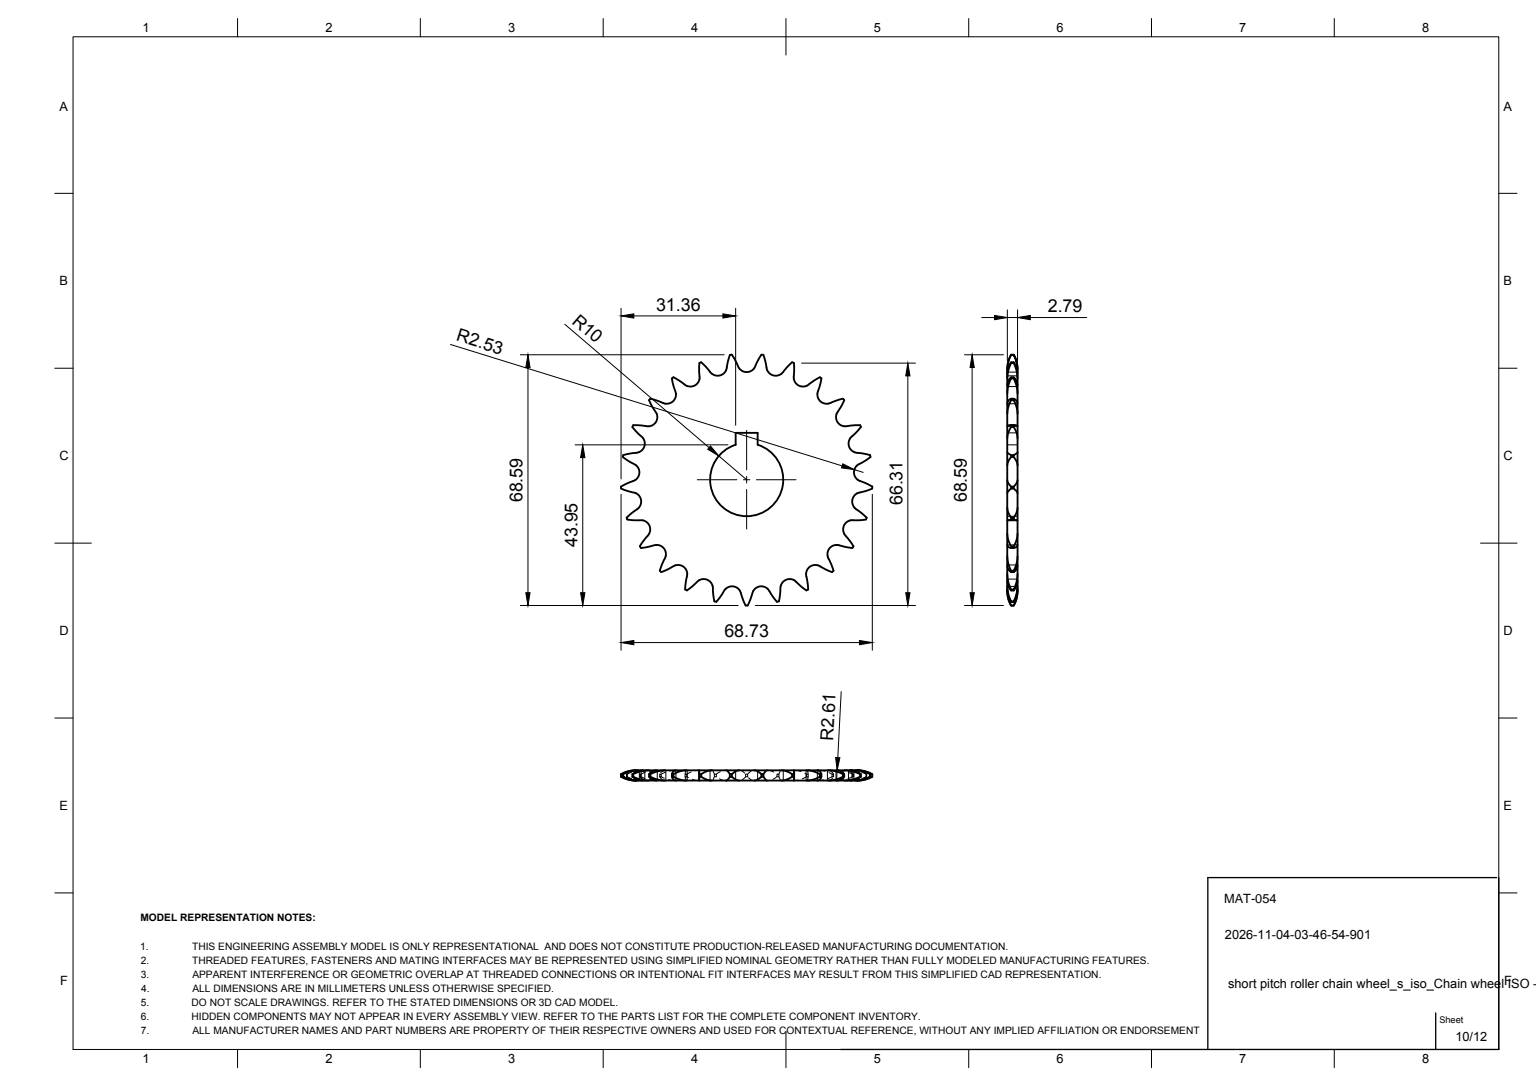
ISO-10303-21;
HEADER;
FILE_DESCRIPTION (('STEP AP214'),
    '1' );
FILE_NAME ('short pitch roller chain wheel_s_iso_Chain wheel ISO - 25Z 05B-1 --25SA20.0S1.step',
    '2026-10-21T17:50:41',
    ( '' ),
    ( '' ),
    'SwSTEP 2.0',
    'SolidWorks 2026',
    '' );
FILE_SCHEMA (( 'AUTOMOTIVE_DESIGN' ));
ENDSEC;

DATA;
#9=CARTESIAN_POINT ( 'NONE',  ( 0.000000000000000000, -17.83604598421681331, 24.70480026434162113 ) ) ;
#11=CARTESIAN_POINT ( 'NONE',  ( 2.789999999999999147, -7.666252171205286459, -29.49034198003814566 ) ) ;
#12=ADVANCED_FACE ( 'NONE', ( #16842 ), #19853, .T. ) ;
#15=ORIENTED_EDGE ( 'NONE', *, *, #1082, .T. ) ;
#18=DIRECTION ( 'NONE',  ( -1.000000000000000000, -0.000000000000000000, -0.000000000000000000 ) ) ;
#20=EDGE_LOOP ( 'NONE', ( #54, #27423, #18321, #7945 ) ) ;
#27=EDGE_LOOP ( 'NONE', ( #3921, #9561, #6087, #4128, #28214, #30495, #16586, #17626 ) ) ;
#41=DIRECTION ( 'NONE',  ( -1.000000000000000000, -0.000000000000000000, -0.000000000000000000 ) ) ;
#48=CARTESIAN_POINT ( 'NONE',  ( 8.000000000000000000, 0.000000000000000000, 0.000000000000000000 ) ) ;
#50=DIRECTION ( 'NONE',  ( -1.000000000000000000, -0.000000000000000000, -0.000000000000000000 ) ) ;
#53=B_SPLINE_CURVE_WITH_KNOTS ( 'NONE', 3,
 ( #11296, #13610, #21443, #2909 ),
 .UNSPECIFIED., .F., .F.,
 ( 4, 4 ),
 ( 1.980634265047841514E-07, 0.0006879337600918932361 ),
 .UNSPECIFIED. ) ;
#54=ORIENTED_EDGE ( 'NONE', *, *, #21337, .T. ) ;
#56=CARTESIAN_POINT ( 'NONE',  ( 2.789999999999999147, -23.41952779159776199, 19.49300927180536291 ) ) ;
#64=AXIS2_PLACEMENT_3D ( 'NONE', #13573, #18917, #21744 ) ;
#71=DIRECTION ( 'NONE',  ( 0.000000000000000000, -6.870191984066554061E-16, -1.000000000000000000 ) ) ;
#72=EDGE_LOOP ( 'NONE', ( #10606, #16036, #12165, #7623, #9118, #25813 ) ) ;
#78=ORIENTED_EDGE ( 'NONE', *, *, #19900, .T. ) ;
#82=ORIENTED_EDGE ( 'NONE', *, *, #22501, .F. ) ;
#89=FACE_OUTER_BOUND ( 'NONE', #8391, .T. ) ;
#102=AXIS2_PLACEMENT_3D ( 'NONE', #15826, #31812, #4404 ) ;
#107=CARTESIAN_POINT ( 'NONE',  ( 0.000000000000000000, -29.91351748324107973, 5.799410679710550021 ) ) ;
#112=ADVANCED_FACE ( 'NONE', ( #7166 ), #34411, .T. ) ;
#113=DIRECTION ( 'NONE',  ( 0.000000000000000000, 1.717547996016640980E-15, -1.000000000000000000 ) ) ;
#115=CARTESIAN_POINT ( 'NONE',  ( 1.749999999999999778, -10.89151784028265624, -32.64600270996228204 ) ) ;
#117=ORIENTED_EDGE ( 'NONE', *, *, #2620, .T. ) ;
#131=CARTESIAN_POINT ( 'NONE',  ( 1.039999999999999591, -18.21166265554809627, 29.20140402659733425 ) ) ;
#147=B_SPLINE_CURVE_WITH_KNOTS ( 'NONE', 3,
 ( #10015, #12703, #20870, #26557, #32247, #23363 ),
 .UNSPECIFIED., .F., .F.,
 ( 4, 2, 4 ),
 ( 2.446897702420577325E-07, 0.001873443032870420388, 0.003746641375970598611 ),
 .UNSPECIFIED. ) ;
#152=B_SPLINE_CURVE_WITH_KNOTS ( 'NONE', 3,
 ( #1584, #18327, #31299, #33977, #2108, #6909 ),
 .UNSPECIFIED., .F., .F.,
 ( 4, 2, 4 ),
 ( 4.404817104455272006E-07, 0.001874269680285309877, 0.003748098878860173927 ),
 .UNSPECIFIED. ) ;
#154=AXIS2_PLACEMENT_3D ( 'NONE', #33975, #1065, #20629 ) ;
#159=ORIENTED_EDGE ( 'NONE', *, *, #4581, .F. ) ;
#163=EDGE_CURVE ( 'NONE', #29138, #16548, #8258, .T. ) ;
#164=DIRECTION ( 'NONE',  ( -1.000000000000000000, -0.000000000000000000, -0.000000000000000000 ) ) ;
#176=DIRECTION ( 'NONE',  ( 0.000000000000000000, 0.000000000000000000, 1.000000000000000000 ) ) ;
#183=CARTESIAN_POINT ( 'NONE',  ( 1.749999999999999778, 32.09669216789253454, -12.41728656686340138 ) ) ;
#184=DIRECTION ( 'NONE',  ( 0.000000000000000000, 0.000000000000000000, 1.000000000000000000 ) ) ;
#188=TOROIDAL_SURFACE ( 'NONE', #34853, 30.47050528711512030, 8.000000000000000000 ) ;
#190=LINE ( 'NONE', #16406, #20541 ) ;
#191=CARTESIAN_POINT ( 'NONE',  ( 2.789999999999999147, -1.291199951812987523, -30.41225463960053332 ) ) ;
#205=TOROIDAL_SURFACE ( 'NONE', #2485, 30.47050528711512030, 8.000000000000000000 ) ;
#206=ORIENTED_EDGE ( 'NONE', *, *, #33017, .T. ) ;
#207=ORIENTED_EDGE ( 'NONE', *, *, #14796, .T. ) ;
#218=CARTESIAN_POINT ( 'NONE',  ( 1.749999999999999778, -33.26546734453825849, 8.820166447041632551 ) ) ;
#220=CARTESIAN_POINT ( 'NONE',  ( 0.5248942730704680981, -11.05013152551600442, -31.49770363594219091 ) ) ;
#227=CARTESIAN_POINT ( 'NONE',  ( -8.297462993384987146E-14, 27.83741677616693266, 12.85620214406761086 ) ) ;
#245=VERTEX_POINT ( 'NONE', #5376 ) ;
#256=VECTOR ( 'NONE', #18006, 1000.000000000000000 ) ;
#258=CARTESIAN_POINT ( 'NONE',  ( 2.789999999999999147, -25.83993731729808729, 18.77381338200959604 ) ) ;
#263=AXIS2_PLACEMENT_3D ( 'NONE', #22124, #50, #11096 ) ;
#267=CARTESIAN_POINT ( 'NONE',  ( 0.000000000000000000, -7.666252171205264254, -29.49034198003815632 ) ) ;
#272=ORIENTED_EDGE ( 'NONE', *, *, #3278, .F. ) ;
#278=ADVANCED_FACE ( 'NONE', ( #16441 ), #5428, .T. ) ;
#289=ORIENTED_EDGE ( 'NONE', *, *, #26141, .T. ) ;
#292=VERTEX_POINT ( 'NONE', #13238 ) ;
#293=ORIENTED_EDGE ( 'NONE', *, *, #23924, .F. ) ;
#294=CARTESIAN_POINT ( 'NONE',  ( -10.00000000000000000, 0.000000000000000000, 0.000000000000000000 ) ) ;
#301=CARTESIAN_POINT ( 'NONE',  ( 2.033589663487044952, 13.95893286369055097, -30.90974742850055179 ) ) ;
#312=CARTESIAN_POINT ( 'NONE',  ( 2.789999999999999147, 7.350529080603967813, -30.20932655202929595 ) ) ;
#320=CARTESIAN_POINT ( 'NONE',  ( 1.749999999999999778, 0.000000000000000000, 0.000000000000000000 ) ) ;
#326=ORIENTED_EDGE ( 'NONE', *, *, #11265, .T. ) ;
#328=CARTESIAN_POINT ( 'NONE',  ( 2.789999999999999147, 0.000000000000000000, 0.000000000000000000 ) ) ;
#343=ORIENTED_EDGE ( 'NONE', *, *, #19695, .F. ) ;
#349=CARTESIAN_POINT ( 'NONE',  ( 0.000000000000000000, -30.41598411195408502, -1.821977758773957179 ) ) ;
#364=VECTOR ( 'NONE', #34672, 1000.000000000000000 ) ;
#391=CARTESIAN_POINT ( 'NONE',  ( 2.261199744108339349, -18.53787122671715082, -27.77096539590149504 ) ) ;
#400=ORIENTED_EDGE ( 'NONE', *, *, #18488, .T. ) ;
#401=DIRECTION ( 'NONE',  ( 0.000000000000000000, -4.122115190439938353E-15, -1.000000000000000000 ) ) ;
#403=DIRECTION ( 'NONE',  ( 0.000000000000000000, 0.000000000000000000, 1.000000000000000000 ) ) ;
#405=CARTESIAN_POINT ( 'NONE',  ( 2.789999999999999147, -2.530647759431309929, -30.33427519320597199 ) ) ;
#408=FACE_OUTER_BOUND ( 'NONE', #18168, .T. ) ;
#416=ORIENTED_EDGE ( 'NONE', *, *, #6218, .F. ) ;
#422=DIRECTION ( 'NONE',  ( -1.000000000000000000, -0.000000000000000000, -0.000000000000000000 ) ) ;
#432=ORIENTED_EDGE ( 'NONE', *, *, #20397, .F. ) ;
#447=CARTESIAN_POINT ( 'NONE',  ( 0.006892415499590480790, 4.187058600949983500, -30.58452291340886831 ) ) ;
#448=CARTESIAN_POINT ( 'NONE',  ( 2.719010669804482916, -30.32061017160040350, -9.230676164042293408 ) ) ;
#453=ORIENTED_EDGE ( 'NONE', *, *, #7812, .T. ) ;
#455=CIRCLE ( 'NONE', #12411, 2.524999999999999467 ) ;
#462=EDGE_LOOP ( 'NONE', ( #2821, #4541, #31445, #15602, #5501, #28046 ) ) ;
#471=CARTESIAN_POINT ( 'NONE',  ( 2.783107615394383672, -17.88431215799149143, 25.16139613958896604 ) ) ;
#483=CARTESIAN_POINT ( 'NONE',  ( 0.7564103440795023614, 14.91861104533797899, -30.45815716957487496 ) ) ;
#485=DIRECTION ( 'NONE',  ( -1.000000000000000000, 0.000000000000000000, -0.000000000000000000 ) ) ;
#487=ORIENTED_EDGE ( 'NONE', *, *, #9637, .F. ) ;
#491=CIRCLE ( 'NONE', #22653, 2.524999999999999467 ) ;
#492=DIRECTION ( 'NONE',  ( -1.000000000000000000, -0.000000000000000000, -0.000000000000000000 ) ) ;
#500=TOROIDAL_SURFACE ( 'NONE', #9599, 30.47050528711512030, 8.000000000000000000 ) ;
#507=CARTESIAN_POINT ( 'NONE',  ( 0.5248942543850775300, -33.37077467988373769, 0.7759739055973007282 ) ) ;
#509=VERTEX_POINT ( 'NONE', #1793 ) ;
#513=CARTESIAN_POINT ( 'NONE',  ( 2.719010673315533477, 14.74869129583236216, -28.05389252521634802 ) ) ;
#517=ORIENTED_EDGE ( 'NONE', *, *, #32290, .F. ) ;
#527=VERTEX_POINT ( 'NONE', #12669 ) ;
#528=LINE ( 'NONE', #11379, #25963 ) ;
#536=DIRECTION ( 'NONE',  ( 1.000000000000000000, -0.000000000000000000, -0.000000000000000000 ) ) ;
#537=ORIENTED_EDGE ( 'NONE', *, *, #19901, .F. ) ;
#543=LINE ( 'NONE', #35085, #19991 ) ;
#550=DIRECTION ( 'NONE',  ( -1.000000000000000000, 0.000000000000000000, 0.000000000000000000 ) ) ;
#559=EDGE_CURVE ( 'NONE', #10218, #5077, #21246, .T. ) ;
#570=CARTESIAN_POINT ( 'NONE',  ( 0.000000000000000000, -20.35927063852824048, 24.61013060777164796 ) ) ;
#583=DIRECTION ( 'NONE',  ( -1.000000000000000000, -0.000000000000000000, -0.000000000000000000 ) ) ;
#589=CARTESIAN_POINT ( 'NONE',  ( 2.789999999999999591, -3.625355760179855835, 30.44651458975030067 ) ) ;
#595=CARTESIAN_POINT ( 'NONE',  ( 0.000000000000000000, -25.77598557799239742, -16.24962337825829195 ) ) ;
#597=ORIENTED_EDGE ( 'NONE', *, *, #21069, .F. ) ;
#602=ADVANCED_FACE ( 'NONE', ( #4451 ), #23172, .T. ) ;
#605=CARTESIAN_POINT ( 'NONE',  ( 2.261199747851626807, 5.497007441955480189, -32.93420861807575051 ) ) ;
#612=CARTESIAN_POINT ( 'NONE',  ( 1.040000000000003810, -2.430610048905784915, -34.32897884578301984 ) ) ;
#615=CARTESIAN_POINT ( 'NONE',  ( 1.040000000000000258, 28.00026196654270905, 20.00929742917132614 ) ) ;
#617=CARTESIAN_POINT ( 'NONE',  ( 0.02407890056655825201, -23.70329957282570632, -20.11932597908854703 ) ) ;
#622=( GEOMETRIC_REPRESENTATION_CONTEXT ( 3 ) GLOBAL_UNCERTAINTY_ASSIGNED_CONTEXT ( ( #6076 ) ) GLOBAL_UNIT_ASSIGNED_CONTEXT ( ( #14562, #33576, #1191 ) ) REPRESENTATION_CONTEXT ( 'NONE', 'WORKASPACE' ) );
#625=DIRECTION ( 'NONE',  ( -1.000000000000000000, -0.000000000000000000, -0.000000000000000000 ) ) ;
#628=CYLINDRICAL_SURFACE ( 'NONE', #33668, 34.41491905851385269 ) ;
#637=DIRECTION ( 'NONE',  ( -1.000000000000000000, -0.000000000000000000, -0.000000000000000000 ) ) ;
#638=CARTESIAN_POINT ( 'NONE',  ( 2.789999999999999147, -21.75986515490462736, -21.28569233123117144 ) ) ;
#642=FACE_OUTER_BOUND ( 'NONE', #3782, .T. ) ;
#644=AXIS2_PLACEMENT_3D ( 'NONE', #32551, #30604, #176 ) ;
#645=CARTESIAN_POINT ( 'NONE',  ( -4.087654984470516816E-16, 27.73515059361837842, -12.87176213890998433 ) ) ;
#655=LINE ( 'NONE', #13651, #10552 ) ;
#671=AXIS2_PLACEMENT_3D ( 'NONE', #19191, #13656, #30199 ) ;
#674=CARTESIAN_POINT ( 'NONE',  ( 1.749999999999999778, 14.89726405156217126, 31.02351007835983054 ) ) ;
#681=EDGE_CURVE ( 'NONE', #1567, #23446, #30476, .T. ) ;
#684=DIRECTION ( 'NONE',  ( -1.000000000000000000, -0.000000000000000000, -0.000000000000000000 ) ) ;
#686=CARTESIAN_POINT ( 'NONE',  ( 0.02407890056655695096, -23.70329957282599764, 20.11932597908820242 ) ) ;
#689=LINE ( 'NONE', #22397, #22097 ) ;
#693=VERTEX_POINT ( 'NONE', #5676 ) ;
#698=CARTESIAN_POINT ( 'NONE',  ( 2.765921099433441999, -23.70329957282570632, -20.11932597908854703 ) ) ;
#701=VERTEX_POINT ( 'NONE', #5505 ) ;
#706=CARTESIAN_POINT ( 'NONE',  ( 0.02407890056655868569, 24.20451283648829133, 19.51346322004938827 ) ) ;
#713=FACE_OUTER_BOUND ( 'NONE', #31703, .T. ) ;
#719=EDGE_CURVE ( 'NONE', #25735, #29292, #10014, .T. ) ;
#723=VECTOR ( 'NONE', #4056, 1000.000000000000000 ) ;
#758=ORIENTED_EDGE ( 'NONE', *, *, #30163, .F. ) ;
#762=EDGE_CURVE ( 'NONE', #30403, #3499, #15137, .T. ) ;
#765=ORIENTED_EDGE ( 'NONE', *, *, #6752, .T. ) ;
#767=AXIS2_PLACEMENT_3D ( 'NONE', #17195, #9516, #17375 ) ;
#784=ORIENTED_EDGE ( 'NONE', *, *, #22789, .T. ) ;
#795=AXIS2_PLACEMENT_3D ( 'NONE', #25885, #23221, #30872 ) ;
#797=VERTEX_POINT ( 'NONE', #7654 ) ;
#798=DIRECTION ( 'NONE',  ( 0.000000000000000000, 0.000000000000000000, 1.000000000000000000 ) ) ;
#812=ORIENTED_EDGE ( 'NONE', *, *, #27179, .F. ) ;
#814=B_SPLINE_CURVE_WITH_KNOTS ( 'NONE', 3,
 ( #14475, #31011, #28163, #940, #14997, #1459 ),
 .UNSPECIFIED., .F., .F.,
 ( 4, 2, 4 ),
 ( 2.343813143889068798E-07, 0.001873432713173589807, 0.003746631045032783325 ),
 .UNSPECIFIED. ) ;
#816=CIRCLE ( 'NONE', #30389, 30.47050528711512030 ) ;
#818=CARTESIAN_POINT ( 'NONE',  ( 0.000000000000000000, 0.000000000000000000, 0.000000000000000000 ) ) ;
#822=CARTESIAN_POINT ( 'NONE',  ( 0.07098932849787087385, 31.23843357299762857, -5.357709411917221054 ) ) ;
#824=ORIENTED_EDGE ( 'NONE', *, *, #23128, .F. ) ;
#830=DIRECTION ( 'NONE',  ( 0.000000000000000000, 0.000000000000000000, 1.000000000000000000 ) ) ;
#831=CARTESIAN_POINT ( 'NONE',  ( 0.000000000000000000, -5.984944020946091570, 31.37417528048439763 ) ) ;
#833=CARTESIAN_POINT ( 'NONE',  ( 1.394999999999999574, 6.714005886385425725, -33.75364837705166110 ) ) ;
#839=AXIS2_PLACEMENT_3D ( 'NONE', #13257, #7899, #20906 ) ;
#840=B_SPLINE_CURVE_WITH_KNOTS ( 'NONE', 3,
 ( #9936, #25292, #8926, #10109, #6597, #26129 ),
 .UNSPECIFIED., .F., .F.,
 ( 4, 2, 4 ),
 ( 4.404817133574835894E-07, 0.001874269703891905288, 0.003748098926070445643 ),
 .UNSPECIFIED. ) ;
#845=AXIS2_PLACEMENT_3D ( 'NONE', #22762, #9054, #27387 ) ;
#850=AXIS2_PLACEMENT_3D ( 'NONE', #14253, #6390, #19596 ) ;
#853=LINE ( 'NONE', #6703, #25713 ) ;
#856=ORIENTED_EDGE ( 'NONE', *, *, #12997, .T. ) ;
#876=ORIENTED_EDGE ( 'NONE', *, *, #5437, .T. ) ;
#886=ORIENTED_EDGE ( 'NONE', *, *, #32162, .T. ) ;
#908=CARTESIAN_POINT ( 'NONE',  ( 8.000000000000000000, 0.000000000000000000, 0.000000000000000000 ) ) ;
#915=DIRECTION ( 'NONE',  ( -1.000000000000000000, -0.000000000000000000, -0.000000000000000000 ) ) ;
#916=VERTEX_POINT ( 'NONE', #17758 ) ;
#919=AXIS2_PLACEMENT_3D ( 'NONE', #30994, #17497, #28147 ) ;
#925=CARTESIAN_POINT ( 'NONE',  ( 0.07094833174329351344, -22.12275578582332258, -22.69570394412150094 ) ) ;
#926=EDGE_CURVE ( 'NONE', #18645, #8559, #4534, .T. ) ;
#930=DIRECTION ( 'NONE',  ( -1.000000000000000000, -0.000000000000000000, 0.000000000000000000 ) ) ;
#933=CARTESIAN_POINT ( 'NONE',  ( 0.000000000000000000, 0.000000000000000000, 0.000000000000000000 ) ) ;
#938=CARTESIAN_POINT ( 'NONE',  ( 0.07098930208213954929, -22.12324074713423983, 22.69596835361121379 ) ) ;
#939=VERTEX_POINT ( 'NONE', #24113 ) ;
#940=CARTESIAN_POINT ( 'NONE',  ( 2.265105836449367249, -9.574141296992072725, -31.97728166840280295 ) ) ;
#947=EDGE_LOOP ( 'NONE', ( #30573, #9309, #21201, #23371 ) ) ;
#949=VERTEX_POINT ( 'NONE', #26096 ) ;
#956=CARTESIAN_POINT ( 'NONE',  ( 1.749999999999999778, 0.000000000000000000, 0.000000000000000000 ) ) ;
#965=DIRECTION ( 'NONE',  ( -1.000000000000000000, -0.000000000000000000, 0.000000000000000000 ) ) ;
#968=EDGE_CURVE ( 'NONE', #34921, #949, #21287, .T. ) ;
#992=ORIENTED_EDGE ( 'NONE', *, *, #23128, .T. ) ;
#1002=ORIENTED_EDGE ( 'NONE', *, *, #10125, .T. ) ;
#1008=CARTESIAN_POINT ( 'NONE',  ( 1.040000000000000924, -18.66807150955393624, -28.91175816027522316 ) ) ;
#1011=EDGE_CURVE ( 'NONE', #29748, #30400, #2067, .T. ) ;
#1013=DIRECTION ( 'NONE',  ( -1.000000000000000000, 0.000000000000000000, 0.000000000000000000 ) ) ;
#1023=ORIENTED_EDGE ( 'NONE', *, *, #17027, .T. ) ;
#1026=CIRCLE ( 'NONE', #29448, 2.525000000000000799 ) ;
#1033=CYLINDRICAL_SURFACE ( 'NONE', #4520, 16.19999999999999929 ) ;
#1048=B_SPLINE_CURVE_WITH_KNOTS ( 'NONE', 3,
 ( #12793, #34310, #605, #32333, #16164, #22322 ),
 .UNSPECIFIED., .F., .F.,
 ( 4, 2, 4 ),
 ( 4.404817060652725496E-07, 0.001874269649560036423, 0.003748098817414007630 ),
 .UNSPECIFIED. ) ;
#1049=CARTESIAN_POINT ( 'NONE',  ( 1.040000000000001146, 21.72796464722008025, 26.68861566460903134 ) ) ;
#1051=ORIENTED_EDGE ( 'NONE', *, *, #3243, .F. ) ;
#1052=CARTESIAN_POINT ( 'NONE',  ( 2.606461907020827251, -31.53621309121735194, 6.848028948309839770 ) ) ;
#1057=ADVANCED_FACE ( 'NONE', ( #28943 ), #34459, .F. ) ;
#1060=ORIENTED_EDGE ( 'NONE', *, *, #27470, .F. ) ;
#1065=DIRECTION ( 'NONE',  ( -1.000000000000000000, -0.000000000000000000, -0.000000000000000000 ) ) ;
#1078=EDGE_LOOP ( 'NONE', ( #8545, #2209, #34917, #26406 ) ) ;
#1080=EDGE_CURVE ( 'NONE', #5077, #15056, #15786, .T. ) ;
#1082=EDGE_CURVE ( 'NONE', #13600, #23413, #21990, .T. ) ;
#1088=CARTESIAN_POINT ( 'NONE',  ( 2.719010679974587230, -18.14847849655048506, 25.98417794693611782 ) ) ;
#1093=CARTESIAN_POINT ( 'NONE',  ( 1.749999999999999778, 34.10861917999622506, -4.581348211831717698 ) ) ;
#1099=EDGE_CURVE ( 'NONE', #12821, #24367, #15334, .T. ) ;
#1100=EDGE_CURVE ( 'NONE', #17221, #31475, #28500, .T. ) ;
#1106=CARTESIAN_POINT ( 'NONE',  ( 2.265105730852140287, 33.01038087096667084, 4.952322205615443451 ) ) ;
#1112=FACE_OUTER_BOUND ( 'NONE', #12815, .T. ) ;
#1122=ORIENTED_EDGE ( 'NONE', *, *, #12067, .F. ) ;
#1127=EDGE_CURVE ( 'NONE', #13812, #701, #14617, .T. ) ;
#1135=DIRECTION ( 'NONE',  ( -1.000000000000000000, -0.000000000000000000, -0.000000000000000000 ) ) ;
#1139=FACE_OUTER_BOUND ( 'NONE', #18911, .T. ) ;
#1150=AXIS2_PLACEMENT_3D ( 'NONE', #6582, #33640, #25277 ) ;
#1159=CARTESIAN_POINT ( 'NONE',  ( 2.765921099433444219, 31.00221527374952046, 2.344426712874309260 ) ) ;
#1166=ORIENTED_EDGE ( 'NONE', *, *, #4549, .T. ) ;
#1173=ORIENTED_EDGE ( 'NONE', *, *, #31545, .T. ) ;
#1176=DIRECTION ( 'NONE',  ( 1.000000000000000000, -0.000000000000000000, -0.000000000000000000 ) ) ;
#1183=AXIS2_PLACEMENT_3D ( 'NONE', #16487, #14473, #30162 ) ;
#1185=CARTESIAN_POINT ( 'NONE',  ( 1.040000000000000036, 31.89769921723006263, -12.91988538846923973 ) ) ;
#1187=ORIENTED_EDGE ( 'NONE', *, *, #14083, .F. ) ;
#1191=( NAMED_UNIT ( * ) SI_UNIT ( $, .STERADIAN. ) SOLID_ANGLE_UNIT ( ) );
#1195=SHAPE_REPRESENTATION ( 'short pitch roller chain wheel_s_iso_Chain wheel ISO - 25Z 05B-1 --25SA20.0S1', ( #28566 ), #10954 ) ;
#1205=AXIS2_PLACEMENT_3D ( 'NONE', #9898, #1882, #15429 ) ;
#1206=CARTESIAN_POINT ( 'NONE',  ( 2.789999999999999147, -29.91351748324099091, -5.799410679710938155 ) ) ;
#1207=ADVANCED_FACE ( 'NONE', ( #28028 ), #11195, .T. ) ;
#1215=ORIENTED_EDGE ( 'NONE', *, *, #12710, .T. ) ;
#1219=AXIS2_PLACEMENT_3D ( 'NONE', #14763, #14936, #23289 ) ;
#1222=CARTESIAN_POINT ( 'NONE',  ( 2.789999999999999147, 11.49079834592189897, 28.42701364291173149 ) ) ;
#1224=CARTESIAN_POINT ( 'NONE',  ( 0.000000000000000000, 1.224646799147353256E-15, -10.00000000000000000 ) ) ;
#1226=VERTEX_POINT ( 'NONE', #12375 ) ;
#1231=CARTESIAN_POINT ( 'NONE',  ( 1.749999999999999778, -18.21166265554766994, -29.20140402659760070 ) ) ;
#1236=AXIS2_PLACEMENT_3D ( 'NONE', #2308, #29726, #32744 ) ;
#1250=EDGE_CURVE ( 'NONE', #2295, #22708, #31023, .T. ) ;
#1251=CARTESIAN_POINT ( 'NONE',  ( 2.033800793502754445, 13.95859842408627038, 30.90949138205576219 ) ) ;
#1253=EDGE_CURVE ( 'NONE', #22184, #6749, #4918, .T. ) ;
#1254=DIRECTION ( 'NONE',  ( -1.000000000000000000, -0.000000000000000000, -0.000000000000000000 ) ) ;
#1277=CARTESIAN_POINT ( 'NONE',  ( 0.5248942285756895698, 33.20489141755878393, 3.412611943275336124 ) ) ;
#1281=AXIS2_PLACEMENT_3D ( 'NONE', #20582, #12757, #15597 ) ;
#1284=CYLINDRICAL_SURFACE ( 'NONE', #1183, 2.524999999999999467 ) ;
#1286=B_SPLINE_CURVE_WITH_KNOTS ( 'NONE', 3,
 ( #7807, #32013, #34519, #18000 ),
 .UNSPECIFIED., .F., .F.,
 ( 4, 4 ),
 ( 0.005298345749243330016, 0.005985214453301815341 ),
 .UNSPECIFIED. ) ;
#1293=FACE_OUTER_BOUND ( 'NONE', #25940, .T. ) ;
#1294=EDGE_CURVE ( 'NONE', #23520, #30318, #7681, .T. ) ;
#1297=ORIENTED_EDGE ( 'NONE', *, *, #33193, .F. ) ;
#1302=CARTESIAN_POINT ( 'NONE',  ( 2.789999999999999147, -23.41952779159776199, 19.49300927180536291 ) ) ;
#1305=VERTEX_POINT ( 'NONE', #14347 ) ;
#1307=EDGE_LOOP ( 'NONE', ( #15407, #21157, #27983, #5723, #28927, #18871 ) ) ;
#1313=EDGE_CURVE ( 'NONE', #292, #9463, #11107, .T. ) ;
#1333=CARTESIAN_POINT ( 'NONE',  ( 0.000000000000000000, -20.35927063852789232, -24.61013060777193218 ) ) ;
#1336=AXIS2_PLACEMENT_3D ( 'NONE', #1879, #2063, #34282 ) ;
#1341=B_SPLINE_CURVE_WITH_KNOTS ( 'NONE', 3,
 ( #18800, #8455, #21987, #19157 ),
 .UNSPECIFIED., .F., .F.,
 ( 4, 4 ),
 ( 0.005298347253562356134, 0.005985215922708608631 ),
 .UNSPECIFIED. ) ;
#1348=CARTESIAN_POINT ( 'NONE',  ( 0.02407890056655738464, -11.07880054387241664, 29.04985141099759360 ) ) ;
#1351=CARTESIAN_POINT ( 'NONE',  ( 0.000000000000000000, 0.000000000000000000, 0.000000000000000000 ) ) ;
#1352=ORIENTED_EDGE ( 'NONE', *, *, #31784, .F. ) ;
#1362=VECTOR ( 'NONE', #25435, 1000.000000000000000 ) ;
#1364=VERTEX_POINT ( 'NONE', #34776 ) ;
#1366=CARTESIAN_POINT ( 'NONE',  ( 2.783107601403548959, -11.06505884892056102, 28.81855237217592958 ) ) ;
#1371=CARTESIAN_POINT ( 'NONE',  ( 2.789999999999999147, 0.000000000000000000, 0.000000000000000000 ) ) ;
#1380=ORIENTED_EDGE ( 'NONE', *, *, #5701, .T. ) ;
#1384=ORIENTED_EDGE ( 'NONE', *, *, #16115, .T. ) ;
#1389=CARTESIAN_POINT ( 'NONE',  ( 2.789999999999999147, 30.11551674275779433, 4.430359003076457469 ) ) ;
#1391=ORIENTED_EDGE ( 'NONE', *, *, #25706, .F. ) ;
#1395=CARTESIAN_POINT ( 'NONE',  ( 2.783128933731652488, 23.98851302352063897, -19.42881381898143545 ) ) ;
#1401=ORIENTED_EDGE ( 'NONE', *, *, #25136, .T. ) ;
#1404=CARTESIAN_POINT ( 'NONE',  ( 0.5288002438369178160, 20.68324032934645018, 26.21226347405753998 ) ) ;
#1408=EDGE_CURVE ( 'NONE', #14065, #34278, #9467, .T. ) ;
#1409=AXIS2_PLACEMENT_3D ( 'NONE', #21590, #27624, #30295 ) ;
#1412=ORIENTED_EDGE ( 'NONE', *, *, #19543, .F. ) ;
#1459=CARTESIAN_POINT ( 'NONE',  ( 1.749999999999999778, -10.37741591188871482, -32.81304455236878681 ) ) ;
#1466=CIRCLE ( 'NONE', #5996, 34.41491905851385269 ) ;
#1467=CARTESIAN_POINT ( 'NONE',  ( 0.006871098824289784829, 18.40312061469623472, 24.78412275958840283 ) ) ;
#1468=ORIENTED_EDGE ( 'NONE', *, *, #27241, .T. ) ;
#1476=DIRECTION ( 'NONE',  ( -1.000000000000000000, -0.000000000000000000, -0.000000000000000000 ) ) ;
#1477=ORIENTED_EDGE ( 'NONE', *, *, #32189, .F. ) ;
#1481=LINE ( 'NONE', #23362, #3323 ) ;
#1490=CARTESIAN_POINT ( 'NONE',  ( 1.749999999999999778, 14.89726405156260469, -31.02351007835961383 ) ) ;
#1502=ORIENTED_EDGE ( 'NONE', *, *, #9274, .F. ) ;
#1510=EDGE_CURVE ( 'NONE', #24976, #16592, #18747, .T. ) ;
#1511=B_SPLINE_CURVE_WITH_KNOTS ( 'NONE', 3,
 ( #13514, #35058, #32364, #29704 ),
 .UNSPECIFIED., .F., .F.,
 ( 4, 4 ),
 ( 0.0006242955995025980349, 0.0006879396046782833979 ),
 .UNSPECIFIED. ) ;
#1515=ORIENTED_EDGE ( 'NONE', *, *, #30287, .F. ) ;
#1519=CARTESIAN_POINT ( 'NONE',  ( 0.5288002590931849545, -11.04911166161968161, 31.50867056184614867 ) ) ;
#1522=B_SPLINE_CURVE_WITH_KNOTS ( 'NONE', 3,
 ( #218, #30393, #18920, #10736, #5365, #5537 ),
 .UNSPECIFIED., .F., .F.,
 ( 4, 2, 4 ),
 ( 4.404817001457452636E-07, 0.001874269605587669443, 0.003748098729475193413 ),
 .UNSPECIFIED. ) ;
#1537=CARTESIAN_POINT ( 'NONE',  ( 8.768203845046324740E-16, -14.96303950468941402, 26.76267923429985629 ) ) ;
#1540=ORIENTED_EDGE ( 'NONE', *, *, #30668, .F. ) ;
#1544=ORIENTED_EDGE ( 'NONE', *, *, #30501, .F. ) ;
#1548=AXIS2_PLACEMENT_3D ( 'NONE', #5309, #19047, #32723 ) ;
#1564=DIRECTION ( 'NONE',  ( 0.000000000000000000, 0.000000000000000000, 1.000000000000000000 ) ) ;
#1567=VERTEX_POINT ( 'NONE', #17212 ) ;
#1573=TOROIDAL_SURFACE ( 'NONE', #14654, 30.47050528711512030, 8.000000000000000000 ) ;
#1581=EDGE_LOOP ( 'NONE', ( #13449, #1380, #34172, #23284 ) ) ;
#1582=CARTESIAN_POINT ( 'NONE',  ( 1.394999999999999574, -18.66807150955433769, 28.91175816027496381 ) ) ;
#1584=CARTESIAN_POINT ( 'NONE',  ( 1.749999999999999778, -25.27164158951550732, -23.36088151536945645 ) ) ;
#1603=ORIENTED_EDGE ( 'NONE', *, *, #13178, .F. ) ;
#1604=DIRECTION ( 'NONE',  ( -1.000000000000000000, -0.000000000000000000, -0.000000000000000000 ) ) ;
#1613=VERTEX_POINT ( 'NONE', #10394 ) ;
#1617=VERTEX_POINT ( 'NONE', #31408 ) ;
#1624=CARTESIAN_POINT ( 'NONE',  ( 0.000000000000000000, 0.000000000000000000, -3.000000000000000000 ) ) ;
#1626=CARTESIAN_POINT ( 'NONE',  ( 0.01642902444827818234, 28.19451832957808435, -12.86842533592864868 ) ) ;
#1628=AXIS2_PLACEMENT_3D ( 'NONE', #14190, #24007, #830 ) ;
#1629=ORIENTED_EDGE ( 'NONE', *, *, #19026, .F. ) ;
#1630=( NAMED_UNIT ( * ) SI_UNIT ( $, .STERADIAN. ) SOLID_ANGLE_UNIT ( ) );
#1633=ADVANCED_FACE ( 'NONE', ( #34077 ), #26587, .T. ) ;
#1636=DIRECTION ( 'NONE',  ( 0.000000000000000000, 0.000000000000000000, 1.000000000000000000 ) ) ;
#1637=ORIENTED_EDGE ( 'NONE', *, *, #15211, .T. ) ;
#1638=ORIENTED_EDGE ( 'NONE', *, *, #5076, .T. ) ;
#1640=EDGE_CURVE ( 'NONE', #21299, #6869, #11120, .T. ) ;
#1641=CYLINDRICAL_SURFACE ( 'NONE', #33225, 34.41491905851385269 ) ;
#1651=EDGE_CURVE ( 'NONE', #12523, #25735, #8256, .T. ) ;
#1656=DIRECTION ( 'NONE',  ( 0.000000000000000000, 0.000000000000000000, 1.000000000000000000 ) ) ;
#1659=CARTESIAN_POINT ( 'NONE',  ( 2.789999999999999147, -29.32277567846606203, 8.169899392882690847 ) ) ;
#1667=VECTOR ( 'NONE', #14363, 1000.000000000000000 ) ;
#1669=ORIENTED_EDGE ( 'NONE', *, *, #20197, .F. ) ;
#1671=CARTESIAN_POINT ( 'NONE',  ( 2.765921099433441999, 26.03801215795542134, -16.98986790278583570 ) ) ;
#1676=EDGE_LOOP ( 'NONE', ( #26031, #3781, #26289, #18122 ) ) ;
#1681=CARTESIAN_POINT ( 'NONE',  ( 2.789999999999999147, -20.35927063852789232, -24.61013060777193218 ) ) ;
#1686=EDGE_CURVE ( 'NONE', #14706, #14486, #11041, .T. ) ;
#1696=EDGE_CURVE ( 'NONE', #23220, #32336, #12547, .T. ) ;
#1700=VECTOR ( 'NONE', #12167, 1000.000000000000000 ) ;
#1702=CARTESIAN_POINT ( 'NONE',  ( 1.749999999999999778, -18.66807150955392913, -28.91175816027522671 ) ) ;
#1705=CARTESIAN_POINT ( 'NONE',  ( 0.7564103443181301456, 33.57753319639230227, 4.776354065835291429 ) ) ;
#1706=DIRECTION ( 'NONE',  ( -1.000000000000000000, -0.000000000000000000, -0.000000000000000000 ) ) ;
#1708=FACE_OUTER_BOUND ( 'NONE', #15646, .T. ) ;
#1710=B_SPLINE_CURVE_WITH_KNOTS ( 'NONE', 3,
 ( #22334, #12024, #8988, #8621, #30342, #32997 ),
 .UNSPECIFIED., .F., .F.,
 ( 4, 2, 4 ),
 ( 2.555309558411697678E-07, 0.001873453885876980246, 0.003746652240798119347 ),
 .UNSPECIFIED. ) ;
#1712=VERTEX_POINT ( 'NONE', #7183 ) ;
#1727=DIRECTION ( 'NONE',  ( 0.000000000000000000, 0.000000000000000000, 1.000000000000000000 ) ) ;
#1732=ORIENTED_EDGE ( 'NONE', *, *, #9450, .T. ) ;
#1744=CYLINDRICAL_SURFACE ( 'NONE', #33902, 16.19999999999999574 ) ;
#1749=EDGE_LOOP ( 'NONE', ( #32130, #272, #159, #32027 ) ) ;
#1766=AXIS2_PLACEMENT_3D ( 'NONE', #4866, #15764, #4174 ) ;
#1771=VERTEX_POINT ( 'NONE', #21603 ) ;
#1773=CARTESIAN_POINT ( 'NONE',  ( 2.765921099433442887, 24.20451283648829133, 19.51346322004938827 ) ) ;
#1782=FACE_OUTER_BOUND ( 'NONE', #3943, .T. ) ;
#1785=CARTESIAN_POINT ( 'NONE',  ( 2.789999999999999147, -20.92506858792740587, -22.14933852381698642 ) ) ;
#1790=DIRECTION ( 'NONE',  ( -1.000000000000000000, 0.000000000000000000, 0.000000000000000000 ) ) ;
#1792=CARTESIAN_POINT ( 'NONE',  ( 2.789999999999999147, -7.666252171205286459, -29.49034198003814566 ) ) ;
#1793=CARTESIAN_POINT ( 'NONE',  ( 2.765921099433441555, -0.3931553186911057041, -31.08824725498900676 ) ) ;
#1797=DIRECTION ( 'NONE',  ( -1.000000000000000000, -0.000000000000000000, -0.000000000000000000 ) ) ;
#1805=TOROIDAL_SURFACE ( 'NONE', #33644, 30.47050528711511674, 8.000000000000000000 ) ;
#1821=CARTESIAN_POINT ( 'NONE',  ( 2.789999999999999147, 20.99477179376825120, 22.93149026599753526 ) ) ;
#1822=CARTESIAN_POINT ( 'NONE',  ( 2.789999999999999147, -29.32277567846594835, -8.169899392883101186 ) ) ;
#1832=CARTESIAN_POINT ( 'NONE',  ( 0.000000000000000000, 12.80000000000000071, -3.000000000000000000 ) ) ;
#1833=EDGE_CURVE ( 'NONE', #1364, #11691, #30931, .T. ) ;
#1839=DIRECTION ( 'NONE',  ( 0.000000000000000000, 0.000000000000000000, 1.000000000000000000 ) ) ;
#1840=ORIENTED_EDGE ( 'NONE', *, *, #24407, .T. ) ;
#1845=ORIENTED_EDGE ( 'NONE', *, *, #34788, .F. ) ;
#1846=DIRECTION ( 'NONE',  ( 0.000000000000000000, 0.9048270524660234626, -0.4257792915650642773 ) ) ;
#1851=AXIS2_PLACEMENT_3D ( 'NONE', #14872, #12538, #26057 ) ;
#1852=ORIENTED_EDGE ( 'NONE', *, *, #29644, .T. ) ;
#1854=ORIENTED_EDGE ( 'NONE', *, *, #33044, .F. ) ;
#1869=DIRECTION ( 'NONE',  ( -1.000000000000000000, -0.000000000000000000, -0.000000000000000000 ) ) ;
#1871=CARTESIAN_POINT ( 'NONE',  ( 2.033589655505266158, -10.98355401466430337, -32.08778326630013567 ) ) ;
#1877=AXIS2_PLACEMENT_3D ( 'NONE', #3498, #19362, #16524 ) ;
#1879=CARTESIAN_POINT ( 'NONE',  ( 2.789999999999999147, 31.93991905851385837, 0.000000000000000000 ) ) ;
#1882=DIRECTION ( 'NONE',  ( -1.000000000000000000, -0.000000000000000000, -0.000000000000000000 ) ) ;
#1903=ORIENTED_EDGE ( 'NONE', *, *, #33134, .F. ) ;
#1909=CARTESIAN_POINT ( 'NONE',  ( 2.604019713817498527, 32.15598440394879987, 2.846506069495843061 ) ) ;
#1922=EDGE_CURVE ( 'NONE', #3499, #33582, #12992, .T. ) ;
#1929=DIRECTION ( 'NONE',  ( -1.000000000000000000, 0.000000000000000000, -0.000000000000000000 ) ) ;
#1939=CARTESIAN_POINT ( 'NONE',  ( 0.02407890056655564992, -30.46391896562403190, -6.211548095912885259 ) ) ;
#1956=CARTESIAN_POINT ( 'NONE',  ( 2.265105787010242011, 21.86923048072728548, -25.21799932878511896 ) ) ;
#1957=ORIENTED_EDGE ( 'NONE', *, *, #8248, .F. ) ;
#1959=EDGE_CURVE ( 'NONE', #15766, #27456, #3071, .T. ) ;
#1962=ORIENTED_EDGE ( 'NONE', *, *, #24634, .F. ) ;
#1965=DIRECTION ( 'NONE',  ( -1.000000000000000000, -0.000000000000000000, -0.000000000000000000 ) ) ;
#1982=EDGE_LOOP ( 'NONE', ( #31595, #16984, #9012, #11873, #16346, #19167 ) ) ;
#1997=ORIENTED_EDGE ( 'NONE', *, *, #1696, .T. ) ;
#2001=CARTESIAN_POINT ( 'NONE',  ( 2.790000000000080860, 27.73561032191001274, -12.87169219037303236 ) ) ;
#2003=CARTESIAN_POINT ( 'NONE',  ( 1.040000000000000924, 14.89726405156217126, 31.02351007835982344 ) ) ;
#2013=CARTESIAN_POINT ( 'NONE',  ( 0.07098929342602722237, -24.04031276246357152, -20.65449384219786211 ) ) ;
#2025=ORIENTED_EDGE ( 'NONE', *, *, #17902, .T. ) ;
#2026=CARTESIAN_POINT ( 'NONE',  ( 2.789999999999999147, -13.59935610937951900, -28.90010281771846223 ) ) ;
#2028=TOROIDAL_SURFACE ( 'NONE', #3167, 30.47050528711511674, 8.000000000000000000 ) ;
#2036=EDGE_CURVE ( 'NONE', #5629, #3012, #1511, .T. ) ;
#2041=CARTESIAN_POINT ( 'NONE',  ( 0.02407890056655825201, -23.70329957282570632, -20.11932597908854703 ) ) ;
#2047=DIRECTION ( 'NONE',  ( -1.000000000000000000, 0.000000000000000000, 0.000000000000000000 ) ) ;
#2058=DIRECTION ( 'NONE',  ( 0.000000000000000000, 0.000000000000000000, 1.000000000000000000 ) ) ;
#2061=DIRECTION ( 'NONE',  ( 0.000000000000000000, 0.000000000000000000, 1.000000000000000000 ) ) ;
#2063=DIRECTION ( 'NONE',  ( 1.000000000000000000, 0.000000000000000000, -0.000000000000000000 ) ) ;
#2067=CIRCLE ( 'NONE', #16283, 2.525000000000003020 ) ;
#2082=B_SPLINE_CURVE_WITH_KNOTS ( 'NONE', 3,
 ( #2722, #26446, #34958, #8239 ),
 .UNSPECIFIED., .F., .F.,
 ( 4, 4 ),
 ( 1.979774382698240400E-07, 0.0006879336733830264785 ),
 .UNSPECIFIED. ) ;
#2085=DIRECTION ( 'NONE',  ( 0.000000000000000000, 0.000000000000000000, 1.000000000000000000 ) ) ;
#2101=EDGE_CURVE ( 'NONE', #14860, #30400, #4774, .T. ) ;
#2108=CARTESIAN_POINT ( 'NONE',  ( 2.719051671025304984, -24.04001846604966630, -20.65402650742342061 ) ) ;
#2110=ORIENTED_EDGE ( 'NONE', *, *, #1080, .T. ) ;
#2117=EDGE_LOOP ( 'NONE', ( #2255, #11135, #14646, #758, #24030, #12999 ) ) ;
#2122=DIRECTION ( 'NONE',  ( -1.000000000000000000, -0.000000000000000000, -0.000000000000000000 ) ) ;
#2127=EDGE_CURVE ( 'NONE', #26408, #23670, #4212, .T. ) ;
#2135=DIRECTION ( 'NONE',  ( -1.000000000000000000, -0.000000000000000000, -0.000000000000000000 ) ) ;
#2136=EDGE_LOOP ( 'NONE', ( #15980, #30214, #23106, #20246 ) ) ;
#2141=AXIS2_PLACEMENT_3D ( 'NONE', #28233, #6846, #28049 ) ;
#2142=ORIENTED_EDGE ( 'NONE', *, *, #10636, .F. ) ;
#2146=CARTESIAN_POINT ( 'NONE',  ( 0.006892420738473521713, 30.38148214875513631, -5.469007969453248741 ) ) ;
#2154=CARTESIAN_POINT ( 'NONE',  ( 2.765921099433443331, 18.59128259035506758, -24.91982945642901726 ) ) ;
#2155=VECTOR ( 'NONE', #1176, 1000.000000000000000 ) ;
#2163=DIRECTION ( 'NONE',  ( -1.000000000000000000, -0.000000000000000000, -0.000000000000000000 ) ) ;
#2168=CARTESIAN_POINT ( 'NONE',  ( 2.604019716835467513, 21.49213631816418513, 24.08729967255630910 ) ) ;
#2174=EDGE_CURVE ( 'NONE', #18033, #11540, #23587, .T. ) ;
#2187=DIRECTION ( 'NONE',  ( -1.000000000000000000, -0.000000000000000000, -0.000000000000000000 ) ) ;
#2191=CARTESIAN_POINT ( 'NONE',  ( 1.749999999999999778, 27.68252950111368094, -20.44661865013457458 ) ) ;
#2192=ORIENTED_EDGE ( 'NONE', *, *, #4524, .T. ) ;
#2196=EDGE_CURVE ( 'NONE', #2517, #13256, #7869, .T. ) ;
#2199=ORIENTED_EDGE ( 'NONE', *, *, #6355, .F. ) ;
#2200=DIRECTION ( 'NONE',  ( 0.000000000000000000, 0.000000000000000000, 1.000000000000000000 ) ) ;
#2209=ORIENTED_EDGE ( 'NONE', *, *, #4188, .T. ) ;
#2217=CARTESIAN_POINT ( 'NONE',  ( 0.02407890056655564992, -30.46391896562403190, -6.211548095912885259 ) ) ;
#2221=ORIENTED_EDGE ( 'NONE', *, *, #29603, .F. ) ;
#2228=CARTESIAN_POINT ( 'NONE',  ( 2.033589660436532220, -9.974843919189428476, 32.41553303492214866 ) ) ;
#2229=ORIENTED_EDGE ( 'NONE', *, *, #4752, .T. ) ;
#2231=DIRECTION ( 'NONE',  ( -1.000000000000000000, 0.000000000000000000, 0.000000000000000000 ) ) ;
#2232=ORIENTED_EDGE ( 'NONE', *, *, #32979, .F. ) ;
#2234=VERTEX_POINT ( 'NONE', #24516 ) ;
#2241=ORIENTED_EDGE ( 'NONE', *, *, #34180, .T. ) ;
#2255=ORIENTED_EDGE ( 'NONE', *, *, #8623, .F. ) ;
#2258=CARTESIAN_POINT ( 'NONE',  ( 2.789999999999999147, 2.005524111408653720, -31.87689292423236154 ) ) ;
#2266=CARTESIAN_POINT ( 'NONE',  ( 0.7564103367120450505, 27.74660763222631132, -19.50359089280043534 ) ) ;
#2267=CARTESIAN_POINT ( 'NONE',  ( 2.719051659750488792, 28.92406410882585277, -12.95800229409215909 ) ) ;
#2274=TOROIDAL_SURFACE ( 'NONE', #27278, 30.47050528711511674, 8.000000000000000000 ) ;
#2282=ORIENTED_EDGE ( 'NONE', *, *, #5572, .F. ) ;
#2285=DIRECTION ( 'NONE',  ( -0.000000000000000000, 1.000000000000000000, 0.000000000000000000 ) ) ;
#2295=VERTEX_POINT ( 'NONE', #11547 ) ;
#2299=CYLINDRICAL_SURFACE ( 'NONE', #33443, 2.524999999999999467 ) ;
#2308=CARTESIAN_POINT ( 'NONE',  ( 2.789999999999999147, 23.28319895603578971, 21.86437915510226659 ) ) ;
#2311=CARTESIAN_POINT ( 'NONE',  ( 0.5288002570077341424, -33.38088972941606869, -0.7716149733917129216 ) ) ;
#2316=CARTESIAN_POINT ( 'NONE',  ( 2.265105789152631388, 5.490830290249586909, 32.92508943594316406 ) ) ;
#2325=ORIENTED_EDGE ( 'NONE', *, *, #5872, .T. ) ;
#2330=AXIS2_PLACEMENT_3D ( 'NONE', #23825, #21512, #16361 ) ;
#2331=ORIENTED_EDGE ( 'NONE', *, *, #3397, .F. ) ;
#2332=VECTOR ( 'NONE', #17025, 1000.000000000000000 ) ;
#2336=B_SPLINE_CURVE_WITH_KNOTS ( 'NONE', 3,
 ( #9511, #12012, #8979, #28197 ),
 .UNSPECIFIED., .F., .F.,
 ( 4, 4 ),
 ( 2.038594426256260137E-07, 0.0006242955995025980349 ),
 .UNSPECIFIED. ) ;
#2340=CARTESIAN_POINT ( 'NONE',  ( 1.040000000000001146, 6.183021911002323456, -33.85493898757056286 ) ) ;
#2341=CIRCLE ( 'NONE', #6887, 2.524999999999999467 ) ;
#2346=ORIENTED_EDGE ( 'NONE', *, *, #11507, .F. ) ;
#2350=CARTESIAN_POINT ( 'NONE',  ( 2.789999999999999147, 28.95078156989571383, -9.502838467757751317 ) ) ;
#2351=APPLICATION_CONTEXT ( 'automotive_design' ) ;
#2359=CARTESIAN_POINT ( 'NONE',  ( 2.789999999999999147, -29.00730259674844902, 9.328884633908842261 ) ) ;
#2368=ADVANCED_FACE ( 'NONE', ( #4032 ), #26990, .T. ) ;
#2369=CARTESIAN_POINT ( 'NONE',  ( 2.789999999999998703, -23.48484457444959972, 19.71282888652477538 ) ) ;
#2376=DIRECTION ( 'NONE',  ( 0.000000000000000000, 0.000000000000000000, 1.000000000000000000 ) ) ;
#2379=CARTESIAN_POINT ( 'NONE',  ( 1.749999999999999778, 0.000000000000000000, 0.000000000000000000 ) ) ;
#2381=ORIENTED_EDGE ( 'NONE', *, *, #9348, .F. ) ;
#2390=EDGE_CURVE ( 'NONE', #22410, #13078, #29117, .T. ) ;
#2397=CARTESIAN_POINT ( 'NONE',  ( 2.789999999999999147, -20.35927063852824048, 24.61013060777164796 ) ) ;
#2408=CYLINDRICAL_SURFACE ( 'NONE', #28466, 16.19999999999999574 ) ;
#2421=DIRECTION ( 'NONE',  ( -1.000000000000000000, -0.000000000000000000, 0.000000000000000000 ) ) ;
#2427=FACE_OUTER_BOUND ( 'NONE', #2848, .T. ) ;
#2428=DIRECTION ( 'NONE',  ( -1.000000000000000000, -0.000000000000000000, 0.000000000000000000 ) ) ;
#2454=VERTEX_POINT ( 'NONE', #28266 ) ;
#2456=VERTEX_POINT ( 'NONE', #26285 ) ;
#2460=DIRECTION ( 'NONE',  ( 0.000000000000000000, 0.000000000000000000, 1.000000000000000000 ) ) ;
#2464=CARTESIAN_POINT ( 'NONE',  ( 1.394999999999999574, -18.66807150955393624, -28.91175816027523027 ) ) ;
#2485=AXIS2_PLACEMENT_3D ( 'NONE', #24632, #16659, #21985 ) ;
#2490=DIRECTION ( 'NONE',  ( 1.000000000000000000, 0.000000000000000000, 0.000000000000000000 ) ) ;
#2492=CARTESIAN_POINT ( 'NONE',  ( 0.07094833732824711026, -0.5905164915254609292, -31.68852467239035420 ) ) ;
#2515=CARTESIAN_POINT ( 'NONE',  ( 2.604019710756261929, -18.30372525367464220, -26.59104308589841992 ) ) ;
#2517=VERTEX_POINT ( 'NONE', #25009 ) ;
#2518=CARTESIAN_POINT ( 'NONE',  ( -8.205391194442450056E-14, 7.412271713511258575, -29.75335163721776865 ) ) ;
#2522=CARTESIAN_POINT ( 'NONE',  ( 0.02407890056655825201, 14.63235270440936731, 27.43224275967444470 ) ) ;
#2527=TOROIDAL_SURFACE ( 'NONE', #11642, 30.47050528711512030, 8.000000000000000000 ) ;
#2531=CARTESIAN_POINT ( 'NONE',  ( 0.5248942728107164335, 7.015288891536787474, 32.63428354963185285 ) ) ;
#2540=CARTESIAN_POINT ( 'NONE',  ( 2.765921099433441999, 26.03801215795542134, -16.98986790278583570 ) ) ;
#2549=ORIENTED_EDGE ( 'NONE', *, *, #24788, .T. ) ;
#2551=ORIENTED_EDGE ( 'NONE', *, *, #10036, .F. ) ;
#2555=FACE_OUTER_BOUND ( 'NONE', #28740, .T. ) ;
#2557=ORIENTED_EDGE ( 'NONE', *, *, #25305, .F. ) ;
#2560=CARTESIAN_POINT ( 'NONE',  ( 2.789999999999999147, -26.45933846664182099, -16.32596387352474565 ) ) ;
#2567=EDGE_CURVE ( 'NONE', #8018, #25712, #5266, .T. ) ;
#2572=CARTESIAN_POINT ( 'NONE',  ( 2.790000000000000036, -30.07665394020993688, 5.960573492977232490 ) ) ;
#2577=AXIS2_PLACEMENT_3D ( 'NONE', #7021, #31756, #14894 ) ;
#2590=ORIENTED_EDGE ( 'NONE', *, *, #24493, .T. ) ;
#2592=EDGE_CURVE ( 'NONE', #18981, #33679, #10388, .T. ) ;
#2604=VERTEX_POINT ( 'NONE', #8645 ) ;
#2606=DIRECTION ( 'NONE',  ( 0.000000000000000000, 0.000000000000000000, 1.000000000000000000 ) ) ;
#2608=CARTESIAN_POINT ( 'NONE',  ( 2.604019705252365480, 7.229557500018881200, 31.46177729073544072 ) ) ;
#2610=CARTESIAN_POINT ( 'NONE',  ( 2.789999999999999147, -20.35927063852789232, -24.61013060777193218 ) ) ;
#2611=EDGE_CURVE ( 'NONE', #14020, #18600, #14001, .T. ) ;
#2620=EDGE_CURVE ( 'NONE', #32635, #26400, #25402, .T. ) ;
#2631=CARTESIAN_POINT ( 'NONE',  ( 1.395000000000002238, -33.26546734453825849, 8.820166447041648539 ) ) ;
#2632=DIRECTION ( 'NONE',  ( 1.000000000000000000, -0.000000000000000000, -0.000000000000000000 ) ) ;
#2635=VERTEX_POINT ( 'NONE', #115 ) ;
#2640=CARTESIAN_POINT ( 'NONE',  ( 0.7561992242453015045, -33.91102616014372728, 0.5305038583916231731 ) ) ;
#2642=AXIS2_PLACEMENT_3D ( 'NONE', #4328, #34068, #26576 ) ;
#2649=ORIENTED_EDGE ( 'NONE', *, *, #29824, .T. ) ;
#2652=DIRECTION ( 'NONE',  ( 0.000000000000000000, 0.000000000000000000, 1.000000000000000000 ) ) ;
#2662=CARTESIAN_POINT ( 'NONE',  ( 0.006871079570366611135, -21.36428053051087161, -22.28216981039808786 ) ) ;
#2667=VERTEX_POINT ( 'NONE', #25368 ) ;
#2669=CARTESIAN_POINT ( 'NONE',  ( 2.789999999999999147, 28.52477022197300727, 10.62590764890735606 ) ) ;
#2673=CARTESIAN_POINT ( 'NONE',  ( -10.00000000000000000, 0.000000000000000000, 0.000000000000000000 ) ) ;
#2674=DIRECTION ( 'NONE',  ( -1.000000000000000000, -0.000000000000000000, -0.000000000000000000 ) ) ;
#2679=CIRCLE ( 'NONE', #12381, 2.524999999999999467 ) ;
#2680=AXIS2_PLACEMENT_3D ( 'NONE', #26348, #23504, #18018 ) ;
#2683=CARTESIAN_POINT ( 'NONE',  ( 0.5594631266314759044, 30.83012635351326480, 13.00174666746673324 ) ) ;
#2695=ORIENTED_EDGE ( 'NONE', *, *, #4672, .T. ) ;
#2697=CARTESIAN_POINT ( 'NONE',  ( 0.02407890056655564992, -0.3931553186911057041, -31.08824725498900676 ) ) ;
#2698=DIRECTION ( 'NONE',  ( -1.000000000000000000, -0.000000000000000000, -0.000000000000000000 ) ) ;
#2711=CARTESIAN_POINT ( 'NONE',  ( 2.765921099433441555, 18.59128259035472297, 24.91982945642928016 ) ) ;
#2722=CARTESIAN_POINT ( 'NONE',  ( 0.02407890056655738464, -11.07880054387241664, 29.04985141099759360 ) ) ;
#2732=CIRCLE ( 'NONE', #5014, 34.41491905851385269 ) ;
#2737=CARTESIAN_POINT ( 'NONE',  ( 0.5248940516409021928, -29.61686074518734202, -15.39650178189456398 ) ) ;
#2739=CARTESIAN_POINT ( 'NONE',  ( 1.040000000000000480, -10.89151784028265979, -32.64600270996228204 ) ) ;
#2744=AXIS2_PLACEMENT_3D ( 'NONE', #9095, #27781, #6227 ) ;
#2753=CARTESIAN_POINT ( 'NONE',  ( 2.789999999999999147, -13.59935610937992401, 28.90010281771827039 ) ) ;
#2759=VERTEX_POINT ( 'NONE', #3650 ) ;
#2761=CARTESIAN_POINT ( 'NONE',  ( 1.394999999999999574, -10.89151784028311809, 32.64600270996213283 ) ) ;
#2772=ORIENTED_EDGE ( 'NONE', *, *, #18265, .F. ) ;
#2783=CYLINDRICAL_SURFACE ( 'NONE', #14085, 16.19999999999999574 ) ;
#2786=DIRECTION ( 'NONE',  ( 0.000000000000000000, 0.000000000000000000, 1.000000000000000000 ) ) ;
#2792=CARTESIAN_POINT ( 'NONE',  ( 2.765921099433443775, -31.05158812718220673, -1.559667679918931738 ) ) ;
#2796=EDGE_LOOP ( 'NONE', ( #16490, #1957, #8917, #16128, #9760, #32886 ) ) ;
#2800=ORIENTED_EDGE ( 'NONE', *, *, #6915, .F. ) ;
#2804=ORIENTED_EDGE ( 'NONE', *, *, #33019, .T. ) ;
#2807=ADVANCED_FACE ( 'NONE', ( #17219 ), #9362, .T. ) ;
#2820=ORIENTED_EDGE ( 'NONE', *, *, #25287, .T. ) ;
#2821=ORIENTED_EDGE ( 'NONE', *, *, #5114, .F. ) ;
#2824=CARTESIAN_POINT ( 'NONE',  ( 0.006871057928818130774, -30.82708482934414462, -1.618146408792933810 ) ) ;
#2825=CYLINDRICAL_SURFACE ( 'NONE', #28658, 2.525000000000001243 ) ;
#2829=ORIENTED_EDGE ( 'NONE', *, *, #1250, .T. ) ;
#2843=CARTESIAN_POINT ( 'NONE',  ( 1.749999999999999778, -30.02688531850407472, 16.81585001935568613 ) ) ;
#2844=DIRECTION ( 'NONE',  ( 1.000000000000000000, 0.000000000000000000, 0.000000000000000000 ) ) ;
#2848=EDGE_LOOP ( 'NONE', ( #8992, #33439, #11552, #27371 ) ) ;
#2849=EDGE_CURVE ( 'NONE', #9840, #13159, #18778, .T. ) ;
#2861=TOROIDAL_SURFACE ( 'NONE', #6348, 30.47050528711512030, 8.000000000000000000 ) ;
#2862=ORIENTED_EDGE ( 'NONE', *, *, #25345, .F. ) ;
#2874=LINE ( 'NONE', #13406, #7241 ) ;
#2879=CARTESIAN_POINT ( 'NONE',  ( 2.789999999999999147, 23.53611639059738536, -19.35207786518964213 ) ) ;
#2885=LINE ( 'NONE', #29957, #32538 ) ;
#2886=CARTESIAN_POINT ( 'NONE',  ( 2.033800775754698975, -33.91102616014372018, -0.5305038583921004580 ) ) ;
#2893=EDGE_LOOP ( 'NONE', ( #13763, #14228, #35021, #11969, #19644, #12214 ) ) ;
#2909=CARTESIAN_POINT ( 'NONE',  ( 2.789999999999999147, 7.489092610871091793, 29.53582882395389930 ) ) ;
#2913=ADVANCED_FACE ( 'NONE', ( #15941 ), #8952, .T. ) ;
#2915=CARTESIAN_POINT ( 'NONE',  ( 1.039999999999999369, -1.891117961020236216, 34.36292081097831641 ) ) ;
#2921=CARTESIAN_POINT ( 'NONE',  ( 1.256659300721212479E-17, 4.060282914029830437, -30.39157201494045779 ) ) ;
#2928=CARTESIAN_POINT ( 'NONE',  ( 2.606461819198067520, -27.67670874042536511, -16.59602520068896325 ) ) ;
#2929=CARTESIAN_POINT ( 'NONE',  ( 0.000000000000000000, 0.000000000000000000, 0.000000000000000000 ) ) ;
#2930=AXIS2_PLACEMENT_3D ( 'NONE', #4126, #18048, #4472 ) ;
#2936=CIRCLE ( 'NONE', #21693, 2.525000000000003020 ) ;
#2947=CARTESIAN_POINT ( 'NONE',  ( 0.006892384605615998854, -17.88431215799113971, -25.16139613958922894 ) ) ;
#2950=VERTEX_POINT ( 'NONE', #12734 ) ;
#2963=CARTESIAN_POINT ( 'NONE',  ( 0.7561992021476438008, -17.72251720152558008, 28.91628452940440752 ) ) ;
#2966=ORIENTED_EDGE ( 'NONE', *, *, #32440, .F. ) ;
#2967=AXIS2_PLACEMENT_3D ( 'NONE', #13018, #15203, #23850 ) ;
#2968=EDGE_CURVE ( 'NONE', #8710, #18246, #11277, .T. ) ;
#2973=CARTESIAN_POINT ( 'NONE',  ( 2.765921099433442443, 30.61125888652961891, 5.439165181699118889 ) ) ;
#2985=CARTESIAN_POINT ( 'NONE',  ( 0.07094832897469352528, -24.04001846604995762, 20.65402650742307955 ) ) ;
#2996=DIRECTION ( 'NONE',  ( -1.000000000000000000, -0.000000000000000000, -0.000000000000000000 ) ) ;
#2997=DIRECTION ( 'NONE',  ( 0.000000000000000000, -0.8443279255020161855, 0.5358267949789948803 ) ) ;
#3010=EDGE_CURVE ( 'NONE', #5255, #939, #27647, .T. ) ;
#3012=VERTEX_POINT ( 'NONE', #595 ) ;
#3015=CARTESIAN_POINT ( 'NONE',  ( 0.02407890056655651728, 7.350529080603541487, 30.20932655202940254 ) ) ;
#3025=CYLINDRICAL_SURFACE ( 'NONE', #26247, 16.19999999999999574 ) ;
#3031=CIRCLE ( 'NONE', #17300, 2.524999999999999467 ) ;
#3033=DIRECTION ( 'NONE',  ( -1.000000000000000000, 0.000000000000000000, -0.000000000000000000 ) ) ;
#3040=CARTESIAN_POINT ( 'NONE',  ( 2.789999999999999147, -30.41598411195409923, 1.821977758773558165 ) ) ;
#3057=FACE_OUTER_BOUND ( 'NONE', #15149, .T. ) ;
#3067=CARTESIAN_POINT ( 'NONE',  ( 2.789999999999999147, 27.98916443103621177, -15.38717335695007904 ) ) ;
#3071=CIRCLE ( 'NONE', #3660, 10.00000000000000000 ) ;
#3074=ADVANCED_FACE ( 'NONE', ( #5920 ), #7827, .T. ) ;
#3079=ORIENTED_EDGE ( 'NONE', *, *, #16775, .T. ) ;
#3080=CARTESIAN_POINT ( 'NONE',  ( 2.789999999999999147, 30.61125888652969707, -5.439165181698684570 ) ) ;
#3083=CARTESIAN_POINT ( 'NONE',  ( 8.000000000000000000, 0.000000000000000000, 0.000000000000000000 ) ) ;
#3090=VECTOR ( 'NONE', #31667, 1000.000000000000000 ) ;
#3094=EDGE_CURVE ( 'NONE', #22708, #14860, #23994, .T. ) ;
#3099=ORIENTED_EDGE ( 'NONE', *, *, #33722, .T. ) ;
#3101=CARTESIAN_POINT ( 'NONE',  ( 2.789999999999999147, -21.56796757982795043, -22.39322359481629476 ) ) ;
#3103=CARTESIAN_POINT ( 'NONE',  ( 0.07094834073506586791, -30.32005755872678776, -9.230678093032972598 ) ) ;
#3106=VERTEX_POINT ( 'NONE', #1302 ) ;
#3109=CARTESIAN_POINT ( 'NONE',  ( 1.749999999999999778, 31.89769921722987434, 12.91988538846969803 ) ) ;
#3111=VERTEX_POINT ( 'NONE', #3952 ) ;
#3121=ORIENTED_EDGE ( 'NONE', *, *, #25985, .F. ) ;
#3124=ORIENTED_EDGE ( 'NONE', *, *, #4524, .F. ) ;
#3133=CARTESIAN_POINT ( 'NONE',  ( 0.000000000000000000, 30.40449935640661039, 2.004522720844265304 ) ) ;
#3136=DIRECTION ( 'NONE',  ( 0.000000000000000000, 0.000000000000000000, 1.000000000000000000 ) ) ;
#3138=CARTESIAN_POINT ( 'NONE',  ( 1.039999999999999813, 14.89726405156260114, -31.02351007835961383 ) ) ;
#3141=ORIENTED_EDGE ( 'NONE', *, *, #25780, .T. ) ;
#3142=TOROIDAL_SURFACE ( 'NONE', #7680, 30.47050528711511674, 8.000000000000000000 ) ;
#3151=DIRECTION ( 'NONE',  ( 0.000000000000000000, 0.000000000000000000, 1.000000000000000000 ) ) ;
#3154=ORIENTED_EDGE ( 'NONE', *, *, #12208, .F. ) ;
#3160=ORIENTED_EDGE ( 'NONE', *, *, #8197, .F. ) ;
#3166=ORIENTED_EDGE ( 'NONE', *, *, #32162, .F. ) ;
#3167=AXIS2_PLACEMENT_3D ( 'NONE', #28712, #31212, #3796 ) ;
#3178=ADVANCED_FACE ( 'NONE', ( #30503 ), #6098, .F. ) ;
#3181=ORIENTED_EDGE ( 'NONE', *, *, #13503, .T. ) ;
#3189=ORIENTED_EDGE ( 'NONE', *, *, #11960, .T. ) ;
#3192=EDGE_LOOP ( 'NONE', ( #16759, #10547, #21688, #33457, #35003, #10147 ) ) ;
#3196=CARTESIAN_POINT ( 'NONE',  ( 2.789999999999999147, -0.3931553186915530129, 31.08824725498900321 ) ) ;
#3199=DIRECTION ( 'NONE',  ( 1.000000000000000000, 0.000000000000000000, 0.000000000000000000 ) ) ;
#3213=EDGE_CURVE ( 'NONE', #5389, #22114, #19236, .T. ) ;
#3215=ORIENTED_EDGE ( 'NONE', *, *, #32034, .F. ) ;
#3220=VERTEX_POINT ( 'NONE', #28360 ) ;
#3222=CARTESIAN_POINT ( 'NONE',  ( 2.789999999999999147, 24.98605633783575897, -17.38589710834512658 ) ) ;
#3231=B_SPLINE_CURVE_WITH_KNOTS ( 'NONE', 3,
 ( #20756, #7206, #12930, #4528 ),
 .UNSPECIFIED., .F., .F.,
 ( 4, 4 ),
 ( 3.668583969174124871E-07, 0.0006881039678812997601 ),
 .UNSPECIFIED. ) ;
#3242=VECTOR ( 'NONE', #18530, 1000.000000000000000 ) ;
#3243=EDGE_CURVE ( 'NONE', #29665, #2517, #28645, .T. ) ;
#3245=VERTEX_POINT ( 'NONE', #15362 ) ;
#3265=ORIENTED_EDGE ( 'NONE', *, *, #21739, .F. ) ;
#3269=DIRECTION ( 'NONE',  ( -1.000000000000000000, 0.000000000000000000, 0.000000000000000000 ) ) ;
#3278=EDGE_CURVE ( 'NONE', #10268, #4330, #12402, .T. ) ;
#3281=CARTESIAN_POINT ( 'NONE',  ( 1.040000000000001590, -33.26546734453813059, -8.820166447042128155 ) ) ;
#3300=DIRECTION ( 'NONE',  ( -1.000000000000000000, -0.000000000000000000, 0.000000000000000000 ) ) ;
#3301=ORIENTED_EDGE ( 'NONE', *, *, #13740, .F. ) ;
#3302=ORIENTED_EDGE ( 'NONE', *, *, #15393, .F. ) ;
#3308=ORIENTED_EDGE ( 'NONE', *, *, #19543, .T. ) ;
#3312=CARTESIAN_POINT ( 'NONE',  ( 0.000000000000000000, -27.53147453683416757, -13.05640081644872197 ) ) ;
#3321=CARTESIAN_POINT ( 'NONE',  ( 1.749999999999999778, -33.26546734453825849, 8.820166447041632551 ) ) ;
#3322=DIRECTION ( 'NONE',  ( -1.000000000000000000, -0.000000000000000000, -0.000000000000000000 ) ) ;
#3323=VECTOR ( 'NONE', #28186, 1000.000000000000000 ) ;
#3325=DIRECTION ( 'NONE',  ( -1.000000000000000000, -0.000000000000000000, -0.000000000000000000 ) ) ;
#3334=CARTESIAN_POINT ( 'NONE',  ( 0.000000000000000000, -7.666252171205713672, 29.49034198003804974 ) ) ;
#3340=FACE_OUTER_BOUND ( 'NONE', #18173, .T. ) ;
#3342=CARTESIAN_POINT ( 'NONE',  ( 0.5288002468691824776, -9.581412748858038952, -31.98555481955064295 ) ) ;
#3344=DIRECTION ( 'NONE',  ( 0.000000000000000000, 0.000000000000000000, 1.000000000000000000 ) ) ;
#3346=CARTESIAN_POINT ( 'NONE',  ( 2.789999999999999147, 27.60935207499552035, 12.89090262359662731 ) ) ;
#3366=EDGE_CURVE ( 'NONE', #25284, #27727, #29228, .T. ) ;
#3380=ORIENTED_EDGE ( 'NONE', *, *, #16494, .T. ) ;
#3384=CARTESIAN_POINT ( 'NONE',  ( 2.606462031291651993, 12.63602821951805133, 29.69442701139049134 ) ) ;
#3392=DIRECTION ( 'NONE',  ( -1.000000000000000000, -0.000000000000000000, -0.000000000000000000 ) ) ;
#3393=FACE_OUTER_BOUND ( 'NONE', #18212, .T. ) ;
#3397=EDGE_CURVE ( 'NONE', #7267, #34651, #12693, .T. ) ;
#3399=CARTESIAN_POINT ( 'NONE',  ( 2.783107613148426029, -27.79373726981387449, 13.43326644626213806 ) ) ;
#3416=DIRECTION ( 'NONE',  ( 0.000000000000000000, 0.000000000000000000, -1.000000000000000000 ) ) ;
#3422=CARTESIAN_POINT ( 'NONE',  ( 2.790000000000000924, 0.000000000000000000, 0.000000000000000000 ) ) ;
#3441=CARTESIAN_POINT ( 'NONE',  ( 0.5248942630475922355, -2.869810969760784314, -33.25620129461683661 ) ) ;
#3451=EDGE_CURVE ( 'NONE', #6854, #18398, #14229, .T. ) ;
#3469=FACE_OUTER_BOUND ( 'NONE', #30331, .T. ) ;
#3474=DIRECTION ( 'NONE',  ( -1.000000000000000000, 0.000000000000000000, -0.000000000000000000 ) ) ;
#3491=LINE ( 'NONE', #28061, #32689 ) ;
#3493=CIRCLE ( 'NONE', #12033, 30.47050528711512030 ) ;
#3495=ORIENTED_EDGE ( 'NONE', *, *, #18707, .F. ) ;
#3496=ADVANCED_FACE ( 'NONE', ( #26899 ), #11071, .T. ) ;
#3498=CARTESIAN_POINT ( 'NONE',  ( 0.000000000000000000, 0.000000000000000000, 0.000000000000000000 ) ) ;
#3499=VERTEX_POINT ( 'NONE', #29933 ) ;
#3502=AXIS2_PLACEMENT_3D ( 'NONE', #10283, #12969, #7958 ) ;
#3505=CARTESIAN_POINT ( 'NONE',  ( 1.749999999999999778, 31.89769921722987434, 12.91988538846969803 ) ) ;
#3509=ORIENTED_EDGE ( 'NONE', *, *, #12209, .T. ) ;
#3513=CARTESIAN_POINT ( 'NONE',  ( 2.789999999999999591, 0.000000000000000000, -3.000000000000000000 ) ) ;
#3516=EDGE_CURVE ( 'NONE', #949, #4047, #24333, .T. ) ;
#3522=ORIENTED_EDGE ( 'NONE', *, *, #30033, .F. ) ;
#3526=CARTESIAN_POINT ( 'NONE',  ( 2.789999999999999147, 17.11426446101199161, 26.96776559937732642 ) ) ;
#3532=AXIS2_PLACEMENT_3D ( 'NONE', #27531, #3325, #27349 ) ;
#3541=ORIENTED_EDGE ( 'NONE', *, *, #32779, .T. ) ;
#3548=EDGE_CURVE ( 'NONE', #18398, #25712, #33233, .T. ) ;
#3553=VECTOR ( 'NONE', #4364, 1000.000000000000000 ) ;
#3559=ADVANCED_FACE ( 'NONE', ( #11414 ), #500, .T. ) ;
#3567=ORIENTED_EDGE ( 'NONE', *, *, #33673, .F. ) ;
#3574=CARTESIAN_POINT ( 'NONE',  ( 2.789999999999999147, -23.70329957282599764, 20.11932597908820242 ) ) ;
#3582=CYLINDRICAL_SURFACE ( 'NONE', #21847, 2.524999999999999467 ) ;
#3585=CARTESIAN_POINT ( 'NONE',  ( 0.02407890056655738464, -11.07880054387200985, -29.04985141099774637 ) ) ;
#3591=EDGE_CURVE ( 'NONE', #25806, #32541, #4082, .T. ) ;
#3595=B_SPLINE_CURVE_WITH_KNOTS ( 'NONE', 3,
 ( #30959, #6564, #34142, #28808, #17980, #15299 ),
 .UNSPECIFIED., .F., .F.,
 ( 4, 2, 4 ),
 ( 2.333473478908865889E-07, 0.001873431678079538970, 0.003746630008811186949 ),
 .UNSPECIFIED. ) ;
#3596=ADVANCED_FACE ( 'NONE', ( #3393 ), #31164, .T. ) ;
#3611=CARTESIAN_POINT ( 'NONE',  ( 2.033800777031441243, -1.599833918847377801, -33.87742110695038633 ) ) ;
#3620=ORIENTED_EDGE ( 'NONE', *, *, #30632, .T. ) ;
#3633=CARTESIAN_POINT ( 'NONE',  ( 0.02407890056655695096, 30.61125888652961891, 5.439165181699118889 ) ) ;
#3638=VECTOR ( 'NONE', #28264, 1000.000000000000000 ) ;
#3642=ORIENTED_EDGE ( 'NONE', *, *, #32787, .T. ) ;
#3648=LINE ( 'NONE', #11158, #1667 ) ;
#3649=AXIS2_PLACEMENT_3D ( 'NONE', #10378, #4660, #26919 ) ;
#3650=CARTESIAN_POINT ( 'NONE',  ( 2.789999999999999147, -25.77598557799260703, 16.24962337825793313 ) ) ;
#3651=CARTESIAN_POINT ( 'NONE',  ( 0.1835381989597825725, 31.84255742294098113, -5.242117949250411080 ) ) ;
#3652=EDGE_CURVE ( 'NONE', #18208, #7089, #8442, .T. ) ;
#3657=CARTESIAN_POINT ( 'NONE',  ( 0.7564103407256241862, -32.97789401874111093, 7.919772684712727440 ) ) ;
#3660=AXIS2_PLACEMENT_3D ( 'NONE', #3422, #6260, #19651 ) ;
#3664=DIRECTION ( 'NONE',  ( 0.000000000000000000, 0.000000000000000000, 1.000000000000000000 ) ) ;
#3668=ADVANCED_FACE ( 'NONE', ( #30810 ), #25458, .T. ) ;
#3677=ORIENTED_EDGE ( 'NONE', *, *, #21645, .F. ) ;
#3689=CARTESIAN_POINT ( 'NONE',  ( 2.783128731155445124, -30.26101440722778335, -6.099076262612814325 ) ) ;
#3695=DIRECTION ( 'NONE',  ( -1.000000000000000000, -0.000000000000000000, -0.000000000000000000 ) ) ;
#3709=VECTOR ( 'NONE', #2632, 1000.000000000000000 ) ;
#3710=CARTESIAN_POINT ( 'NONE',  ( 0.02407890056655781832, 18.59128259035472297, 24.91982945642928016 ) ) ;
#3725=ADVANCED_FACE ( 'NONE', ( #16956 ), #33999, .F. ) ;
#3728=B_SPLINE_CURVE_WITH_KNOTS ( 'NONE', 3,
 ( #25457, #1088, #8556, #11956, #19436, #30274 ),
 .UNSPECIFIED., .F., .F.,
 ( 4, 2, 4 ),
 ( 2.073839991540172406E-07, 0.001873405686414694694, 0.003746603988830235401 ),
 .UNSPECIFIED. ) ;
#3730=FACE_OUTER_BOUND ( 'NONE', #9143, .T. ) ;
#3744=ORIENTED_EDGE ( 'NONE', *, *, #17853, .T. ) ;
#3746=VECTOR ( 'NONE', #18434, 1000.000000000000000 ) ;
#3748=CARTESIAN_POINT ( 'NONE',  ( 2.789999999999999147, 0.000000000000000000, 0.000000000000000000 ) ) ;
#3753=CARTESIAN_POINT ( 'NONE',  ( 2.789999999999999147, 24.25608676733002156, -18.39061402768334119 ) ) ;
#3754=CARTESIAN_POINT ( 'NONE',  ( 0.000000000000000000, 27.98916443103621177, -15.38717335695007904 ) ) ;
#3764=CARTESIAN_POINT ( 'NONE',  ( 0.07098931461607634053, 31.58942871418359744, 2.579295332369118565 ) ) ;
#3766=CARTESIAN_POINT ( 'NONE',  ( 2.765921099433440666, -8.112136323388726922, -30.01377904834218668 ) ) ;
#3778=ORIENTED_EDGE ( 'NONE', *, *, #3839, .T. ) ;
#3781=ORIENTED_EDGE ( 'NONE', *, *, #28415, .F. ) ;
#3782=EDGE_LOOP ( 'NONE', ( #23329, #34940, #22038, #30078 ) ) ;
#3783=FACE_OUTER_BOUND ( 'NONE', #33989, .T. ) ;
#3790=FACE_OUTER_BOUND ( 'NONE', #5666, .T. ) ;
#3791=CARTESIAN_POINT ( 'NONE',  ( 0.006871051096725699914, -29.45617853245860118, -9.233693611950151592 ) ) ;
#3796=DIRECTION ( 'NONE',  ( 0.000000000000000000, 0.000000000000000000, 1.000000000000000000 ) ) ;
#3806=DIRECTION ( 'NONE',  ( 0.000000000000000000, 0.000000000000000000, 1.000000000000000000 ) ) ;
#3807=ORIENTED_EDGE ( 'NONE', *, *, #30479, .F. ) ;
#3808=ADVANCED_FACE ( 'NONE', ( #12478 ), #23489, .T. ) ;
#3830=DIRECTION ( 'NONE',  ( -1.000000000000000000, 0.000000000000000000, -0.000000000000000000 ) ) ;
#3839=EDGE_CURVE ( 'NONE', #33582, #693, #18890, .T. ) ;
#3844=DIRECTION ( 'NONE',  ( -1.000000000000000000, -0.000000000000000000, -0.000000000000000000 ) ) ;
#3847=DIRECTION ( 'NONE',  ( 0.000000000000000000, 0.000000000000000000, 1.000000000000000000 ) ) ;
#3856=CARTESIAN_POINT ( 'NONE',  ( 2.789999999999999147, -25.77598557799260703, 16.24962337825793313 ) ) ;
#3862=ORIENTED_EDGE ( 'NONE', *, *, #13178, .T. ) ;
#3865=CARTESIAN_POINT ( 'NONE',  ( 8.000000000000000000, 0.000000000000000000, 0.000000000000000000 ) ) ;
#3872=CARTESIAN_POINT ( 'NONE',  ( 2.789999999999999147, -5.984944020945660803, -28.84917528048448787 ) ) ;
#3876=ORIENTED_EDGE ( 'NONE', *, *, #6661, .T. ) ;
#3877=CARTESIAN_POINT ( 'NONE',  ( 2.719010698802078796, -31.01706505092339228, 6.518161977769513449 ) ) ;
#3888=CARTESIAN_POINT ( 'NONE',  ( 0.000000000000000000, -0.09145294252657359957, -30.47036804522409525 ) ) ;
#3892=ADVANCED_FACE ( 'NONE', ( #18700 ), #34052, .T. ) ;
#3895=UNCERTAINTY_MEASURE_WITH_UNIT (LENGTH_MEASURE( 1.000000000000000082E-05 ), #25844, 'distance_accuracy_value', 'NONE');
#3898=ORIENTED_EDGE ( 'NONE', *, *, #28327, .F. ) ;
#3902=ORIENTED_EDGE ( 'NONE', *, *, #4188, .F. ) ;
#3905=FACE_OUTER_BOUND ( 'NONE', #14944, .T. ) ;
#3914=DIRECTION ( 'NONE',  ( -1.000000000000000000, 0.000000000000000000, 0.000000000000000000 ) ) ;
#3917=CARTESIAN_POINT ( 'NONE',  ( 2.789999999999999147, 23.28319895603611300, -21.86437915510192909 ) ) ;
#3921=ORIENTED_EDGE ( 'NONE', *, *, #18983, .F. ) ;
#3939=ORIENTED_EDGE ( 'NONE', *, *, #9917, .T. ) ;
#3940=ORIENTED_EDGE ( 'NONE', *, *, #28690, .F. ) ;
#3943=EDGE_LOOP ( 'NONE', ( #16572, #34885, #28217, #16509, #8418, #26069 ) ) ;
#3950=EDGE_CURVE ( 'NONE', #25284, #21475, #26063, .T. ) ;
#3952=CARTESIAN_POINT ( 'NONE',  ( 0.000000000000000000, -11.13185981125856294, -28.36429779836965182 ) ) ;
#3967=B_SPLINE_CURVE_WITH_KNOTS ( 'NONE', 3,
 ( #15599, #31136, #26609, #5061, #26435, #1231 ),
 .UNSPECIFIED., .F., .F.,
 ( 4, 2, 4 ),
 ( 2.699892340800535851E-07, 0.001873468359918846558, 0.003746666730603612824 ),
 .UNSPECIFIED. ) ;
#3975=CARTESIAN_POINT ( 'NONE',  ( 2.719051662671754244, -0.5905164915259186742, 31.68852467239034709 ) ) ;
#3977=CARTESIAN_POINT ( 'NONE',  ( 2.789999999999999147, 29.44518845714779332, -9.980709654879110104 ) ) ;
#3978=CYLINDRICAL_SURFACE ( 'NONE', #16082, 2.524999999999999467 ) ;
#3981=DIRECTION ( 'NONE',  ( -1.000000000000000000, -0.000000000000000000, -0.000000000000000000 ) ) ;
#3994=DIRECTION ( 'NONE',  ( -1.000000000000000000, 0.000000000000000000, 0.000000000000000000 ) ) ;
#3995=CARTESIAN_POINT ( 'NONE',  ( 0.5248942691478599709, 33.01038087096675611, -4.952322205614974493 ) ) ;
#4005=AXIS2_PLACEMENT_3D ( 'NONE', #8397, #16430, #22457 ) ;
#4007=ORIENTED_EDGE ( 'NONE', *, *, #15393, .T. ) ;
#4010=CARTESIAN_POINT ( 'NONE',  ( 2.789999999999999147, -11.13185981125896795, 28.36429779836946352 ) ) ;
#4015=CIRCLE ( 'NONE', #22786, 2.525000000000000799 ) ;
#4019=ORIENTED_EDGE ( 'NONE', *, *, #10405, .F. ) ;
#4027=CARTESIAN_POINT ( 'NONE',  ( 2.789999999999999147, -25.83993731729781729, -16.24881338200996694 ) ) ;
#4032=FACE_OUTER_BOUND ( 'NONE', #7499, .T. ) ;
#4037=VECTOR ( 'NONE', #15730, 1000.000000000000000 ) ;
#4044=EDGE_CURVE ( 'NONE', #31622, #9953, #27215, .T. ) ;
#4047=VERTEX_POINT ( 'NONE', #1008 ) ;
#4051=EDGE_CURVE ( 'NONE', #527, #5845, #21767, .T. ) ;
#4056=DIRECTION ( 'NONE',  ( -1.000000000000000000, 0.000000000000000000, 0.000000000000000000 ) ) ;
#4072=CARTESIAN_POINT ( 'NONE',  ( 2.789999999999999147, -29.00730259674831757, -9.328884633909261481 ) ) ;
#4074=DIRECTION ( 'NONE',  ( 0.000000000000000000, 0.000000000000000000, 1.000000000000000000 ) ) ;
#4082=LINE ( 'NONE', #22800, #25487 ) ;
#4083=ORIENTED_EDGE ( 'NONE', *, *, #5194, .T. ) ;
#4087=LINE ( 'NONE', #31506, #28226 ) ;
#4097=CARTESIAN_POINT ( 'NONE',  ( 0.02407890056655651728, 18.59128259035506758, -24.91982945642901726 ) ) ;
#4116=ORIENTED_EDGE ( 'NONE', *, *, #926, .T. ) ;
#4121=DIRECTION ( 'NONE',  ( -1.000000000000000000, -0.000000000000000000, -0.000000000000000000 ) ) ;
#4123=ORIENTED_EDGE ( 'NONE', *, *, #8999, .F. ) ;
#4126=CARTESIAN_POINT ( 'NONE',  ( 0.000000000000000000, 0.000000000000000000, 0.000000000000000000 ) ) ;
#4128=ORIENTED_EDGE ( 'NONE', *, *, #32403, .T. ) ;
#4129=EDGE_CURVE ( 'NONE', #13694, #12785, #17746, .T. ) ;
#4142=EDGE_LOOP ( 'NONE', ( #16622, #6608, #22354, #24302 ) ) ;
#4147=CARTESIAN_POINT ( 'NONE',  ( 0.000000000000000000, 14.59907093257217170, 26.74544485249471393 ) ) ;
#4154=DIRECTION ( 'NONE',  ( -1.000000000000000000, -0.000000000000000000, -0.000000000000000000 ) ) ;
#4159=EDGE_LOOP ( 'NONE', ( #13622, #22176, #15776, #27684 ) ) ;
#4174=DIRECTION ( 'NONE',  ( 0.000000000000000000, 0.000000000000000000, 1.000000000000000000 ) ) ;
#4175=ORIENTED_EDGE ( 'NONE', *, *, #27568, .F. ) ;
#4187=ORIENTED_EDGE ( 'NONE', *, *, #11783, .T. ) ;
#4188=EDGE_CURVE ( 'NONE', #16780, #1364, #23588, .T. ) ;
#4199=EDGE_CURVE ( 'NONE', #23325, #5785, #6757, .T. ) ;
#4200=EDGE_CURVE ( 'NONE', #14739, #28456, #6512, .T. ) ;
#4212=CIRCLE ( 'NONE', #27523, 30.47050528711511674 ) ;
#4242=CARTESIAN_POINT ( 'NONE',  ( 0.02407890056655695096, -26.45933846664205902, 16.32596387352436551 ) ) ;
#4244=CARTESIAN_POINT ( 'NONE',  ( 0.000000000000000000, -13.59935610937951900, -28.90010281771846223 ) ) ;
#4247=AXIS2_PLACEMENT_3D ( 'NONE', #25281, #25807, #6584 ) ;
#4251=TOROIDAL_SURFACE ( 'NONE', #11678, 30.47050528711512030, 8.000000000000000000 ) ;
#4255=AXIS2_PLACEMENT_3D ( 'NONE', #24678, #22031, #3151 ) ;
#4256=FACE_OUTER_BOUND ( 'NONE', #1982, .T. ) ;
#4268=CARTESIAN_POINT ( 'NONE',  ( 0.000000000000000000, 30.40449935640661039, 2.004522720844265304 ) ) ;
#4291=ORIENTED_EDGE ( 'NONE', *, *, #18038, .F. ) ;
#4293=DIRECTION ( 'NONE',  ( -1.000000000000000000, 0.000000000000000000, 0.000000000000000000 ) ) ;
#4297=DIRECTION ( 'NONE',  ( -1.000000000000000000, -0.000000000000000000, -0.000000000000000000 ) ) ;
#4302=CARTESIAN_POINT ( 'NONE',  ( 0.7564103425703777583, 27.12319051591914487, 20.36165095825682414 ) ) ;
#4303=ORIENTED_EDGE ( 'NONE', *, *, #29931, .F. ) ;
#4328=CARTESIAN_POINT ( 'NONE',  ( 0.000000000000000000, -31.68806325674604452, -4.003133335385915537 ) ) ;
#4329=AXIS2_PLACEMENT_3D ( 'NONE', #5622, #19357, #14199 ) ;
#4330=VERTEX_POINT ( 'NONE', #2739 ) ;
#4335=ORIENTED_EDGE ( 'NONE', *, *, #25985, .T. ) ;
#4339=ORIENTED_EDGE ( 'NONE', *, *, #18971, .F. ) ;
#4351=CARTESIAN_POINT ( 'NONE',  ( 50.00050000000000239, 9.539392014169456147, 3.000000000000000000 ) ) ;
#4353=CARTESIAN_POINT ( 'NONE',  ( 2.765921099433441999, -31.05158812718222450, 1.559667679918499417 ) ) ;
#4361=CARTESIAN_POINT ( 'NONE',  ( 0.000000000000000000, -14.75935258146432005, 26.65732927035515232 ) ) ;
#4363=FACE_OUTER_BOUND ( 'NONE', #4142, .T. ) ;
#4364=DIRECTION ( 'NONE',  ( -1.000000000000000000, 0.000000000000000000, 0.000000000000000000 ) ) ;
#4367=EDGE_LOOP ( 'NONE', ( #33169, #27149, #32648, #21965, #16147, #24832, #24199 ) ) ;
#4373=CIRCLE ( 'NONE', #23725, 34.41491905851385269 ) ;
#4374=EDGE_LOOP ( 'NONE', ( #22803, #11011, #12293, #32546, #30410, #4291 ) ) ;
#4376=CARTESIAN_POINT ( 'NONE',  ( 2.789999999999999147, -14.75935258146429341, 26.65732927035513811 ) ) ;
#4399=CARTESIAN_POINT ( 'NONE',  ( 2.261199745872888744, 33.21438043751174973, 3.418204286533153446 ) ) ;
#4404=DIRECTION ( 'NONE',  ( 0.000000000000000000, 0.000000000000000000, 1.000000000000000000 ) ) ;
#4415=VERTEX_POINT ( 'NONE', #23203 ) ;
#4423=CARTESIAN_POINT ( 'NONE',  ( 0.7561992169675183506, -32.97757984916171381, -7.919492155588399918 ) ) ;
#4446=CARTESIAN_POINT ( 'NONE',  ( 0.02407890056655564992, 31.00221527374952046, 2.344426712874309260 ) ) ;
#4450=CARTESIAN_POINT ( 'NONE',  ( 1.040000000000001812, -34.41385771548413430, -0.2702793785573777696 ) ) ;
#4451=FACE_OUTER_BOUND ( 'NONE', #6884, .T. ) ;
#4454=CARTESIAN_POINT ( 'NONE',  ( 2.789999999999999147, 28.06759692514783922, -11.78059558880183921 ) ) ;
#4462=CARTESIAN_POINT ( 'NONE',  ( 1.749999999999999778, 0.000000000000000000, 0.000000000000000000 ) ) ;
#4472=DIRECTION ( 'NONE',  ( 0.000000000000000000, 0.000000000000000000, 1.000000000000000000 ) ) ;
#4486=CYLINDRICAL_SURFACE ( 'NONE', #7347, 16.19999999999999218 ) ;
#4487=ORIENTED_EDGE ( 'NONE', *, *, #6509, .T. ) ;
#4490=EDGE_CURVE ( 'NONE', #23180, #25989, #15874, .T. ) ;
#4497=CARTESIAN_POINT ( 'NONE',  ( 2.765921099433441555, 18.59128259035472297, 24.91982945642928016 ) ) ;
#4503=AXIS2_PLACEMENT_3D ( 'NONE', #3753, #12314, #22456 ) ;
#4504=ORIENTED_EDGE ( 'NONE', *, *, #19900, .F. ) ;
#4509=CARTESIAN_POINT ( 'NONE',  ( 8.000000000000000000, 0.000000000000000000, 0.000000000000000000 ) ) ;
#4510=DIRECTION ( 'NONE',  ( 0.000000000000000000, 0.000000000000000000, 1.000000000000000000 ) ) ;
#4517=CARTESIAN_POINT ( 'NONE',  ( 0.000000000000000000, 11.30192140231274500, -28.29696565125059493 ) ) ;
#4518=CARTESIAN_POINT ( 'NONE',  ( 1.394999999999999574, 22.14447232807506438, 26.34405054495565679 ) ) ;
#4520=AXIS2_PLACEMENT_3D ( 'NONE', #11723, #6536, #20085 ) ;
#4524=EDGE_CURVE ( 'NONE', #34913, #18033, #33683, .T. ) ;
#4528=CARTESIAN_POINT ( 'NONE',  ( 2.789999999999999147, -7.666252171205694133, 29.49034198003803198 ) ) ;
#4529=DIRECTION ( 'NONE',  ( 0.000000000000000000, 0.000000000000000000, 1.000000000000000000 ) ) ;
#4534=LINE ( 'NONE', #21106, #9445 ) ;
#4541=ORIENTED_EDGE ( 'NONE', *, *, #8957, .F. ) ;
#4542=CIRCLE ( 'NONE', #28433, 30.47050528711511674 ) ;
#4545=ORIENTED_EDGE ( 'NONE', *, *, #10903, .T. ) ;
#4549=EDGE_CURVE ( 'NONE', #7253, #9347, #147, .T. ) ;
#4557=CARTESIAN_POINT ( 'NONE',  ( 1.040000000000000258, 28.00026196654270905, 20.00929742917132614 ) ) ;
#4562=EDGE_CURVE ( 'NONE', #2950, #2759, #23291, .T. ) ;
#4566=VECTOR ( 'NONE', #10233, 1000.000000000000000 ) ;
#4567=FACE_OUTER_BOUND ( 'NONE', #29904, .T. ) ;
#4569=VECTOR ( 'NONE', #28439, 1000.000000000000000 ) ;
#4577=TOROIDAL_SURFACE ( 'NONE', #1205, 30.47050528711512030, 8.000000000000000000 ) ;
#4581=EDGE_CURVE ( 'NONE', #31215, #10268, #15728, .T. ) ;
#4589=CARTESIAN_POINT ( 'NONE',  ( 0.000000000000000000, 0.000000000000000000, 0.000000000000000000 ) ) ;
#4601=VERTEX_POINT ( 'NONE', #34752 ) ;
#4602=CIRCLE ( 'NONE', #30781, 34.41491905851385269 ) ;
#4605=CARTESIAN_POINT ( 'NONE',  ( 2.789999999999999147, -11.13185981125896795, 28.36429779836946352 ) ) ;
#4614=FACE_OUTER_BOUND ( 'NONE', #21775, .T. ) ;
#4615=DIRECTION ( 'NONE',  ( 1.000000000000000000, 0.000000000000000000, -0.000000000000000000 ) ) ;
#4632=ORIENTED_EDGE ( 'NONE', *, *, #9637, .T. ) ;
#4633=FACE_OUTER_BOUND ( 'NONE', #20108, .T. ) ;
#4644=ORIENTED_EDGE ( 'NONE', *, *, #21449, .F. ) ;
#4645=CARTESIAN_POINT ( 'NONE',  ( 0.02407890056655781832, 4.286445725888479608, -30.79383171238939809 ) ) ;
#4655=ORIENTED_EDGE ( 'NONE', *, *, #31078, .F. ) ;
#4660=DIRECTION ( 'NONE',  ( -1.000000000000000000, 0.000000000000000000, 0.000000000000000000 ) ) ;
#4668=EDGE_CURVE ( 'NONE', #9316, #28134, #26201, .T. ) ;
#4669=EDGE_CURVE ( 'NONE', #16394, #14153, #12022, .T. ) ;
#4672=EDGE_CURVE ( 'NONE', #16780, #8132, #23267, .T. ) ;
#4680=ORIENTED_EDGE ( 'NONE', *, *, #12361, .F. ) ;
#4682=CARTESIAN_POINT ( 'NONE',  ( 2.765921099433442443, 28.29688452313417812, -12.88099432405573630 ) ) ;
#4685=DIRECTION ( 'NONE',  ( 0.000000000000000000, -1.000000000000000000, 0.000000000000000000 ) ) ;
#4686=ORIENTED_EDGE ( 'NONE', *, *, #27186, .F. ) ;
#4694=ORIENTED_EDGE ( 'NONE', *, *, #1294, .F. ) ;
#4695=CARTESIAN_POINT ( 'NONE',  ( 2.789999999999999147, 30.40449935640660684, 2.004522720844263084 ) ) ;
#4697=CARTESIAN_POINT ( 'NONE',  ( 0.02407890056655868569, -17.95514392185398833, -25.38201125280375692 ) ) ;
#4700=CYLINDRICAL_SURFACE ( 'NONE', #7480, 16.19999999999999574 ) ;
#4708=CIRCLE ( 'NONE', #24603, 30.47050528711512030 ) ;
#4710=ORIENTED_EDGE ( 'NONE', *, *, #14205, .F. ) ;
#4712=CARTESIAN_POINT ( 'NONE',  ( 0.006871066268349140978, 23.98851302352036186, 19.42881381898178716 ) ) ;
#4713=B_SPLINE_CURVE_WITH_KNOTS ( 'NONE', 3,
 ( #19285, #21592, #24590, #2540 ),
 .UNSPECIFIED., .F., .F.,
 ( 4, 4 ),
 ( 0.005298347253562320572, 0.005985215922708605162 ),
 .UNSPECIFIED. ) ;
#4716=DIRECTION ( 'NONE',  ( -1.000000000000000000, -0.000000000000000000, -0.000000000000000000 ) ) ;
#4735=ORIENTED_EDGE ( 'NONE', *, *, #30501, .T. ) ;
#4741=CARTESIAN_POINT ( 'NONE',  ( 0.000000000000000000, -3.728217946243090886, 30.24156218513556738 ) ) ;
#4752=EDGE_CURVE ( 'NONE', #22681, #8703, #30675, .T. ) ;
#4761=CYLINDRICAL_SURFACE ( 'NONE', #10882, 2.525000000000001243 ) ;
#4768=ADVANCED_FACE ( 'NONE', ( #30108 ), #31728, .T. ) ;
#4774=LINE ( 'NONE', #5127, #7617 ) ;
#4786=CARTESIAN_POINT ( 'NONE',  ( 1.749999999999999778, -30.28730148581149706, -16.34215476954067015 ) ) ;
#4790=DIRECTION ( 'NONE',  ( -1.000000000000000000, 0.000000000000000000, -0.000000000000000000 ) ) ;
#4791=ORIENTED_EDGE ( 'NONE', *, *, #19067, .T. ) ;
#4795=ORIENTED_EDGE ( 'NONE', *, *, #2849, .F. ) ;
#4799=CARTESIAN_POINT ( 'NONE',  ( 5.127716880498843092E-16, 30.15879770317936348, -5.529954278609071849 ) ) ;
#4800=CARTESIAN_POINT ( 'NONE',  ( 0.1859802911799672831, -32.25918669212988021, -1.206152977788097713 ) ) ;
#4805=ADVANCED_FACE ( 'NONE', ( #19796 ), #30815, .T. ) ;
#4808=DIRECTION ( 'NONE',  ( -1.000000000000000000, -0.000000000000000000, -0.000000000000000000 ) ) ;
#4818=CARTESIAN_POINT ( 'NONE',  ( 0.000000000000000000, 25.67797970382157402, -16.40405592474731833 ) ) ;
#4821=CARTESIAN_POINT ( 'NONE',  ( 0.000000000000000000, 20.79173593595263370, 22.27454621808773538 ) ) ;
#4822=CARTESIAN_POINT ( 'NONE',  ( 0.02407890056655911937, -15.32140196853734970, -27.05343472113007763 ) ) ;
#4824=CARTESIAN_POINT ( 'NONE',  ( 2.789999999999999147, -11.07880054387241664, 29.04985141099759360 ) ) ;
#4825=CARTESIAN_POINT ( 'NONE',  ( -10.00000000000000000, 0.000000000000000000, 0.000000000000000000 ) ) ;
#4830=CARTESIAN_POINT ( 'NONE',  ( 0.02407890056655695096, 26.03801215795542134, -16.98986790278583570 ) ) ;
#4836=EDGE_CURVE ( 'NONE', #23446, #5845, #28346, .T. ) ;
#4842=AXIS2_PLACEMENT_3D ( 'NONE', #1681, #17911, #12549 ) ;
#4845=DIRECTION ( 'NONE',  ( -1.000000000000000000, -0.000000000000000000, 0.000000000000000000 ) ) ;
#4857=AXIS2_PLACEMENT_3D ( 'NONE', #30327, #19488, #16298 ) ;
#4858=EDGE_LOOP ( 'NONE', ( #34273, #30610, #6487, #7399, #16364, #19702 ) ) ;
#4859=ORIENTED_EDGE ( 'NONE', *, *, #31267, .F. ) ;
#4862=ORIENTED_EDGE ( 'NONE', *, *, #14813, .T. ) ;
#4866=CARTESIAN_POINT ( 'NONE',  ( 0.000000000000000000, 0.000000000000000000, 0.000000000000000000 ) ) ;
#4871=DIRECTION ( 'NONE',  ( -1.000000000000000000, -0.000000000000000000, -0.000000000000000000 ) ) ;
#4883=B_SPLINE_CURVE_WITH_KNOTS ( 'NONE', 3,
 ( #30092, #29920, #2683, #27065 ),
 .UNSPECIFIED., .F., .F.,
 ( 4, 4 ),
 ( 4.404817005620765685E-07, 0.001749480761540356689 ),
 .UNSPECIFIED. ) ;
#4897=AXIS2_PLACEMENT_3D ( 'NONE', #13196, #32039, #19070 ) ;
#4898=ORIENTED_EDGE ( 'NONE', *, *, #26687, .T. ) ;
#4901=ORIENTED_EDGE ( 'NONE', *, *, #15315, .T. ) ;
#4904=ORIENTED_EDGE ( 'NONE', *, *, #31270, .F. ) ;
#4909=CARTESIAN_POINT ( 'NONE',  ( 2.783107618804362193, 30.78707849925352136, -2.258378142202823735 ) ) ;
#4911=CARTESIAN_POINT ( 'NONE',  ( 2.790000000000000924, 12.80000000000000071, -3.000000000000000000 ) ) ;
#4918=CIRCLE ( 'NONE', #12320, 2.524999999999999467 ) ;
#4921=FACE_OUTER_BOUND ( 'NONE', #13858, .T. ) ;
#4924=CARTESIAN_POINT ( 'NONE',  ( 2.789999999999999147, 25.67797970382158113, -16.40405592474728635 ) ) ;
#4926=ADVANCED_FACE ( 'NONE', ( #33479 ), #11609, .T. ) ;
#4932=ORIENTED_EDGE ( 'NONE', *, *, #16204, .T. ) ;
#4938=VERTEX_POINT ( 'NONE', #20317 ) ;
#4942=EDGE_LOOP ( 'NONE', ( #21439, #33003, #28983, #33705 ) ) ;
#4945=DIRECTION ( 'NONE',  ( -1.000000000000000000, 0.000000000000000000, 0.000000000000000000 ) ) ;
#4958=DIRECTION ( 'NONE',  ( 0.000000000000000000, 0.000000000000000000, 1.000000000000000000 ) ) ;
#4966=CARTESIAN_POINT ( 'NONE',  ( 2.765921099433443775, -26.45933846664182099, -16.32596387352474565 ) ) ;
#4970=CARTESIAN_POINT ( 'NONE',  ( 0.000000000000000000, -25.83993731729808729, 18.77381338200959604 ) ) ;
#4976=FACE_OUTER_BOUND ( 'NONE', #12978, .T. ) ;
#4980=DIRECTION ( 'NONE',  ( 1.000000000000000000, 0.000000000000000000, 0.000000000000000000 ) ) ;
#4982=AXIS2_PLACEMENT_3D ( 'NONE', #29015, #1965, #34362 ) ;
#4989=DIRECTION ( 'NONE',  ( 0.000000000000000000, 0.000000000000000000, 1.000000000000000000 ) ) ;
#5005=DIRECTION ( 'NONE',  ( -1.000000000000000000, -0.000000000000000000, 0.000000000000000000 ) ) ;
#5014=AXIS2_PLACEMENT_3D ( 'NONE', #20278, #28450, #25774 ) ;
#5018=ADVANCED_FACE ( 'NONE', ( #1782 ), #2299, .F. ) ;
#5023=CARTESIAN_POINT ( 'NONE',  ( 0.000000000000000000, 9.869977788040968036, 30.37666815053940539 ) ) ;
#5032=ORIENTED_EDGE ( 'NONE', *, *, #9390, .F. ) ;
#5039=ORIENTED_EDGE ( 'NONE', *, *, #31322, .T. ) ;
#5047=ORIENTED_EDGE ( 'NONE', *, *, #8835, .F. ) ;
#5049=CARTESIAN_POINT ( 'NONE',  ( 1.040000000000001368, -30.28730148581149706, -16.34215476954066304 ) ) ;
#5051=CARTESIAN_POINT ( 'NONE',  ( 0.006915246992955798207, 27.98916443103565399, -12.86217335695007868 ) ) ;
#5061=CARTESIAN_POINT ( 'NONE',  ( 2.265105943055672810, -17.22577838686547835, -28.59166429730548487 ) ) ;
#5068=ADVANCED_FACE ( 'NONE', ( #26516 ), #15500, .T. ) ;
#5072=AXIS2_PLACEMENT_3D ( 'NONE', #18220, #18395, #18749 ) ;
#5076=EDGE_CURVE ( 'NONE', #18937, #9222, #19645, .T. ) ;
#5077=VERTEX_POINT ( 'NONE', #4966 ) ;
#5085=B_SPLINE_CURVE_WITH_KNOTS ( 'NONE', 3,
 ( #27057, #24020, #24728, #29912, #2492, #7651 ),
 .UNSPECIFIED., .F., .F.,
 ( 4, 2, 4 ),
 ( 4.404817030685402330E-07, 0.001874269627226453306, 0.003748098772749838131 ),
 .UNSPECIFIED. ) ;
#5091=ORIENTED_EDGE ( 'NONE', *, *, #30449, .F. ) ;
#5109=B_SPLINE_CURVE_WITH_KNOTS ( 'NONE', 3,
 ( #4697, #34626, #6853, #34095, #31426, #15592 ),
 .UNSPECIFIED., .F., .F.,
 ( 4, 2, 4 ),
 ( 2.073839991539819829E-07, 0.001873405686414693827, 0.003746603988830233666 ),
 .UNSPECIFIED. ) ;
#5113=ORIENTED_EDGE ( 'NONE', *, *, #3278, .T. ) ;
#5114=EDGE_CURVE ( 'NONE', #7721, #26602, #28390, .T. ) ;
#5127=CARTESIAN_POINT ( 'NONE',  ( 2.789999999999999147, 9.869977788041397915, -27.85166815053926115 ) ) ;
#5130=VERTEX_POINT ( 'NONE', #27396 ) ;
#5137=CARTESIAN_POINT ( 'NONE',  ( 2.033800773663356765, -10.98362253094254726, 32.08736770015211448 ) ) ;
#5140=CARTESIAN_POINT ( 'NONE',  ( 0.7564103416931459156, 5.833445725192799358, 33.41010632092324073 ) ) ;
#5158=VECTOR ( 'NONE', #4685, 1000.000000000000000 ) ;
#5164=ADVANCED_FACE ( 'NONE', ( #16561 ), #32733, .F. ) ;
#5191=DIRECTION ( 'NONE',  ( 0.000000000000000000, 0.000000000000000000, -1.000000000000000000 ) ) ;
#5194=EDGE_CURVE ( 'NONE', #7946, #17530, #13952, .T. ) ;
#5216=AXIS2_PLACEMENT_3D ( 'NONE', #16305, #5229, #32819 ) ;
#5219=ORIENTED_EDGE ( 'NONE', *, *, #28327, .T. ) ;
#5221=CARTESIAN_POINT ( 'NONE',  ( 0.02407890056655608360, -27.96208973699893008, -13.59246946040217630 ) ) ;
#5229=DIRECTION ( 'NONE',  ( -1.000000000000000000, 0.000000000000000000, -0.000000000000000000 ) ) ;
#5239=CARTESIAN_POINT ( 'NONE',  ( 1.040000000000000258, 22.14447232807544452, -26.34405054495532639 ) ) ;
#5245=EDGE_LOOP ( 'NONE', ( #11945, #24399, #34992, #4898, #1637, #15865, #30497, #24758 ) ) ;
#5253=CARTESIAN_POINT ( 'NONE',  ( -5.210000000000000853, 0.000000000000000000, 0.000000000000000000 ) ) ;
#5255=VERTEX_POINT ( 'NONE', #33440 ) ;
#5266=B_SPLINE_CURVE_WITH_KNOTS ( 'NONE', 3,
 ( #33014, #18996, #2947, #11505 ),
 .UNSPECIFIED., .F., .F.,
 ( 4, 4 ),
 ( 0.005298373595863164684, 0.005985241895929849926 ),
 .UNSPECIFIED. ) ;
#5270=CARTESIAN_POINT ( 'NONE',  ( 1.394999999999999574, 6.183021911001842064, 33.85493898757065523 ) ) ;
#5278=CARTESIAN_POINT ( 'NONE',  ( 2.765921099433443331, -3.506335382740311868, -30.89238256715869468 ) ) ;
#5281=CARTESIAN_POINT ( 'NONE',  ( 2.789999999999999147, -0.09145294252698496495, 30.47036804522407749 ) ) ;
#5282=VERTEX_POINT ( 'NONE', #30773 ) ;
#5286=CARTESIAN_POINT ( 'NONE',  ( 2.789999999999999147, 29.94779062842786743, 5.619744560739183825 ) ) ;
#5287=CARTESIAN_POINT ( 'NONE',  ( 2.789999999999999147, -29.68817180695669578, -9.232883799364548949 ) ) ;
#5291=DIRECTION ( 'NONE',  ( -1.000000000000000000, -0.000000000000000000, -0.000000000000000000 ) ) ;
#5309=CARTESIAN_POINT ( 'NONE',  ( 2.789999999999999147, 2.005524111408653720, -31.87689292423236154 ) ) ;
#5322=VERTEX_POINT ( 'NONE', #11923 ) ;
#5333=CARTESIAN_POINT ( 'NONE',  ( 2.789999999999999147, -23.70329957282570632, -20.11932597908854703 ) ) ;
#5334=DIRECTION ( 'NONE',  ( 0.000000000000000000, 0.6845471059286788451, 0.7289686274214207673 ) ) ;
#5337=CARTESIAN_POINT ( 'NONE',  ( 2.790000000000000924, 0.000000000000000000, 0.000000000000000000 ) ) ;
#5352=CARTESIAN_POINT ( 'NONE',  ( 2.789999999999999147, 20.79173593595296055, -22.27454621808740853 ) ) ;
#5354=DIRECTION ( 'NONE',  ( -1.000000000000000000, -0.000000000000000000, -0.000000000000000000 ) ) ;
#5361=CARTESIAN_POINT ( 'NONE',  ( 2.789999999999999147, 23.28319895603611300, -19.33937915510192695 ) ) ;
#5363=ORIENTED_EDGE ( 'NONE', *, *, #25345, .T. ) ;
#5365=CARTESIAN_POINT ( 'NONE',  ( 2.719051659264935417, -30.32005755872691921, 9.230678093032533837 ) ) ;
#5367=CARTESIAN_POINT ( 'NONE',  ( 2.719051683032043254, -15.78353653323396166, 27.48438217453478671 ) ) ;
#5371=CARTESIAN_POINT ( 'NONE',  ( 0.07098932975109609189, 7.308614668456146823, 30.84037831947998143 ) ) ;
#5374=DIRECTION ( 'NONE',  ( 0.000000000000000000, 0.9048270524660234626, -0.4257792915650642773 ) ) ;
#5376=CARTESIAN_POINT ( 'NONE',  ( 1.040000000000000924, 14.89726405156217126, 31.02351007835982344 ) ) ;
#5378=ADVANCED_FACE ( 'NONE', ( #13463 ), #10664, .T. ) ;
#5381=FACE_OUTER_BOUND ( 'NONE', #16709, .T. ) ;
#5383=CYLINDRICAL_SURFACE ( 'NONE', #18473, 34.41491905851385269 ) ;
#5387=ORIENTED_EDGE ( 'NONE', *, *, #10036, .T. ) ;
#5389=VERTEX_POINT ( 'NONE', #5776 ) ;
#5404=CARTESIAN_POINT ( 'NONE',  ( 2.789999999999999147, 23.53611639059710114, 19.35207786518998319 ) ) ;
#5420=FACE_OUTER_BOUND ( 'NONE', #14418, .T. ) ;
#5428=TOROIDAL_SURFACE ( 'NONE', #35006, 30.47050528711512030, 8.000000000000000000 ) ;
#5435=ORIENTED_EDGE ( 'NONE', *, *, #1313, .T. ) ;
#5437=EDGE_CURVE ( 'NONE', #28097, #33936, #14665, .T. ) ;
#5453=CARTESIAN_POINT ( 'NONE',  ( 1.395000000000002238, -30.02688531850407827, 16.81585001935568968 ) ) ;
#5461=VERTEX_POINT ( 'NONE', #16740 ) ;
#5464=DIRECTION ( 'NONE',  ( 0.000000000000000000, 0.000000000000000000, -1.000000000000000000 ) ) ;
#5471=LINE ( 'NONE', #27021, #3709 ) ;
#5472=FACE_OUTER_BOUND ( 'NONE', #11128, .T. ) ;
#5478=CYLINDRICAL_SURFACE ( 'NONE', #17525, 16.19999999999999574 ) ;
#5481=CARTESIAN_POINT ( 'NONE',  ( 2.765921099433443331, 14.63235270440974922, -27.43224275967423509 ) ) ;
#5484=EDGE_LOOP ( 'NONE', ( #9410, #876, #3181, #34065, #28483, #23898 ) ) ;
#5487=AXIS2_PLACEMENT_3D ( 'NONE', #27970, #19804, #14107 ) ;
#5490=CARTESIAN_POINT ( 'NONE',  ( 1.749999999999999778, -10.37741591188916424, 32.81304455236865181 ) ) ;
#5501=ORIENTED_EDGE ( 'NONE', *, *, #11064, .T. ) ;
#5503=CARTESIAN_POINT ( 'NONE',  ( 8.000000000000000000, 0.000000000000000000, 0.000000000000000000 ) ) ;
#5505=CARTESIAN_POINT ( 'NONE',  ( 2.789999999999999147, 27.60935207499552035, 12.89090262359662731 ) ) ;
#5506=CARTESIAN_POINT ( 'NONE',  ( 0.02407890056655825201, -17.95514392185434360, 25.38201125280350468 ) ) ;
#5512=VERTEX_POINT ( 'NONE', #22000 ) ;
#5522=CARTESIAN_POINT ( 'NONE',  ( 2.765921099433441110, -17.95514392185398833, -25.38201125280375692 ) ) ;
#5537=CARTESIAN_POINT ( 'NONE',  ( 2.765921099433443331, -29.68817180695682723, 9.232883799364120847 ) ) ;
#5538=DIRECTION ( 'NONE',  ( 0.000000000000000000, 0.000000000000000000, -1.000000000000000000 ) ) ;
#5539=CARTESIAN_POINT ( 'NONE',  ( 1.040000000000000480, -10.89151784028265979, -32.64600270996228204 ) ) ;
#5548=DIRECTION ( 'NONE',  ( -1.000000000000000000, 0.000000000000000000, -0.000000000000000000 ) ) ;
#5552=ADVANCED_FACE ( 'NONE', ( #23077 ), #22725, .T. ) ;
#5560=ORIENTED_EDGE ( 'NONE', *, *, #30163, .T. ) ;
#5561=EDGE_LOOP ( 'NONE', ( #16389, #21797, #33200, #25822, #29105, #1669 ) ) ;
#5564=CIRCLE ( 'NONE', #30034, 30.47050528711511674 ) ;
#5566=DIRECTION ( 'NONE',  ( 0.000000000000000000, 0.000000000000000000, 1.000000000000000000 ) ) ;
#5572=EDGE_CURVE ( 'NONE', #16565, #31475, #28582, .T. ) ;
#5579=CARTESIAN_POINT ( 'NONE',  ( 1.039999999999999813, -30.02688531850407117, 16.81585001935569323 ) ) ;
#5588=ORIENTED_EDGE ( 'NONE', *, *, #32376, .T. ) ;
#5590=CARTESIAN_POINT ( 'NONE',  ( 0.5288002523874972827, 21.87231946537524152, -25.22857168675658812 ) ) ;
#5592=CIRCLE ( 'NONE', #15308, 30.47050528711511674 ) ;
#5612=ORIENTED_EDGE ( 'NONE', *, *, #19594, .T. ) ;
#5622=CARTESIAN_POINT ( 'NONE',  ( 2.789999999999999147, -8.813854705727257155, -29.13568936554952060 ) ) ;
#5629=VERTEX_POINT ( 'NONE', #20404 ) ;
#5638=DIRECTION ( 'NONE',  ( 0.000000000000000000, 0.000000000000000000, 1.000000000000000000 ) ) ;
#5640=ORIENTED_EDGE ( 'NONE', *, *, #13661, .T. ) ;
#5642=ORIENTED_EDGE ( 'NONE', *, *, #23617, .T. ) ;
#5646=CARTESIAN_POINT ( 'NONE',  ( 0.7561992215529863559, 27.12277411069277377, -20.36158770325022260 ) ) ;
#5660=ORIENTED_EDGE ( 'NONE', *, *, #4044, .F. ) ;
#5666=EDGE_LOOP ( 'NONE', ( #10450, #18151, #22236, #1603 ) ) ;
#5676=CARTESIAN_POINT ( 'NONE',  ( 1.749999999999999778, -2.430610048906265419, 34.32897884578299852 ) ) ;
#5692=CARTESIAN_POINT ( 'NONE',  ( 0.000000000000000000, 0.000000000000000000, 0.000000000000000000 ) ) ;
#5695=DIRECTION ( 'NONE',  ( -1.000000000000000000, 0.000000000000000000, 0.000000000000000000 ) ) ;
#5701=EDGE_CURVE ( 'NONE', #15650, #26161, #31757, .T. ) ;
#5702=CARTESIAN_POINT ( 'NONE',  ( 0.7564103365129547507, 13.95893286369010688, 30.90974742850075074 ) ) ;
#5705=ORIENTED_EDGE ( 'NONE', *, *, #16115, .F. ) ;
#5712=CARTESIAN_POINT ( 'NONE',  ( 1.040000000000002034, 6.714005886384948774, 33.75364837705175347 ) ) ;
#5714=DIRECTION ( 'NONE',  ( 0.000000000000000000, 0.000000000000000000, 1.000000000000000000 ) ) ;
#5715=EDGE_CURVE ( 'NONE', #34278, #5461, #21192, .T. ) ;
#5719=CARTESIAN_POINT ( 'NONE',  ( 0.02407890056655521624, 28.29688452313399338, 12.88099432405614309 ) ) ;
#5723=ORIENTED_EDGE ( 'NONE', *, *, #23863, .F. ) ;
#5731=EDGE_LOOP ( 'NONE', ( #22281, #16856, #9079, #7898, #23020, #2800 ) ) ;
#5743=LINE ( 'NONE', #8261, #17111 ) ;
#5769=DIRECTION ( 'NONE',  ( 0.000000000000000000, 0.000000000000000000, 1.000000000000000000 ) ) ;
#5774=CIRCLE ( 'NONE', #17209, 34.41491905851385269 ) ;
#5776=CARTESIAN_POINT ( 'NONE',  ( 1.749999999999999778, -18.66807150955433769, 28.91175816027496381 ) ) ;
#5783=CARTESIAN_POINT ( 'NONE',  ( 2.033800782743256708, -24.35691930005240735, -23.60041548268739220 ) ) ;
#5785=VERTEX_POINT ( 'NONE', #29094 ) ;
#5801=B_SPLINE_CURVE_WITH_KNOTS ( 'NONE', 3,
 ( #23975, #34859, #10467, #21323 ),
 .UNSPECIFIED., .F., .F.,
 ( 4, 4 ),
 ( 4.077050493238099252E-07, 0.0006881451559005025012 ),
 .UNSPECIFIED. ) ;
#5807=EDGE_CURVE ( 'NONE', #701, #30793, #816, .T. ) ;
#5814=LINE ( 'NONE', #2631, #20020 ) ;
#5815=DIRECTION ( 'NONE',  ( -1.000000000000000000, 0.000000000000000000, 0.000000000000000000 ) ) ;
#5819=DIRECTION ( 'NONE',  ( 0.000000000000000000, 0.9510565162951500895, 0.3090169943749579984 ) ) ;
#5829=EDGE_LOOP ( 'NONE', ( #13908, #12301, #9272, #28673 ) ) ;
#5830=VERTEX_POINT ( 'NONE', #25099 ) ;
#5831=AXIS2_PLACEMENT_3D ( 'NONE', #17235, #17754, #15078 ) ;
#5833=CARTESIAN_POINT ( 'NONE',  ( 0.000000000000000000, -29.00730259674847034, 9.328884633908835156 ) ) ;
#5840=CYLINDRICAL_SURFACE ( 'NONE', #19166, 34.41491905851385269 ) ;
#5845=VERTEX_POINT ( 'NONE', #3040 ) ;
#5847=AXIS2_PLACEMENT_3D ( 'NONE', #34236, #4845, #34761 ) ;
#5851=CARTESIAN_POINT ( 'NONE',  ( 1.749999999999999778, 0.000000000000000000, 0.000000000000000000 ) ) ;
#5855=CIRCLE ( 'NONE', #17811, 2.524999999999999467 ) ;
#5859=DIRECTION ( 'NONE',  ( 0.000000000000000000, 0.000000000000000000, 1.000000000000000000 ) ) ;
#5862=EDGE_LOOP ( 'NONE', ( #22382, #29696, #13327, #14311 ) ) ;
#5866=CARTESIAN_POINT ( 'NONE',  ( 1.040000000000000702, -10.89151784028311809, 32.64600270996213283 ) ) ;
#5872=EDGE_CURVE ( 'NONE', #11863, #13812, #32632, .T. ) ;
#5877=CARTESIAN_POINT ( 'NONE',  ( 2.033589656796778833, -18.61839266759088929, -28.34818773854082963 ) ) ;
#5878=CIRCLE ( 'NONE', #26900, 2.525000000000000799 ) ;
#5884=DIRECTION ( 'NONE',  ( -1.000000000000000000, -0.000000000000000000, -0.000000000000000000 ) ) ;
#5889=DIRECTION ( 'NONE',  ( -1.000000000000000000, -0.000000000000000000, -0.000000000000000000 ) ) ;
#5895=DIRECTION ( 'NONE',  ( 0.000000000000000000, 0.000000000000000000, 1.000000000000000000 ) ) ;
#5899=EDGE_CURVE ( 'NONE', #33010, #5389, #3728, .T. ) ;
#5907=AXIS2_PLACEMENT_3D ( 'NONE', #27188, #23822, #29870 ) ;
#5909=ORIENTED_EDGE ( 'NONE', *, *, #25026, .T. ) ;
#5916=EDGE_CURVE ( 'NONE', #19893, #22114, #19617, .T. ) ;
#5919=B_SPLINE_CURVE_WITH_KNOTS ( 'NONE', 3,
 ( #30819, #29151, #14463, #33657, #925, #20795 ),
 .UNSPECIFIED., .F., .F.,
 ( 4, 2, 4 ),
 ( 4.404817078296468374E-07, 0.001874269662699937699, 0.003748098843692045969 ),
 .UNSPECIFIED. ) ;
#5920=FACE_OUTER_BOUND ( 'NONE', #13160, .T. ) ;
#5921=DIRECTION ( 'NONE',  ( -1.000000000000000000, -0.000000000000000000, -0.000000000000000000 ) ) ;
#5948=CARTESIAN_POINT ( 'NONE',  ( 2.783107553646922305, -30.82736387488650820, -1.618073722873514697 ) ) ;
#5951=EDGE_LOOP ( 'NONE', ( #30208, #21601, #14843, #18773, #29079, #1297 ) ) ;
#5954=ORIENTED_EDGE ( 'NONE', *, *, #29830, .T. ) ;
#5970=CARTESIAN_POINT ( 'NONE',  ( 0.000000000000000000, 0.000000000000000000, 0.000000000000000000 ) ) ;
#5980=FACE_OUTER_BOUND ( 'NONE', #13419, .T. ) ;
#5984=B_SPLINE_CURVE_WITH_KNOTS ( 'NONE', 3,
 ( #1792, #6949, #17843, #3766 ),
 .UNSPECIFIED., .F., .F.,
 ( 4, 4 ),
 ( 0.005298349496164106269, 0.005985218188604198714 ),
 .UNSPECIFIED. ) ;
#5992=CARTESIAN_POINT ( 'NONE',  ( 1.395000000000002238, -1.891117961020238436, 34.36292081097831641 ) ) ;
#5996=AXIS2_PLACEMENT_3D ( 'NONE', #14680, #1135, #12000 ) ;
#6001=CARTESIAN_POINT ( 'NONE',  ( 0.1859802741905670354, -24.34160354263086035, 21.20368514569409513 ) ) ;
#6003=DIRECTION ( 'NONE',  ( 0.000000000000000000, 0.000000000000000000, -1.000000000000000000 ) ) ;
#6006=ORIENTED_EDGE ( 'NONE', *, *, #16687, .T. ) ;
#6008=VERTEX_POINT ( 'NONE', #33830 ) ;
#6020=ORIENTED_EDGE ( 'NONE', *, *, #9348, .T. ) ;
#6024=ORIENTED_EDGE ( 'NONE', *, *, #30619, .T. ) ;
#6033=DIRECTION ( 'NONE',  ( 0.000000000000000000, 0.000000000000000000, 1.000000000000000000 ) ) ;
#6036=CARTESIAN_POINT ( 'NONE',  ( 2.765921099433442443, 29.44518845714779332, -9.980709654879110104 ) ) ;
#6076=UNCERTAINTY_MEASURE_WITH_UNIT (LENGTH_MEASURE( 1.000000000000000082E-05 ), #14562, 'distance_accuracy_value', 'NONE');
#6078=ORIENTED_EDGE ( 'NONE', *, *, #15449, .T. ) ;
#6083=EDGE_CURVE ( 'NONE', #34030, #8526, #17824, .T. ) ;
#6086=EDGE_CURVE ( 'NONE', #4938, #1226, #6225, .T. ) ;
#6087=ORIENTED_EDGE ( 'NONE', *, *, #6218, .T. ) ;
#6098=CYLINDRICAL_SURFACE ( 'NONE', #18648, 2.524999999999999467 ) ;
#6109=AXIS2_PLACEMENT_3D ( 'NONE', #26033, #10013, #23026 ) ;
#6119=DIRECTION ( 'NONE',  ( 0.000000000000000000, 0.000000000000000000, 1.000000000000000000 ) ) ;
#6121=LINE ( 'NONE', #5287, #19000 ) ;
#6122=DIRECTION ( 'NONE',  ( -1.000000000000000000, -0.000000000000000000, -0.000000000000000000 ) ) ;
#6130=EDGE_LOOP ( 'NONE', ( #487, #2381, #33524, #1051, #34952, #25371 ) ) ;
#6132=ADVANCED_FACE ( 'NONE', ( #15680 ), #2825, .F. ) ;
#6139=AXIS2_PLACEMENT_3D ( 'NONE', #28319, #3914, #11602 ) ;
#6140=DIRECTION ( 'NONE',  ( 0.000000000000000000, 0.000000000000000000, 1.000000000000000000 ) ) ;
#6141=CARTESIAN_POINT ( 'NONE',  ( 0.002098586324980263994, 27.86175707474580321, -12.86217335695010533 ) ) ;
#6143=ORIENTED_EDGE ( 'NONE', *, *, #30049, .F. ) ;
#6158=CARTESIAN_POINT ( 'NONE',  ( 2.789999999999999147, -11.07880054387200985, -29.04985141099774637 ) ) ;
#6179=B_SPLINE_CURVE_WITH_KNOTS ( 'NONE', 3,
 ( #18835, #32866, #27530, #24853 ),
 .UNSPECIFIED., .F., .F.,
 ( 4, 4 ),
 ( 4.608367445541797598E-07, 0.0006881987313283725351 ),
 .UNSPECIFIED. ) ;
#6189=CARTESIAN_POINT ( 'NONE',  ( -5.210000000000000853, 0.000000000000000000, 0.000000000000000000 ) ) ;
#6190=ORIENTED_EDGE ( 'NONE', *, *, #7737, .T. ) ;
#6192=DIRECTION ( 'NONE',  ( -1.000000000000000000, -0.000000000000000000, -0.000000000000000000 ) ) ;
#6206=AXIS2_PLACEMENT_3D ( 'NONE', #23593, #26430, #12569 ) ;
#6217=ORIENTED_EDGE ( 'NONE', *, *, #22597, .T. ) ;
#6218=EDGE_CURVE ( 'NONE', #11399, #12523, #32102, .T. ) ;
#6225=B_SPLINE_CURVE_WITH_KNOTS ( 'NONE', 3,
 ( #1773, #18177, #20479, #29003, #15494, #34526 ),
 .UNSPECIFIED., .F., .F.,
 ( 4, 2, 4 ),
 ( 2.120780580243931197E-07, 0.001873410385593401008, 0.003746608693128777694 ),
 .UNSPECIFIED. ) ;
#6227=DIRECTION ( 'NONE',  ( 0.000000000000000000, 0.000000000000000000, 1.000000000000000000 ) ) ;
#6228=ORIENTED_EDGE ( 'NONE', *, *, #11773, .T. ) ;
#6234=ORIENTED_EDGE ( 'NONE', *, *, #12997, .F. ) ;
#6239=VERTEX_POINT ( 'NONE', #5490 ) ;
#6240=CARTESIAN_POINT ( 'NONE',  ( 1.040000000000000924, 0.000000000000000000, 0.000000000000000000 ) ) ;
#6247=ORIENTED_EDGE ( 'NONE', *, *, #14778, .F. ) ;
#6252=TOROIDAL_SURFACE ( 'NONE', #33532, 30.47050528711511674, 8.000000000000000000 ) ;
#6257=VERTEX_POINT ( 'NONE', #30597 ) ;
#6260=DIRECTION ( 'NONE',  ( 1.000000000000000000, 0.000000000000000000, 0.000000000000000000 ) ) ;
#6271=CARTESIAN_POINT ( 'NONE',  ( 2.765921099433442887, -26.45933846664205902, 16.32596387352436551 ) ) ;
#6281=ADVANCED_FACE ( 'NONE', ( #17083 ), #27916, .T. ) ;
#6294=CYLINDRICAL_SURFACE ( 'NONE', #28637, 16.19999999999999574 ) ;
#6299=EDGE_CURVE ( 'NONE', #21605, #12335, #31338, .T. ) ;
#6306=VERTEX_POINT ( 'NONE', #11207 ) ;
#6308=ORIENTED_EDGE ( 'NONE', *, *, #23622, .F. ) ;
#6315=CARTESIAN_POINT ( 'NONE',  ( 1.040000000000002034, 28.00026196654299326, -20.00929742917092824 ) ) ;
#6327=EDGE_CURVE ( 'NONE', #11423, #31622, #9388, .T. ) ;
#6328=CARTESIAN_POINT ( 'NONE',  ( -10.00000000000000000, 0.000000000000000000, 0.000000000000000000 ) ) ;
#6343=VECTOR ( 'NONE', #10831, 1000.000000000000000 ) ;
#6345=VERTEX_POINT ( 'NONE', #1049 ) ;
#6347=CARTESIAN_POINT ( 'NONE',  ( 0.02407890056655695096, -8.112136323389137260, 30.01377904834206589 ) ) ;
#6348=AXIS2_PLACEMENT_3D ( 'NONE', #6189, #17450, #12274 ) ;
#6355=EDGE_CURVE ( 'NONE', #21781, #13694, #16482, .T. ) ;
#6359=DIRECTION ( 'NONE',  ( -1.000000000000000000, -0.000000000000000000, -0.000000000000000000 ) ) ;
#6363=ORIENTED_EDGE ( 'NONE', *, *, #18028, .F. ) ;
#6367=LINE ( 'NONE', #3872, #10304 ) ;
#6373=VERTEX_POINT ( 'NONE', #26122 ) ;
#6390=DIRECTION ( 'NONE',  ( -1.000000000000000000, -0.000000000000000000, -0.000000000000000000 ) ) ;
#6391=CARTESIAN_POINT ( 'NONE',  ( 1.040000000000001590, -33.26546734453813059, -8.820166447042128155 ) ) ;
#6394=ORIENTED_EDGE ( 'NONE', *, *, #2611, .T. ) ;
#6398=VERTEX_POINT ( 'NONE', #28623 ) ;
#6400=CARTESIAN_POINT ( 'NONE',  ( 2.719010730813550047, 12.21472555652470326, 29.24628546289466868 ) ) ;
#6408=EDGE_LOOP ( 'NONE', ( #2110, #32877, #26075, #21112 ) ) ;
#6421=AXIS2_PLACEMENT_3D ( 'NONE', #22118, #29595, #21936 ) ;
#6430=FACE_OUTER_BOUND ( 'NONE', #21986, .T. ) ;
#6431=ORIENTED_EDGE ( 'NONE', *, *, #30379, .F. ) ;
#6432=DIRECTION ( 'NONE',  ( 0.000000000000000000, 0.000000000000000000, 1.000000000000000000 ) ) ;
#6434=VECTOR ( 'NONE', #29766, 1000.000000000000000 ) ;
#6443=ORIENTED_EDGE ( 'NONE', *, *, #24356, .F. ) ;
#6466=ORIENTED_EDGE ( 'NONE', *, *, #8929, .T. ) ;
#6474=CIRCLE ( 'NONE', #34328, 2.525000000000000355 ) ;
#6478=DIRECTION ( 'NONE',  ( -1.000000000000000000, 0.000000000000000000, -0.000000000000000000 ) ) ;
#6487=ORIENTED_EDGE ( 'NONE', *, *, #23617, .F. ) ;
#6496=CARTESIAN_POINT ( 'NONE',  ( 2.789999999999999147, 13.51972826729810961, 27.27250221666296071 ) ) ;
#6500=AXIS2_PLACEMENT_3D ( 'NONE', #18556, #1797, #31690 ) ;
#6506=CARTESIAN_POINT ( 'NONE',  ( 2.789999999999999147, -30.43331811787860275, -0.6209492052235439097 ) ) ;
#6509=EDGE_CURVE ( 'NONE', #34482, #30531, #17306, .T. ) ;
#6510=CARTESIAN_POINT ( 'NONE',  ( 2.789999999999999147, 28.29688452313417812, -12.88099432405573630 ) ) ;
#6512=B_SPLINE_CURVE_WITH_KNOTS ( 'NONE', 3,
 ( #4517, #26952, #21442, #34443 ),
 .UNSPECIFIED., .F., .F.,
 ( 4, 4 ),
 ( 0.005298346188946806770, 0.005985214897255182465 ),
 .UNSPECIFIED. ) ;
#6513=CARTESIAN_POINT ( 'NONE',  ( 0.02407890056655695096, 30.61125888652961891, 5.439165181699118889 ) ) ;
#6536=DIRECTION ( 'NONE',  ( -1.000000000000000000, 0.000000000000000000, 0.000000000000000000 ) ) ;
#6538=LINE ( 'NONE', #17437, #3638 ) ;
#6539=EDGE_CURVE ( 'NONE', #10340, #7014, #34372, .T. ) ;
#6546=ORIENTED_EDGE ( 'NONE', *, *, #15233, .F. ) ;
#6562=CARTESIAN_POINT ( 'NONE',  ( 8.000000000000000000, 0.000000000000000000, 0.000000000000000000 ) ) ;
#6564=CARTESIAN_POINT ( 'NONE',  ( 2.719010706573971703, -24.04031276246385929, 20.65449384219750684 ) ) ;
#6581=LINE ( 'NONE', #33463, #15254 ) ;
#6582=CARTESIAN_POINT ( 'NONE',  ( 1.749999999999999778, 0.000000000000000000, 0.000000000000000000 ) ) ;
#6583=ORIENTED_EDGE ( 'NONE', *, *, #14966, .F. ) ;
#6584=DIRECTION ( 'NONE',  ( 0.000000000000000000, 0.000000000000000000, 1.000000000000000000 ) ) ;
#6593=CIRCLE ( 'NONE', #919, 2.524999999999999911 ) ;
#6597=CARTESIAN_POINT ( 'NONE',  ( 2.719051674741964852, 29.95509811880031492, 10.35390711157494081 ) ) ;
#6603=CARTESIAN_POINT ( 'NONE',  ( 0.1835381450695051930, 32.14582644238494424, 2.841494734165256109 ) ) ;
#6606=CARTESIAN_POINT ( 'NONE',  ( 0.7561992064972459238, 13.95859842408671447, -30.90949138205555968 ) ) ;
#6607=CARTESIAN_POINT ( 'NONE',  ( 2.715598927533382057, 28.97026656347592777, 12.96367524219944833 ) ) ;
#6608=ORIENTED_EDGE ( 'NONE', *, *, #3397, .T. ) ;
#6613=ADVANCED_FACE ( 'NONE', ( #4921 ), #15986, .T. ) ;
#6616=ORIENTED_EDGE ( 'NONE', *, *, #23864, .F. ) ;
#6627=ORIENTED_EDGE ( 'NONE', *, *, #14795, .T. ) ;
#6652=DIRECTION ( 'NONE',  ( -1.000000000000000000, -0.000000000000000000, 0.000000000000000000 ) ) ;
#6655=FACE_OUTER_BOUND ( 'NONE', #20955, .T. ) ;
#6656=DIRECTION ( 'NONE',  ( -1.000000000000000000, -0.000000000000000000, -0.000000000000000000 ) ) ;
#6661=EDGE_CURVE ( 'NONE', #9347, #14830, #29142, .T. ) ;
#6673=ADVANCED_FACE ( 'NONE', ( #12964 ), #4251, .T. ) ;
#6675=CARTESIAN_POINT ( 'NONE',  ( 2.261199747612499422, 21.87231946537488270, 25.22857168675692563 ) ) ;
#6677=CARTESIAN_POINT ( 'NONE',  ( 0.02407890056655695096, 30.61125888652969707, -5.439165181698684570 ) ) ;
#6688=ORIENTED_EDGE ( 'NONE', *, *, #23302, .T. ) ;
#6701=CARTESIAN_POINT ( 'NONE',  ( 0.02407890056655695096, -21.56796757982795043, -22.39322359481629476 ) ) ;
#6703=CARTESIAN_POINT ( 'NONE',  ( 2.789999999999999147, 29.44518845714764765, 9.980709654879525772 ) ) ;
#6707=ADVANCED_FACE ( 'NONE', ( #17229 ), #32685, .T. ) ;
#6709=DIRECTION ( 'NONE',  ( 0.000000000000000000, 0.000000000000000000, 1.000000000000000000 ) ) ;
#6710=ORIENTED_EDGE ( 'NONE', *, *, #19615, .T. ) ;
#6722=ADVANCED_FACE ( 'NONE', ( #27873 ), #17050, .T. ) ;
#6739=EDGE_LOOP ( 'NONE', ( #1477, #6443, #9689, #18085 ) ) ;
#6744=VECTOR ( 'NONE', #24515, 1000.000000000000000 ) ;
#6749=VERTEX_POINT ( 'NONE', #9019 ) ;
#6752=EDGE_CURVE ( 'NONE', #27456, #32641, #655, .T. ) ;
#6757=CIRCLE ( 'NONE', #15887, 30.47050528711511674 ) ;
#6758=DIRECTION ( 'NONE',  ( -1.000000000000000000, 0.000000000000000000, 0.000000000000000000 ) ) ;
#6770=ORIENTED_EDGE ( 'NONE', *, *, #25841, .T. ) ;
#6775=ORIENTED_EDGE ( 'NONE', *, *, #22145, .T. ) ;
#6793=CARTESIAN_POINT ( 'NONE',  ( 0.000000000000000000, 17.98401995359632011, 24.59729088254965035 ) ) ;
#6800=EDGE_LOOP ( 'NONE', ( #824, #27580, #34472, #3677, #29955, #10962 ) ) ;
#6807=ADVANCED_FACE ( 'NONE', ( #27341 ), #14528, .T. ) ;
#6815=EDGE_CURVE ( 'NONE', #13866, #2454, #31276, .T. ) ;
#6816=B_SPLINE_CURVE_WITH_KNOTS ( 'NONE', 3,
 ( #30477, #27449, #8572, #220, #32780, #5539 ),
 .UNSPECIFIED., .F., .F.,
 ( 4, 2, 4 ),
 ( 1.978042196653065176E-07, 0.001873396096185922770, 0.003746594388152190303 ),
 .UNSPECIFIED. ) ;
#6818=ORIENTED_EDGE ( 'NONE', *, *, #24185, .T. ) ;
#6822=CARTESIAN_POINT ( 'NONE',  ( 0.02407890056655695096, 20.99477179376825120, 22.93149026599753526 ) ) ;
#6825=CARTESIAN_POINT ( 'NONE',  ( 1.394999999999999574, -24.90160365674885057, 23.75493189058332533 ) ) ;
#6846=DIRECTION ( 'NONE',  ( -1.000000000000000000, -0.000000000000000000, -0.000000000000000000 ) ) ;
#6847=CARTESIAN_POINT ( 'NONE',  ( 8.000000000000000000, 0.000000000000000000, 0.000000000000000000 ) ) ;
#6853=CARTESIAN_POINT ( 'NONE',  ( 0.1835381660689911765, -18.30111164264862111, -26.58002197185247439 ) ) ;
#6854=VERTEX_POINT ( 'NONE', #1702 ) ;
#6857=CARTESIAN_POINT ( 'NONE',  ( 2.719051659378652896, -11.11627562454391338, -29.68062877649334652 ) ) ;
#6858=CARTESIAN_POINT ( 'NONE',  ( 0.7561992259563318219, 31.33438324387140383, -12.97673134914391824 ) ) ;
#6862=ORIENTED_EDGE ( 'NONE', *, *, #16343, .T. ) ;
#6869=VERTEX_POINT ( 'NONE', #11881 ) ;
#6871=CARTESIAN_POINT ( 'NONE',  ( 2.790000000000080416, -14.96425809615007907, 26.76330950827329147 ) ) ;
#6878=VERTEX_POINT ( 'NONE', #28238 ) ;
#6883=DIRECTION ( 'NONE',  ( -1.000000000000000000, -0.000000000000000000, -0.000000000000000000 ) ) ;
#6884=EDGE_LOOP ( 'NONE', ( #7265, #19306, #12856, #30916 ) ) ;
#6886=VERTEX_POINT ( 'NONE', #14552 ) ;
#6887=AXIS2_PLACEMENT_3D ( 'NONE', #26909, #8039, #30110 ) ;
#6896=ORIENTED_EDGE ( 'NONE', *, *, #1922, .F. ) ;
#6900=CARTESIAN_POINT ( 'NONE',  ( 1.040000000000002034, 32.09669216789253454, -12.41728656686340315 ) ) ;
#6909=CARTESIAN_POINT ( 'NONE',  ( 2.765921099433441999, -23.70329957282570632, -20.11932597908854703 ) ) ;
#6914=ORIENTED_EDGE ( 'NONE', *, *, #27258, .T. ) ;
#6915=EDGE_CURVE ( 'NONE', #5282, #23190, #11753, .T. ) ;
#6932=B_SPLINE_CURVE_WITH_KNOTS ( 'NONE', 3,
 ( #2191, #26572, #7169, #31564, #13241, #12535 ),
 .UNSPECIFIED., .F., .F.,
 ( 4, 2, 4 ),
 ( 4.404817046727483726E-07, 0.001874269636018133147, 0.003748098790331593627 ),
 .UNSPECIFIED. ) ;
#6934=DIRECTION ( 'NONE',  ( 0.000000000000000000, 0.000000000000000000, 1.000000000000000000 ) ) ;
#6946=CARTESIAN_POINT ( 'NONE',  ( 1.394999999999999574, 34.17636915695680244, 4.045051921974837761 ) ) ;
#6949=CARTESIAN_POINT ( 'NONE',  ( 2.789999999999999147, -7.837340408379732892, -29.64303704467405964 ) ) ;
#6951=VECTOR ( 'NONE', #536, 1000.000000000000000 ) ;
#6966=CYLINDRICAL_SURFACE ( 'NONE', #28413, 16.19999999999999574 ) ;
#6975=DIRECTION ( 'NONE',  ( -1.000000000000000000, 0.000000000000000000, 0.000000000000000000 ) ) ;
#6976=AXIS2_PLACEMENT_3D ( 'NONE', #24494, #10991, #30037 ) ;
#6987=ORIENTED_EDGE ( 'NONE', *, *, #2036, .T. ) ;
#6989=FACE_OUTER_BOUND ( 'NONE', #8560, .T. ) ;
#6994=FACE_OUTER_BOUND ( 'NONE', #13567, .T. ) ;
#6998=AXIS2_PLACEMENT_3D ( 'NONE', #21794, #16656, #26964 ) ;
#7002=DIRECTION ( 'NONE',  ( 0.000000000000000000, 0.000000000000000000, 1.000000000000000000 ) ) ;
#7006=AXIS2_PLACEMENT_3D ( 'NONE', #13194, #32559, #184 ) ;
#7008=ORIENTED_EDGE ( 'NONE', *, *, #13779, .T. ) ;
#7010=ADVANCED_FACE ( 'NONE', ( #20919 ), #7374, .F. ) ;
#7014=VERTEX_POINT ( 'NONE', #4695 ) ;
#7021=CARTESIAN_POINT ( 'NONE',  ( 0.000000000000000000, 0.000000000000000000, 0.000000000000000000 ) ) ;
#7032=ORIENTED_EDGE ( 'NONE', *, *, #15211, .F. ) ;
#7034=CARTESIAN_POINT ( 'NONE',  ( 0.02407890056655868569, -8.112136323388726922, -30.01377904834218668 ) ) ;
#7049=AXIS2_PLACEMENT_3D ( 'NONE', #17930, #1869, #15418 ) ;
#7074=AXIS2_PLACEMENT_3D ( 'NONE', #3067, #27214, #19050 ) ;
#7077=ORIENTED_EDGE ( 'NONE', *, *, #23302, .F. ) ;
#7078=CIRCLE ( 'NONE', #1409, 2.524999999999999467 ) ;
#7079=AXIS2_PLACEMENT_3D ( 'NONE', #10524, #2674, #11228 ) ;
#7089=VERTEX_POINT ( 'NONE', #10409 ) ;
#7104=DIRECTION ( 'NONE',  ( 0.000000000000000000, 0.9822872507286906085, -0.1873813145857145812 ) ) ;
#7105=AXIS2_PLACEMENT_3D ( 'NONE', #25164, #8801, #27665 ) ;
#7113=CARTESIAN_POINT ( 'NONE',  ( 2.261199756163084551, 20.68324032934681966, -26.21226347405724155 ) ) ;
#7114=CARTESIAN_POINT ( 'NONE',  ( 2.789999999999999147, 23.28319895603611300, -21.86437915510192909 ) ) ;
#7115=VERTEX_POINT ( 'NONE', #12749 ) ;
#7118=ORIENTED_EDGE ( 'NONE', *, *, #24948, .F. ) ;
#7121=DIRECTION ( 'NONE',  ( 1.000000000000000000, -0.000000000000000000, -0.000000000000000000 ) ) ;
#7123=CARTESIAN_POINT ( 'NONE',  ( 2.606461801040218074, 31.84255742294090652, 5.242117949250861386 ) ) ;
#7166=FACE_OUTER_BOUND ( 'NONE', #18705, .T. ) ;
#7169=CARTESIAN_POINT ( 'NONE',  ( 2.261199745677082262, 26.55216317045652730, -20.24504431679611116 ) ) ;
#7175=ADVANCED_FACE ( 'NONE', ( #11656 ), #22507, .F. ) ;
#7179=VERTEX_POINT ( 'NONE', #24806 ) ;
#7183=CARTESIAN_POINT ( 'NONE',  ( 0.02407890056655825201, -17.95514392185434360, 25.38201125280350468 ) ) ;
#7184=ORIENTED_EDGE ( 'NONE', *, *, #24341, .T. ) ;
#7193=VERTEX_POINT ( 'NONE', #14330 ) ;
#7198=CARTESIAN_POINT ( 'NONE',  ( 0.02407890056655738464, -27.96208973699912548, 13.59246946040177129 ) ) ;
#7206=CARTESIAN_POINT ( 'NONE',  ( 2.783128773493238395, -7.987145637396467990, 29.81833655972095087 ) ) ;
#7214=CARTESIAN_POINT ( 'NONE',  ( 1.394999999999999574, -18.21166265554768415, -29.20140402659759715 ) ) ;
#7234=ORIENTED_EDGE ( 'NONE', *, *, #15256, .F. ) ;
#7235=ORIENTED_EDGE ( 'NONE', *, *, #21337, .F. ) ;
#7239=DIRECTION ( 'NONE',  ( -1.000000000000000000, -0.000000000000000000, -0.000000000000000000 ) ) ;
#7241=VECTOR ( 'NONE', #13229, 1000.000000000000000 ) ;
#7244=CARTESIAN_POINT ( 'NONE',  ( 0.006871144406695839368, -27.79352918700758934, 13.43306967213398906 ) ) ;
#7253=VERTEX_POINT ( 'NONE', #24977 ) ;
#7258=CARTESIAN_POINT ( 'NONE',  ( 0.1859802529459479992, -16.26694784591012777, -27.88362116434760551 ) ) ;
#7260=CARTESIAN_POINT ( 'NONE',  ( 50.00050000000000239, 0.000000000000000000, 3.000000000000000000 ) ) ;
#7261=CARTESIAN_POINT ( 'NONE',  ( 2.765921099433441110, 14.63235270440936731, 27.43224275967444470 ) ) ;
#7262=DIRECTION ( 'NONE',  ( -1.000000000000000000, 0.000000000000000000, 0.000000000000000000 ) ) ;
#7265=ORIENTED_EDGE ( 'NONE', *, *, #17058, .T. ) ;
#7267=VERTEX_POINT ( 'NONE', #30516 ) ;
#7280=CARTESIAN_POINT ( 'NONE',  ( 0.02407890056655608360, 4.286445725888036407, 30.79383171238946204 ) ) ;
#7286=EDGE_LOOP ( 'NONE', ( #35031, #34623, #13433, #34456 ) ) ;
#7291=ORIENTED_EDGE ( 'NONE', *, *, #7902, .F. ) ;
#7299=DIRECTION ( 'NONE',  ( 0.000000000000000000, -1.000000000000000000, 0.000000000000000000 ) ) ;
#7308=ORIENTED_EDGE ( 'NONE', *, *, #25454, .T. ) ;
#7309=AXIS2_PLACEMENT_3D ( 'NONE', #18480, #34656, #113 ) ;
#7315=B_SPLINE_CURVE_WITH_KNOTS ( 'NONE', 3,
 ( #29229, #16385, #13870, #24710 ),
 .UNSPECIFIED., .F., .F.,
 ( 4, 4 ),
 ( 0.005298349227682424070, 0.005985217865144619280 ),
 .UNSPECIFIED. ) ;
#7319=CARTESIAN_POINT ( 'NONE',  ( 2.765921099433443331, 14.63235270440974922, -27.43224275967423509 ) ) ;
#7321=ORIENTED_EDGE ( 'NONE', *, *, #15287, .T. ) ;
#7324=DIRECTION ( 'NONE',  ( 0.000000000000000000, 0.000000000000000000, 1.000000000000000000 ) ) ;
#7334=DIRECTION ( 'NONE',  ( 0.000000000000000000, 0.000000000000000000, 1.000000000000000000 ) ) ;
#7339=DIRECTION ( 'NONE',  ( 0.000000000000000000, 0.000000000000000000, 1.000000000000000000 ) ) ;
#7347=AXIS2_PLACEMENT_3D ( 'NONE', #1659, #18062, #20532 ) ;
#7350=ORIENTED_EDGE ( 'NONE', *, *, #26356, .T. ) ;
#7360=ADVANCED_FACE ( 'NONE', ( #6989 ), #2028, .T. ) ;
#7361=CARTESIAN_POINT ( 'NONE',  ( 2.783107584500409626, 4.187058600949539411, 30.58452291340892160 ) ) ;
#7364=LINE ( 'NONE', #15067, #28731 ) ;
#7366=B_SPLINE_CURVE_WITH_KNOTS ( 'NONE', 3,
 ( #1785, #14985, #23499, #25821 ),
 .UNSPECIFIED., .F., .F.,
 ( 4, 4 ),
 ( 0.005298355823470651295, 0.005985224365431043858 ),
 .UNSPECIFIED. ) ;
#7374=CYLINDRICAL_SURFACE ( 'NONE', #20762, 2.524999999999999467 ) ;
#7390=CARTESIAN_POINT ( 'NONE',  ( -5.210000000000000853, 0.000000000000000000, 0.000000000000000000 ) ) ;
#7392=EDGE_LOOP ( 'NONE', ( #25845, #13798, #23914, #3380 ) ) ;
#7395=VERTEX_POINT ( 'NONE', #12525 ) ;
#7399=ORIENTED_EDGE ( 'NONE', *, *, #15315, .F. ) ;
#7405=CIRCLE ( 'NONE', #21064, 34.41491905851385269 ) ;
#7419=ORIENTED_EDGE ( 'NONE', *, *, #5701, .F. ) ;
#7423=CARTESIAN_POINT ( 'NONE',  ( 1.040000000000002034, 28.00026196654299326, -20.00929742917092824 ) ) ;
#7429=CARTESIAN_POINT ( 'NONE',  ( 0.000000000000000000, -17.83604598421681331, 24.70480026434162113 ) ) ;
#7432=CIRCLE ( 'NONE', #22299, 30.47050528711511674 ) ;
#7437=EDGE_LOOP ( 'NONE', ( #14980, #5588, #13560, #14411 ) ) ;
#7440=VECTOR ( 'NONE', #9138, 1000.000000000000000 ) ;
#7441=VERTEX_POINT ( 'NONE', #18754 ) ;
#7452=CARTESIAN_POINT ( 'NONE',  ( 2.033800774785157195, -2.658747979797710936, 33.81079988514328249 ) ) ;
#7453=CIRCLE ( 'NONE', #19405, 30.47050528711511674 ) ;
#7464=LINE ( 'NONE', #21009, #33348 ) ;
#7466=B_SPLINE_CURVE_WITH_KNOTS ( 'NONE', 3,
 ( #1159, #33725, #20214, #35092 ),
 .UNSPECIFIED., .F., .F.,
 ( 4, 4 ),
 ( 2.128468106753875164E-07, 0.0006879486673519094857 ),
 .UNSPECIFIED. ) ;
#7471=CARTESIAN_POINT ( 'NONE',  ( 0.07094833857658310039, -31.66307346108432341, -1.400387680934324308 ) ) ;
#7473=CARTESIAN_POINT ( 'NONE',  ( 0.000000000000000000, 0.000000000000000000, 10.00000000000000000 ) ) ;
#7475=CARTESIAN_POINT ( 'NONE',  ( 0.07098929236673945375, -8.452877438714468283, 30.54658108095609848 ) ) ;
#7480=AXIS2_PLACEMENT_3D ( 'NONE', #28760, #26258, #2058 ) ;
#7488=DIRECTION ( 'NONE',  ( 0.000000000000000000, 0.000000000000000000, -1.000000000000000000 ) ) ;
#7498=CARTESIAN_POINT ( 'NONE',  ( 0.1859802865221972246, 25.38927130757771877, 19.93727243998150556 ) ) ;
#7499=EDGE_LOOP ( 'NONE', ( #6308, #14214, #1903, #2232, #22505, #28404 ) ) ;
#7501=CARTESIAN_POINT ( 'NONE',  ( 0.000000000000000000, 3.909681563761695067, 30.21863799912385673 ) ) ;
#7505=CARTESIAN_POINT ( 'NONE',  ( 2.765921099433443331, 26.03801215795517621, 16.98986790278620873 ) ) ;
#7506=ORIENTED_EDGE ( 'NONE', *, *, #10904, .F. ) ;
#7510=AXIS2_PLACEMENT_3D ( 'NONE', #2397, #18449, #34807 ) ;
#7530=CARTESIAN_POINT ( 'NONE',  ( 2.789999999999999147, -29.00730259674844902, 9.328884633908842261 ) ) ;
#7531=ORIENTED_EDGE ( 'NONE', *, *, #32979, .T. ) ;
#7552=CARTESIAN_POINT ( 'NONE',  ( 2.789999999999999147, -5.984944020945660803, -31.37417528048448645 ) ) ;
#7554=LINE ( 'NONE', #15596, #11189 ) ;
#7559=CARTESIAN_POINT ( 'NONE',  ( 2.765921099433443775, -11.07880054387241664, 29.04985141099759360 ) ) ;
#7563=LINE ( 'NONE', #32129, #9304 ) ;
#7564=ORIENTED_EDGE ( 'NONE', *, *, #10405, .T. ) ;
#7570=VERTEX_POINT ( 'NONE', #7690 ) ;
#7585=EDGE_LOOP ( 'NONE', ( #15443, #6228, #14053, #20033, #23160, #2804, #35019, #7419 ) ) ;
#7596=B_SPLINE_CURVE_WITH_KNOTS ( 'NONE', 3,
 ( #4821, #26548, #18567, #23873 ),
 .UNSPECIFIED., .F., .F.,
 ( 4, 4 ),
 ( 0.005298360586756152568, 0.005985229062776067227 ),
 .UNSPECIFIED. ) ;
#7597=DIRECTION ( 'NONE',  ( 0.000000000000000000, 0.000000000000000000, 1.000000000000000000 ) ) ;
#7598=CARTESIAN_POINT ( 'NONE',  ( 0.1859802613287491191, 26.80718912072172344, -17.98567582844204438 ) ) ;
#7611=CIRCLE ( 'NONE', #33205, 34.41491905851385269 ) ;
#7614=CARTESIAN_POINT ( 'NONE',  ( 0.000000000000000000, 7.489092610871091793, 29.53582882395389930 ) ) ;
#7615=DIRECTION ( 'NONE',  ( -1.000000000000000000, -0.000000000000000000, -0.000000000000000000 ) ) ;
#7617=VECTOR ( 'NONE', #29535, 1000.000000000000000 ) ;
#7623=ORIENTED_EDGE ( 'NONE', *, *, #30632, .F. ) ;
#7627=B_SPLINE_CURVE_WITH_KNOTS ( 'NONE', 3,
 ( #8479, #301, #14369, #8828, #25193, #30553 ),
 .UNSPECIFIED., .F., .F.,
 ( 4, 2, 4 ),
 ( 4.404817168095868535E-07, 0.001874269729529001467, 0.003748098977341193273 ),
 .UNSPECIFIED. ) ;
#7630=EDGE_CURVE ( 'NONE', #916, #27137, #16276, .T. ) ;
#7632=DIRECTION ( 'NONE',  ( 0.000000000000000000, 0.000000000000000000, 1.000000000000000000 ) ) ;
#7637=VECTOR ( 'NONE', #29427, 1000.000000000000000 ) ;
#7639=ORIENTED_EDGE ( 'NONE', *, *, #12710, .F. ) ;
#7641=DIRECTION ( 'NONE',  ( 0.000000000000000000, 0.000000000000000000, 1.000000000000000000 ) ) ;
#7642=ORIENTED_EDGE ( 'NONE', *, *, #28523, .T. ) ;
#7650=CYLINDRICAL_SURFACE ( 'NONE', #2680, 10.00000000000000000 ) ;
#7651=CARTESIAN_POINT ( 'NONE',  ( 0.02407890056655564992, -0.3931553186911057041, -31.08824725498900676 ) ) ;
#7654=CARTESIAN_POINT ( 'NONE',  ( 1.749999999999999778, 6.714005886385429278, -33.75364837705166110 ) ) ;
#7658=CARTESIAN_POINT ( 'NONE',  ( 0.000000000000000000, -0.09145294252700143789, 30.47036804522410236 ) ) ;
#7659=CARTESIAN_POINT ( 'NONE',  ( -5.210000000000000853, 0.000000000000000000, 0.000000000000000000 ) ) ;
#7667=DIRECTION ( 'NONE',  ( -1.000000000000000000, -0.000000000000000000, -0.000000000000000000 ) ) ;
#7669=ORIENTED_EDGE ( 'NONE', *, *, #12702, .T. ) ;
#7671=DIRECTION ( 'NONE',  ( -1.000000000000000000, 0.000000000000000000, 0.000000000000000000 ) ) ;
#7680=AXIS2_PLACEMENT_3D ( 'NONE', #12713, #15378, #13057 ) ;
#7681=B_SPLINE_CURVE_WITH_KNOTS ( 'NONE', 3,
 ( #23052, #9520, #31230, #15046, #11673, #19681 ),
 .UNSPECIFIED., .F., .F.,
 ( 4, 2, 4 ),
 ( 4.404817011923048155E-07, 0.001874269613276477800, 0.003748098744851763222 ),
 .UNSPECIFIED. ) ;
#7686=CARTESIAN_POINT ( 'NONE',  ( 0.07098932668446723826, 14.74869129583196958, 28.05389252521654342 ) ) ;
#7687=FACE_OUTER_BOUND ( 'NONE', #20874, .T. ) ;
#7688=ORIENTED_EDGE ( 'NONE', *, *, #23863, .T. ) ;
#7690=CARTESIAN_POINT ( 'NONE',  ( 0.02407890056655738464, 28.29688452313417812, -12.88099432405573630 ) ) ;
#7697=EDGE_CURVE ( 'NONE', #8132, #23220, #1522, .T. ) ;
#7698=CARTESIAN_POINT ( 'NONE',  ( 2.265105863614538695, 20.67343389904883111, 26.20724806577312904 ) ) ;
#7712=ORIENTED_EDGE ( 'NONE', *, *, #2390, .T. ) ;
#7721=VERTEX_POINT ( 'NONE', #11082 ) ;
#7730=DIRECTION ( 'NONE',  ( 0.000000000000000000, 0.000000000000000000, 1.000000000000000000 ) ) ;
#7733=EDGE_CURVE ( 'NONE', #13445, #21650, #25110, .T. ) ;
#7734=VECTOR ( 'NONE', #21322, 1000.000000000000000 ) ;
#7737=EDGE_CURVE ( 'NONE', #14830, #1305, #840, .T. ) ;
#7749=ADVANCED_FACE ( 'NONE', ( #4567 ), #1744, .T. ) ;
#7761=CARTESIAN_POINT ( 'NONE',  ( 2.765921099433442443, 31.00221527374952046, -2.344426712874310148 ) ) ;
#7769=B_SPLINE_CURVE_WITH_KNOTS ( 'NONE', 3,
 ( #21611, #8430, #13604, #21964 ),
 .UNSPECIFIED., .F., .F.,
 ( 4, 4 ),
 ( 2.876507994500877895E-07, 0.0006880240977454964548 ),
 .UNSPECIFIED. ) ;
#7778=LINE ( 'NONE', #29677, #7734 ) ;
#7784=ORIENTED_EDGE ( 'NONE', *, *, #26682, .T. ) ;
#7786=EDGE_CURVE ( 'NONE', #17311, #24353, #5919, .T. ) ;
#7791=DIRECTION ( 'NONE',  ( 1.000000000000000000, -0.000000000000000000, -0.000000000000000000 ) ) ;
#7793=FACE_OUTER_BOUND ( 'NONE', #11460, .T. ) ;
#7804=CIRCLE ( 'NONE', #30538, 30.47050528711512030 ) ;
#7807=CARTESIAN_POINT ( 'NONE',  ( 0.000000000000000000, -27.53147453683416757, -13.05640081644872197 ) ) ;
#7812=EDGE_CURVE ( 'NONE', #6257, #33253, #6593, .T. ) ;
#7822=B_SPLINE_CURVE_WITH_KNOTS ( 'NONE', 3,
 ( #8271, #448, #13448, #11132, #32820, #22157 ),
 .UNSPECIFIED., .F., .F.,
 ( 4, 2, 4 ),
 ( 1.974571759321287545E-07, 0.001873395748763630230, 0.003746594040351328408 ),
 .UNSPECIFIED. ) ;
#7823=CARTESIAN_POINT ( 'NONE',  ( 2.789999999999999147, -3.728217946242703196, -30.24156218513559935 ) ) ;
#7827=TOROIDAL_SURFACE ( 'NONE', #14698, 30.47050528711511674, 8.000000000000000000 ) ;
#7836=CIRCLE ( 'NONE', #14105, 30.47050528711511674 ) ;
#7841=CARTESIAN_POINT ( 'NONE',  ( 2.789999999999999147, 31.00221527374952046, 2.344426712874309260 ) ) ;
#7842=ADVANCED_FACE ( 'NONE', ( #18666 ), #29511, .F. ) ;
#7847=PRODUCT_DEFINITION_CONTEXT ( 'detailed design', #12152, 'design' ) ;
#7848=ORIENTED_EDGE ( 'NONE', *, *, #14205, .T. ) ;
#7849=ORIENTED_EDGE ( 'NONE', *, *, #30287, .T. ) ;
#7850=DIRECTION ( 'NONE',  ( -1.000000000000000000, -0.000000000000000000, -0.000000000000000000 ) ) ;
#7858=CARTESIAN_POINT ( 'NONE',  ( 1.749999999999999778, -18.66807150955392913, -28.91175816027522671 ) ) ;
#7860=ORIENTED_EDGE ( 'NONE', *, *, #29038, .F. ) ;
#7862=CIRCLE ( 'NONE', #23152, 2.525000000000001243 ) ;
#7864=CARTESIAN_POINT ( 'NONE',  ( 0.000000000000000000, 25.67797970382157402, -16.40405592474731833 ) ) ;
#7869=B_SPLINE_CURVE_WITH_KNOTS ( 'NONE', 3,
 ( #5481, #513, #27376, #19217, #22048, #13682 ),
 .UNSPECIFIED., .F., .F.,
 ( 4, 2, 4 ),
 ( 2.008842330397746412E-07, 0.001873399179558948857, 0.003746597474884857948 ),
 .UNSPECIFIED. ) ;
#7874=PLANE ( 'NONE',  #23193 ) ;
#7876=CARTESIAN_POINT ( 'NONE',  ( 0.7561992144253976145, -25.08322906883816117, -22.82697412903104350 ) ) ;
#7879=DIRECTION ( 'NONE',  ( -1.000000000000000000, -0.000000000000000000, -0.000000000000000000 ) ) ;
#7880=CARTESIAN_POINT ( 'NONE',  ( 2.765921099433441999, -17.95514392185434360, 25.38201125280350468 ) ) ;
#7887=CARTESIAN_POINT ( 'NONE',  ( 2.265105745614923727, -33.37077467988373058, -0.7759739055977695754 ) ) ;
#7893=ORIENTED_EDGE ( 'NONE', *, *, #1833, .F. ) ;
#7895=EDGE_LOOP ( 'NONE', ( #18240, #17119, #7639, #33474 ) ) ;
#7898=ORIENTED_EDGE ( 'NONE', *, *, #10412, .F. ) ;
#7899=DIRECTION ( 'NONE',  ( -1.000000000000000000, -0.000000000000000000, -0.000000000000000000 ) ) ;
#7901=EDGE_CURVE ( 'NONE', #11290, #15534, #32338, .T. ) ;
#7902=EDGE_CURVE ( 'NONE', #25989, #11449, #12326, .T. ) ;
#7918=CARTESIAN_POINT ( 'NONE',  ( 2.789999999999999147, -29.91351748324107263, 5.799410679710522487 ) ) ;
#7927=CARTESIAN_POINT ( 'NONE',  ( 2.033800775632456759, -29.46088656861438793, -16.80164552011282808 ) ) ;
#7937=CARTESIAN_POINT ( 'NONE',  ( 1.395000000000002238, -34.41385771548413430, -0.2702793785573798790 ) ) ;
#7941=EDGE_CURVE ( 'NONE', #28175, #30030, #7778, .T. ) ;
#7944=ORIENTED_EDGE ( 'NONE', *, *, #762, .F. ) ;
#7945=ORIENTED_EDGE ( 'NONE', *, *, #5916, .T. ) ;
#7946=VERTEX_POINT ( 'NONE', #5278 ) ;
#7952=FACE_OUTER_BOUND ( 'NONE', #26976, .T. ) ;
#7956=DIRECTION ( 'NONE',  ( -1.000000000000000000, 0.000000000000000000, -0.000000000000000000 ) ) ;
#7958=DIRECTION ( 'NONE',  ( 0.000000000000000000, 0.000000000000000000, 1.000000000000000000 ) ) ;
#7971=ORIENTED_EDGE ( 'NONE', *, *, #17089, .F. ) ;
#7974=ORIENTED_EDGE ( 'NONE', *, *, #14348, .T. ) ;
#8018=VERTEX_POINT ( 'NONE', #22733 ) ;
#8030=CARTESIAN_POINT ( 'NONE',  ( 2.789999999999999147, -17.95514392185398833, -25.38201125280375692 ) ) ;
#8033=ADVANCED_FACE ( 'NONE', ( #27877 ), #11348, .T. ) ;
#8036=DIRECTION ( 'NONE',  ( 0.000000000000000000, 0.000000000000000000, -1.000000000000000000 ) ) ;
#8037=DIRECTION ( 'NONE',  ( -1.000000000000000000, -0.000000000000000000, -0.000000000000000000 ) ) ;
#8039=DIRECTION ( 'NONE',  ( -1.000000000000000000, -0.000000000000000000, -0.000000000000000000 ) ) ;
#8044=DIRECTION ( 'NONE',  ( 0.000000000000000000, -1.000000000000000000, -0.000000000000000000 ) ) ;
#8048=AXIS2_PLACEMENT_3D ( 'NONE', #26532, #18892, #23859 ) ;
#8055=ORIENTED_EDGE ( 'NONE', *, *, #15598, .F. ) ;
#8057=DIRECTION ( 'NONE',  ( 0.000000000000000000, 0.000000000000000000, 1.000000000000000000 ) ) ;
#8061=ADVANCED_FACE ( 'NONE', ( #5980 ), #27346, .T. ) ;
#8064=EDGE_CURVE ( 'NONE', #2517, #2454, #3491, .T. ) ;
#8078=ORIENTED_EDGE ( 'NONE', *, *, #5715, .T. ) ;
#8079=ORIENTED_EDGE ( 'NONE', *, *, #4051, .T. ) ;
#8084=DIRECTION ( 'NONE',  ( 0.000000000000000000, -0.5877852522924686962, -0.8090169943749506709 ) ) ;
#8088=ORIENTED_EDGE ( 'NONE', *, *, #17426, .T. ) ;
#8090=CARTESIAN_POINT ( 'NONE',  ( -8.427639665100776541E-14, -7.838364976555423524, -29.64395146466218733 ) ) ;
#8092=CARTESIAN_POINT ( 'NONE',  ( 2.265105727189284046, 7.015288891537251992, -32.63428354963176048 ) ) ;
#8096=CARTESIAN_POINT ( 'NONE',  ( 0.02407890056655825201, -3.506335382740311868, -30.89238256715869468 ) ) ;
#8106=CARTESIAN_POINT ( 'NONE',  ( 1.749999999999999778, 0.000000000000000000, 0.000000000000000000 ) ) ;
#8107=CARTESIAN_POINT ( 'NONE',  ( 2.719051668539516076, -31.01658195443389943, -6.517894193013122006 ) ) ;
#8126=DIRECTION ( 'NONE',  ( 1.000000000000000000, -0.000000000000000000, -0.000000000000000000 ) ) ;
#8132=VERTEX_POINT ( 'NONE', #3321 ) ;
#8135=CARTESIAN_POINT ( 'NONE',  ( 2.790000000000082192, -0.2199561701061230334, 30.66195251245370201 ) ) ;
#8136=ORIENTED_EDGE ( 'NONE', *, *, #13110, .T. ) ;
#8138=ORIENTED_EDGE ( 'NONE', *, *, #33019, .F. ) ;
#8144=B_SPLINE_CURVE_WITH_KNOTS ( 'NONE', 3,
 ( #5833, #27736, #16728, #27910 ),
 .UNSPECIFIED., .F., .F.,
 ( 4, 4 ),
 ( 0.005298437004852360292, 0.005985304466813747698 ),
 .UNSPECIFIED. ) ;
#8146=DIRECTION ( 'NONE',  ( 0.000000000000000000, 0.000000000000000000, 1.000000000000000000 ) ) ;
#8150=ORIENTED_EDGE ( 'NONE', *, *, #26237, .T. ) ;
#8167=CARTESIAN_POINT ( 'NONE',  ( 2.033800798445904334, -29.97203090897430755, 15.87187733270971357 ) ) ;
#8169=DIRECTION ( 'NONE',  ( -1.000000000000000000, 0.000000000000000000, -0.000000000000000000 ) ) ;
#8171=EDGE_LOOP ( 'NONE', ( #15773, #784, #20770, #5640, #6688, #856, #27053, #21822 ) ) ;
#8173=ORIENTED_EDGE ( 'NONE', *, *, #11271, .T. ) ;
#8176=CIRCLE ( 'NONE', #795, 2.525000000000000355 ) ;
#8185=CYLINDRICAL_SURFACE ( 'NONE', #34174, 34.41491905851385269 ) ;
#8189=VECTOR ( 'NONE', #2421, 1000.000000000000000 ) ;
#8191=EDGE_CURVE ( 'NONE', #23670, #26414, #11050, .T. ) ;
#8194=VERTEX_POINT ( 'NONE', #31092 ) ;
#8197=EDGE_CURVE ( 'NONE', #2635, #1617, #34821, .T. ) ;
#8198=LINE ( 'NONE', #13669, #15439 ) ;
#8213=CARTESIAN_POINT ( 'NONE',  ( 2.789999999999998703, -27.64940622781567470, 13.25307083675137321 ) ) ;
#8214=CARTESIAN_POINT ( 'NONE',  ( 2.789999999999999147, -25.83993731729781729, -18.77381338200996552 ) ) ;
#8225=LINE ( 'NONE', #26744, #7637 ) ;
#8226=CARTESIAN_POINT ( 'NONE',  ( -5.210000000000000853, 0.000000000000000000, 0.000000000000000000 ) ) ;
#8229=CARTESIAN_POINT ( 'NONE',  ( 0.000000000000000000, 27.60935207499554522, 12.89090262359660422 ) ) ;
#8239=CARTESIAN_POINT ( 'NONE',  ( 0.000000000000000000, -11.13185981125894486, 28.36429779836949194 ) ) ;
#8248=EDGE_CURVE ( 'NONE', #21282, #292, #30137, .T. ) ;
#8251=CARTESIAN_POINT ( 'NONE',  ( 1.039999999999999591, -30.28730148581173864, 16.34215476954022606 ) ) ;
#8256=CIRCLE ( 'NONE', #21907, 30.47050528711512030 ) ;
#8257=CARTESIAN_POINT ( 'NONE',  ( 2.789999999999999147, 9.869977788040968036, 30.37666815053940539 ) ) ;
#8258=CIRCLE ( 'NONE', #28165, 30.47050528711511674 ) ;
#8261=CARTESIAN_POINT ( 'NONE',  ( 2.789999999999999147, -30.46391896562411716, 6.211548095912460710 ) ) ;
#8270=CARTESIAN_POINT ( 'NONE',  ( 2.765921099433442887, -30.46391896562411716, 6.211548095912460710 ) ) ;
#8271=CARTESIAN_POINT ( 'NONE',  ( 2.765921099433441999, -29.68817180695669578, -9.232883799364548949 ) ) ;
#8299=ORIENTED_EDGE ( 'NONE', *, *, #1011, .F. ) ;
#8303=B_SPLINE_CURVE_WITH_KNOTS ( 'NONE', 3,
 ( #33944, #26273, #17764, #31106 ),
 .UNSPECIFIED., .F., .F.,
 ( 4, 4 ),
 ( 0.005298558704933904739, 0.005985424570307885592 ),
 .UNSPECIFIED. ) ;
#8315=FACE_OUTER_BOUND ( 'NONE', #29881, .T. ) ;
#8323=AXIS2_PLACEMENT_3D ( 'NONE', #25636, #12136, #25816 ) ;
#8324=ORIENTED_EDGE ( 'NONE', *, *, #12466, .T. ) ;
#8330=EDGE_LOOP ( 'NONE', ( #23074, #30747, #21901, #23065, #10414, #10256 ) ) ;
#8332=B_SPLINE_CURVE_WITH_KNOTS ( 'NONE', 3,
 ( #24889, #24362, #1404, #17452, #14941, #3710 ),
 .UNSPECIFIED., .F., .F.,
 ( 4, 2, 4 ),
 ( 4.404817130298605098E-07, 0.001874269701320913691, 0.003748098920928797251 ),
 .UNSPECIFIED. ) ;
#8335=VERTEX_POINT ( 'NONE', #21270 ) ;
#8338=DIRECTION ( 'NONE',  ( 0.000000000000000000, 0.000000000000000000, 1.000000000000000000 ) ) ;
#8339=B_SPLINE_CURVE_WITH_KNOTS ( 'NONE', 3,
 ( #1093, #11964, #22808, #20147, #26517, #26695 ),
 .UNSPECIFIED., .F., .F.,
 ( 4, 2, 4 ),
 ( 4.404817006251796231E-07, 0.001874269609036412904, 0.003748098736372200684 ),
 .UNSPECIFIED. ) ;
#8343=EDGE_LOOP ( 'NONE', ( #19380, #18008, #8136, #20464 ) ) ;
#8349=CARTESIAN_POINT ( 'NONE',  ( 2.033589665476111197, -29.97226545381508345, -15.87222719455825093 ) ) ;
#8356=CARTESIAN_POINT ( 'NONE',  ( 0.02407890056655608360, 4.286445725888036407, 30.79383171238946204 ) ) ;
#8357=EDGE_LOOP ( 'NONE', ( #886, #19574, #21910, #11985 ) ) ;
#8367=DIRECTION ( 'NONE',  ( 0.000000000000000000, 0.000000000000000000, 1.000000000000000000 ) ) ;
#8369=CARTESIAN_POINT ( 'NONE',  ( 2.033589655956525188, -2.658578268446866399, -33.81118535743541287 ) ) ;
#8378=ORIENTED_EDGE ( 'NONE', *, *, #24585, .T. ) ;
#8391=EDGE_LOOP ( 'NONE', ( #18046, #29754, #34842, #24361, #11316, #11586 ) ) ;
#8396=DIRECTION ( 'NONE',  ( -1.000000000000000000, -0.000000000000000000, -0.000000000000000000 ) ) ;
#8397=CARTESIAN_POINT ( 'NONE',  ( -10.00000000000000000, 0.000000000000000000, 0.000000000000000000 ) ) ;
#8405=DIRECTION ( 'NONE',  ( 0.000000000000000000, 0.000000000000000000, 1.000000000000000000 ) ) ;
#8407=EDGE_CURVE ( 'NONE', #245, #6008, #7554, .T. ) ;
#8410=CARTESIAN_POINT ( 'NONE',  ( 1.039999999999999147, -24.90160365674884346, 23.75493189058332177 ) ) ;
#8412=DIRECTION ( 'NONE',  ( 0.000000000000000000, 0.000000000000000000, 1.000000000000000000 ) ) ;
#8414=DIRECTION ( 'NONE',  ( 0.000000000000000000, 0.000000000000000000, 1.000000000000000000 ) ) ;
#8418=ORIENTED_EDGE ( 'NONE', *, *, #29791, .T. ) ;
#8420=CIRCLE ( 'NONE', #26059, 34.41491905851385269 ) ;
#8421=AXIS2_PLACEMENT_3D ( 'NONE', #32368, #164, #2652 ) ;
#8430=CARTESIAN_POINT ( 'NONE',  ( 2.783128855593303808, -27.79352918700739394, -13.43306967213438696 ) ) ;
#8434=CARTESIAN_POINT ( 'NONE',  ( 2.606461835800627291, -0.8174345826529154646, -32.26081300283389197 ) ) ;
#8438=AXIS2_PLACEMENT_3D ( 'NONE', #34355, #17831, #21005 ) ;
#8440=VERTEX_POINT ( 'NONE', #23930 ) ;
#8442=CIRCLE ( 'NONE', #31732, 30.47050528711512030 ) ;
#8446=ORIENTED_EDGE ( 'NONE', *, *, #28258, .F. ) ;
#8450=CARTESIAN_POINT ( 'NONE',  ( 0.1859802949991362364, -30.94574698966622250, -9.190792961030568975 ) ) ;
#8452=B_SPLINE_CURVE_WITH_KNOTS ( 'NONE', 3,
 ( #56, #2369, #13593, #29436 ),
 .UNSPECIFIED., .F., .F.,
 ( 4, 4 ),
 ( 0.005298352064454681272, 0.005985220659832064284 ),
 .UNSPECIFIED. ) ;
#8455=CARTESIAN_POINT ( 'NONE',  ( 4.170026905643898252E-16, 25.77033216996917631, 16.61395588374081456 ) ) ;
#8457=CARTESIAN_POINT ( 'NONE',  ( 0.1835380964117766245, -22.67993007562076357, 22.95754798008695019 ) ) ;
#8465=VECTOR ( 'NONE', #2047, 1000.000000000000000 ) ;
#8467=ORIENTED_EDGE ( 'NONE', *, *, #25454, .F. ) ;
#8473=CIRCLE ( 'NONE', #7309, 2.524999999999999467 ) ;
#8475=CARTESIAN_POINT ( 'NONE',  ( 1.749999999999999778, 6.714005886384948774, 33.75364837705175347 ) ) ;
#8479=CARTESIAN_POINT ( 'NONE',  ( 1.749999999999999778, 14.40815186467820475, -31.25366880301303496 ) ) ;
#8490=CARTESIAN_POINT ( 'NONE',  ( 0.5248940569443696358, -17.22577838686597218, 28.59166429730529657 ) ) ;
#8493=VECTOR ( 'NONE', #24052, 1000.000000000000000 ) ;
#8501=CARTESIAN_POINT ( 'NONE',  ( 0.000000000000000000, 17.11426446101236820, -26.96776559937708129 ) ) ;
#8502=CYLINDRICAL_SURFACE ( 'NONE', #32698, 16.19999999999999929 ) ;
#8510=CARTESIAN_POINT ( 'NONE',  ( 1.749999999999999778, 0.000000000000000000, 0.000000000000000000 ) ) ;
#8512=CARTESIAN_POINT ( 'NONE',  ( 0.5288002472147362854, -24.86182815675670810, 22.28830832814871599 ) ) ;
#8522=CARTESIAN_POINT ( 'NONE',  ( 2.719051668256705856, -22.12275578582363877, 22.69570394412120251 ) ) ;
#8523=ORIENTED_EDGE ( 'NONE', *, *, #19695, .T. ) ;
#8524=ORIENTED_EDGE ( 'NONE', *, *, #15558, .F. ) ;
#8526=VERTEX_POINT ( 'NONE', #16476 ) ;
#8527=DIRECTION ( 'NONE',  ( 0.000000000000000000, 0.000000000000000000, 1.000000000000000000 ) ) ;
#8528=DIRECTION ( 'NONE',  ( -1.000000000000000000, -0.000000000000000000, -0.000000000000000000 ) ) ;
#8540=CARTESIAN_POINT ( 'NONE',  ( 2.765921099433443331, -3.506335382740311868, -30.89238256715869468 ) ) ;
#8545=ORIENTED_EDGE ( 'NONE', *, *, #20382, .T. ) ;
#8546=CARTESIAN_POINT ( 'NONE',  ( 0.02407890056655608360, 14.63235270440974922, -27.43224275967423509 ) ) ;
#8553=DIRECTION ( 'NONE',  ( 0.000000000000000000, 0.000000000000000000, 1.000000000000000000 ) ) ;
#8556=CARTESIAN_POINT ( 'NONE',  ( 2.606461833931011274, -18.30111164264898704, 26.58002197185221149 ) ) ;
#8559=VERTEX_POINT ( 'NONE', #21792 ) ;
#8560=EDGE_LOOP ( 'NONE', ( #23090, #25447, #23085, #3124, #10169, #31747 ) ) ;
#8569=CARTESIAN_POINT ( 'NONE',  ( 2.789999999999999147, -17.83604598421647935, -24.70480026434183429 ) ) ;
#8572=CARTESIAN_POINT ( 'NONE',  ( 0.1835382041699210043, -11.11596589742306129, -30.29626325691716815 ) ) ;
#8573=CARTESIAN_POINT ( 'NONE',  ( 0.7561992263075686393, 6.875399836226445238, 33.21096214980147465 ) ) ;
#8574=CIRCLE ( 'NONE', #19975, 30.47050528711512030 ) ;
#8587=B_SPLINE_CURVE_WITH_KNOTS ( 'NONE', 3,
 ( #4830, #15725, #12878, #7864 ),
 .UNSPECIFIED., .F., .F.,
 ( 4, 4 ),
 ( 2.557638148655773837E-07, 0.0006879919438241504466 ),
 .UNSPECIFIED. ) ;
#8595=DIRECTION ( 'NONE',  ( -1.000000000000000000, 0.000000000000000000, -0.000000000000000000 ) ) ;
#8610=ORIENTED_EDGE ( 'NONE', *, *, #13820, .T. ) ;
#8611=AXIS2_PLACEMENT_3D ( 'NONE', #30397, #33768, #27542 ) ;
#8617=CARTESIAN_POINT ( 'NONE',  ( 2.606461796175087997, 7.231184547465761447, -31.45056812073505270 ) ) ;
#8621=CARTESIAN_POINT ( 'NONE',  ( 2.265105899770494702, 27.45362965837546909, -18.98707279867223008 ) ) ;
#8623=EDGE_CURVE ( 'NONE', #32949, #11691, #17883, .T. ) ;
#8639=ORIENTED_EDGE ( 'NONE', *, *, #12857, .T. ) ;
#8645=CARTESIAN_POINT ( 'NONE',  ( 1.040000000000002034, 32.09669216789253454, -12.41728656686340315 ) ) ;
#8653=CARTESIAN_POINT ( 'NONE',  ( 0.02407890056655608360, 14.63235270440974922, -27.43224275967423509 ) ) ;
#8655=CARTESIAN_POINT ( 'NONE',  ( 0.02407890056655695096, -21.56796757982826307, 22.39322359481599278 ) ) ;
#8661=B_SPLINE_CURVE_WITH_KNOTS ( 'NONE', 3,
 ( #2522, #7686, #29050, #13401, #16255, #2003 ),
 .UNSPECIFIED., .F., .F.,
 ( 4, 2, 4 ),
 ( 2.008842330431681463E-07, 0.001873399179558949725, 0.003746597474884856213 ),
 .UNSPECIFIED. ) ;
#8670=CARTESIAN_POINT ( 'NONE',  ( 2.765921099433443331, -29.68817180695682723, 9.232883799364120847 ) ) ;
#8690=CIRCLE ( 'NONE', #22341, 34.41491905851385269 ) ;
#8698=CARTESIAN_POINT ( 'NONE',  ( 2.265105948359096288, -29.61686074518757295, 15.39650178189414476 ) ) ;
#8699=VERTEX_POINT ( 'NONE', #31047 ) ;
#8703=VERTEX_POINT ( 'NONE', #22693 ) ;
#8710=VERTEX_POINT ( 'NONE', #33890 ) ;
#8712=DIRECTION ( 'NONE',  ( 0.000000000000000000, 0.000000000000000000, 1.000000000000000000 ) ) ;
#8713=EDGE_CURVE ( 'NONE', #22746, #3220, #21230, .T. ) ;
#8725=ORIENTED_EDGE ( 'NONE', *, *, #30283, .T. ) ;
#8729=ORIENTED_EDGE ( 'NONE', *, *, #24585, .F. ) ;
#8743=ORIENTED_EDGE ( 'NONE', *, *, #23664, .F. ) ;
#8744=ADVANCED_FACE ( 'NONE', ( #18925 ), #3142, .T. ) ;
#8751=CARTESIAN_POINT ( 'NONE',  ( 2.033800778643362506, 33.71011734938328885, -3.723857881850640261 ) ) ;
#8757=CARTESIAN_POINT ( 'NONE',  ( 0.000000000000000000, 12.80000000000000071, 3.000000000000000000 ) ) ;
#8770=ORIENTED_EDGE ( 'NONE', *, *, #13867, .F. ) ;
#8789=ADVANCED_FACE ( 'NONE', ( #15736 ), #1573, .T. ) ;
#8793=AXIS2_PLACEMENT_3D ( 'NONE', #9114, #25656, #6432 ) ;
#8801=DIRECTION ( 'NONE',  ( -1.000000000000000000, -0.000000000000000000, -0.000000000000000000 ) ) ;
#8802=DIRECTION ( 'NONE',  ( 0.000000000000000000, -0.9048270524660176894, -0.4257792915650768228 ) ) ;
#8816=DIRECTION ( 'NONE',  ( -1.000000000000000000, 0.000000000000000000, 0.000000000000000000 ) ) ;
#8828=CARTESIAN_POINT ( 'NONE',  ( 2.604019739527419830, 12.64393372169708130, -29.70253967906851500 ) ) ;
#8829=DIRECTION ( 'NONE',  ( 0.000000000000000000, 0.000000000000000000, 1.000000000000000000 ) ) ;
#8835=EDGE_CURVE ( 'NONE', #14930, #21561, #23402, .T. ) ;
#8836=B_SPLINE_CURVE_WITH_KNOTS ( 'NONE', 3,
 ( #14541, #19696, #471, #24838 ),
 .UNSPECIFIED., .F., .F.,
 ( 4, 4 ),
 ( 0.005298373595863127387, 0.005985241895929838650 ),
 .UNSPECIFIED. ) ;
#8838=VERTEX_POINT ( 'NONE', #1832 ) ;
#8845=ORIENTED_EDGE ( 'NONE', *, *, #4752, .F. ) ;
#8846=DIRECTION ( 'NONE',  ( -1.000000000000000000, -0.000000000000000000, -0.000000000000000000 ) ) ;
#8850=AXIS2_PLACEMENT_3D ( 'NONE', #9639, #29019, #4615 ) ;
#8852=EDGE_CURVE ( 'NONE', #6869, #6749, #27093, .T. ) ;
#8864=CARTESIAN_POINT ( 'NONE',  ( 0.000000000000000000, 30.93646776788796160, 7.943134866716423659 ) ) ;
#8866=DIRECTION ( 'NONE',  ( 0.000000000000000000, 0.000000000000000000, 1.000000000000000000 ) ) ;
#8874=DIRECTION ( 'NONE',  ( 0.000000000000000000, 0.000000000000000000, 1.000000000000000000 ) ) ;
#8891=AXIS2_PLACEMENT_3D ( 'NONE', #22112, #5889, #24580 ) ;
#8892=CARTESIAN_POINT ( 'NONE',  ( 2.765921099433440666, -11.07880054387200985, -29.04985141099774637 ) ) ;
#8896=CARTESIAN_POINT ( 'NONE',  ( 2.719010718194136533, 29.95554370010558287, -10.35423322779145217 ) ) ;
#8900=ORIENTED_EDGE ( 'NONE', *, *, #32290, .T. ) ;
#8905=CYLINDRICAL_SURFACE ( 'NONE', #30614, 34.41491905851385269 ) ;
#8907=CIRCLE ( 'NONE', #22568, 34.41491905851385269 ) ;
#8910=PRODUCT_CONTEXT ( 'NONE', #2351, 'mechanical' ) ;
#8917=ORIENTED_EDGE ( 'NONE', *, *, #8999, .T. ) ;
#8926=CARTESIAN_POINT ( 'NONE',  ( 2.261199756575918762, 31.32081674369869972, 11.57089561809684497 ) ) ;
#8929=EDGE_CURVE ( 'NONE', #5130, #20230, #15347, .T. ) ;
#8946=ORIENTED_EDGE ( 'NONE', *, *, #13711, .T. ) ;
#8947=EDGE_LOOP ( 'NONE', ( #33352, #10310, #5219, #18601, #4901, #33551, #8078, #14686 ) ) ;
#8949=EDGE_CURVE ( 'NONE', #23519, #4330, #6816, .T. ) ;
#8952=TOROIDAL_SURFACE ( 'NONE', #27064, 30.47050528711511674, 8.000000000000000000 ) ;
#8954=ORIENTED_EDGE ( 'NONE', *, *, #25706, .T. ) ;
#8957=EDGE_CURVE ( 'NONE', #23973, #7721, #4373, .T. ) ;
#8970=CARTESIAN_POINT ( 'NONE',  ( 0.02407890056655651728, 18.59128259035506758, -24.91982945642901726 ) ) ;
#8976=CARTESIAN_POINT ( 'NONE',  ( 0.1835381908571713794, -3.232363112765380464, -32.10887868571001746 ) ) ;
#8979=CARTESIAN_POINT ( 'NONE',  ( 0.001366356357610495681, -26.04873650956165676, -16.24881338200997760 ) ) ;
#8986=ADVANCED_FACE ( 'NONE', ( #3057 ), #13930, .T. ) ;
#8988=CARTESIAN_POINT ( 'NONE',  ( 2.606462025418759598, 26.80070150627962633, -17.97639020990277459 ) ) ;
#8992=ORIENTED_EDGE ( 'NONE', *, *, #10903, .F. ) ;
#8993=DIRECTION ( 'NONE',  ( -1.000000000000000000, -0.000000000000000000, -0.000000000000000000 ) ) ;
#8998=AXIS2_PLACEMENT_3D ( 'NONE', #22848, #14681, #15191 ) ;
#8999=EDGE_CURVE ( 'NONE', #21282, #17861, #15791, .T. ) ;
#9012=ORIENTED_EDGE ( 'NONE', *, *, #33578, .F. ) ;
#9017=DIRECTION ( 'NONE',  ( -1.000000000000000000, -0.000000000000000000, -0.000000000000000000 ) ) ;
#9019=CARTESIAN_POINT ( 'NONE',  ( 0.000000000000000000, -20.35927063852789232, -22.08513060777193004 ) ) ;
#9023=CARTESIAN_POINT ( 'NONE',  ( 0.07098932867738322328, 28.92461259213117586, -12.95806963937394762 ) ) ;
#9031=ORIENTED_EDGE ( 'NONE', *, *, #33228, .F. ) ;
#9032=CARTESIAN_POINT ( 'NONE',  ( 7.647434771771126672E-16, -7.837340408380152112, 29.64303704467396017 ) ) ;
#9040=DIRECTION ( 'NONE',  ( -1.000000000000000000, -0.000000000000000000, 0.000000000000000000 ) ) ;
#9043=DIRECTION ( 'NONE',  ( -1.000000000000000000, -0.000000000000000000, -0.000000000000000000 ) ) ;
#9045=CARTESIAN_POINT ( 'NONE',  ( 2.719051661423419475, -31.66307346108433052, 1.400387680933883328 ) ) ;
#9047=DIRECTION ( 'NONE',  ( 0.000000000000000000, 0.000000000000000000, 1.000000000000000000 ) ) ;
#9054=DIRECTION ( 'NONE',  ( -1.000000000000000000, -0.000000000000000000, -0.000000000000000000 ) ) ;
#9055=AXIS2_PLACEMENT_3D ( 'NONE', #19442, #5884, #24574 ) ;
#9056=CARTESIAN_POINT ( 'NONE',  ( 0.006871054653494480455, 14.58967697705840827, -27.20420702726686102 ) ) ;
#9072=DIRECTION ( 'NONE',  ( -1.000000000000000000, 0.000000000000000000, -0.000000000000000000 ) ) ;
#9079=ORIENTED_EDGE ( 'NONE', *, *, #8929, .F. ) ;
#9083=VERTEX_POINT ( 'NONE', #23332 ) ;
#9087=DIRECTION ( 'NONE',  ( -1.000000000000000000, -0.000000000000000000, -0.000000000000000000 ) ) ;
#9095=CARTESIAN_POINT ( 'NONE',  ( 2.789999999999999147, -29.63162325403014208, -6.967017504692083918 ) ) ;
#9102=EDGE_LOOP ( 'NONE', ( #8079, #32276, #3620, #6862, #5560, #12250, #19867, #26518 ) ) ;
#9103=DIRECTION ( 'NONE',  ( -1.000000000000000000, 0.000000000000000000, -0.000000000000000000 ) ) ;
#9112=CARTESIAN_POINT ( 'NONE',  ( 0.5248941919440579529, -23.79505697368676209, 23.40952781232645918 ) ) ;
#9114=CARTESIAN_POINT ( 'NONE',  ( -5.210000000000000853, 0.000000000000000000, 0.000000000000000000 ) ) ;
#9115=CARTESIAN_POINT ( 'NONE',  ( 0.006871166293030922176, 11.66139262930058962, 28.58215465626868834 ) ) ;
#9118=ORIENTED_EDGE ( 'NONE', *, *, #11509, .T. ) ;
#9138=DIRECTION ( 'NONE',  ( 1.000000000000000000, 0.000000000000000000, -0.000000000000000000 ) ) ;
#9143=EDGE_LOOP ( 'NONE', ( #11380, #17826, #25441, #7077, #7234, #9240 ) ) ;
#9144=CARTESIAN_POINT ( 'NONE',  ( 0.5248942741096497278, -32.12939361471808297, 9.050569439367455615 ) ) ;
#9145=CARTESIAN_POINT ( 'NONE',  ( 0.000000000000000000, 23.53611639059741378, -19.35207786518964213 ) ) ;
#9146=ADVANCED_FACE ( 'NONE', ( #26524, #12664 ), #10331, .F. ) ;
#9148=ADVANCED_FACE ( 'NONE', ( #4976 ), #7650, .F. ) ;
#9154=CARTESIAN_POINT ( 'NONE',  ( 2.789999999999999147, 12.39602498911182593, -27.80127684205855942 ) ) ;
#9155=B_SPLINE_CURVE_WITH_KNOTS ( 'NONE', 3,
 ( #30358, #13748, #16260, #24769, #5367, #10559 ),
 .UNSPECIFIED., .F., .F.,
 ( 4, 2, 4 ),
 ( 4.404817204422397961E-07, 0.001874269756547598462, 0.003748099031374754753 ),
 .UNSPECIFIED. ) ;
#9162=ORIENTED_EDGE ( 'NONE', *, *, #3950, .F. ) ;
#9167=CIRCLE ( 'NONE', #22230, 30.47050528711511674 ) ;
#9171=ORIENTED_EDGE ( 'NONE', *, *, #8835, .T. ) ;
#9175=CYLINDRICAL_SURFACE ( 'NONE', #31765, 2.525000000000001243 ) ;
#9187=DIRECTION ( 'NONE',  ( -1.000000000000000000, 0.000000000000000000, 0.000000000000000000 ) ) ;
#9192=B_SPLINE_CURVE_WITH_KNOTS ( 'NONE', 3,
 ( #31787, #17952, #6871, #4376 ),
 .UNSPECIFIED., .F., .F.,
 ( 4, 4 ),
 ( 2.702373194995081723E-07, 0.0006880065385067430078 ),
 .UNSPECIFIED. ) ;
#9222=VERTEX_POINT ( 'NONE', #4446 ) ;
#9224=ORIENTED_EDGE ( 'NONE', *, *, #34025, .F. ) ;
#9225=EDGE_LOOP ( 'NONE', ( #25932, #27080, #20555, #24426, #29238, #22489 ) ) ;
#9228=CIRCLE ( 'NONE', #33101, 2.525000000000001688 ) ;
#9231=CIRCLE ( 'NONE', #7510, 2.525000000000002132 ) ;
#9240=ORIENTED_EDGE ( 'NONE', *, *, #20397, .T. ) ;
#9242=ORIENTED_EDGE ( 'NONE', *, *, #14817, .T. ) ;
#9250=DIRECTION ( 'NONE',  ( 0.000000000000000000, 0.000000000000000000, -1.000000000000000000 ) ) ;
#9272=ORIENTED_EDGE ( 'NONE', *, *, #7902, .T. ) ;
#9274=EDGE_CURVE ( 'NONE', #3106, #26431, #32831, .T. ) ;
#9289=CARTESIAN_POINT ( 'NONE',  ( 0.7561992213566378629, 33.71011734938328175, 3.723857881850638041 ) ) ;
#9293=CARTESIAN_POINT ( 'NONE',  ( 0.07098926918644703210, 12.21472555652512426, -29.24628546289449105 ) ) ;
#9301=ORIENTED_EDGE ( 'NONE', *, *, #4562, .F. ) ;
#9304=VECTOR ( 'NONE', #34457, 1000.000000000000000 ) ;
#9306=ORIENTED_EDGE ( 'NONE', *, *, #34407, .T. ) ;
#9309=ORIENTED_EDGE ( 'NONE', *, *, #12190, .T. ) ;
#9314=CARTESIAN_POINT ( 'NONE',  ( -8.323328165997453710E-14, 29.09328061627312678, -9.684256520155496872 ) ) ;
#9316=VERTEX_POINT ( 'NONE', #27754 ) ;
#9320=CARTESIAN_POINT ( 'NONE',  ( 2.789999999999999147, 28.95078156989557527, 9.502838467758159879 ) ) ;
#9325=CARTESIAN_POINT ( 'NONE',  ( 2.789999999999999147, -27.53147453683415335, -13.05640081644869532 ) ) ;
#9343=CARTESIAN_POINT ( 'NONE',  ( 2.789999999999999147, 11.30192140231272191, -28.29696565125058072 ) ) ;
#9347=VERTEX_POINT ( 'NONE', #32557 ) ;
#9348=EDGE_CURVE ( 'NONE', #13256, #32232, #23194, .T. ) ;
#9352=ORIENTED_EDGE ( 'NONE', *, *, #14795, .F. ) ;
#9353=B_SPLINE_CURVE_WITH_KNOTS ( 'NONE', 3,
 ( #9738, #31446, #28954, #29127 ),
 .UNSPECIFIED., .F., .F.,
 ( 4, 4 ),
 ( 0.005298612564832102384, 0.005985477723952492904 ),
 .UNSPECIFIED. ) ;
#9357=ADVANCED_FACE ( 'NONE', ( #27403 ), #21889, .T. ) ;
#9359=CARTESIAN_POINT ( 'NONE',  ( 1.749999999999999778, 22.14447232807506438, 26.34405054495565679 ) ) ;
#9362=CYLINDRICAL_SURFACE ( 'NONE', #14565, 16.19999999999999929 ) ;
#9381=ORIENTED_EDGE ( 'NONE', *, *, #24609, .T. ) ;
#9384=EDGE_CURVE ( 'NONE', #15134, #32629, #7836, .T. ) ;
#9386=EDGE_LOOP ( 'NONE', ( #27120, #12237, #4504, #3154, #6143, #23618 ) ) ;
#9388=CIRCLE ( 'NONE', #21321, 2.525000000000002576 ) ;
#9389=LINE ( 'NONE', #20250, #15981 ) ;
#9390=EDGE_CURVE ( 'NONE', #3106, #13445, #8452, .T. ) ;
#9397=AXIS2_PLACEMENT_3D ( 'NONE', #31731, #29061, #7339 ) ;
#9410=ORIENTED_EDGE ( 'NONE', *, *, #34407, .F. ) ;
#9422=ORIENTED_EDGE ( 'NONE', *, *, #5872, .F. ) ;
#9427=VERTEX_POINT ( 'NONE', #3888 ) ;
#9430=ORIENTED_EDGE ( 'NONE', *, *, #20060, .F. ) ;
#9433=CARTESIAN_POINT ( 'NONE',  ( 2.765921099433441110, 14.63235270440936731, 27.43224275967444470 ) ) ;
#9440=VERTEX_POINT ( 'NONE', #17464 ) ;
#9445=VECTOR ( 'NONE', #9899, 1000.000000000000000 ) ;
#9450=EDGE_CURVE ( 'NONE', #1617, #24520, #15292, .T. ) ;
#9460=DIRECTION ( 'NONE',  ( 0.000000000000000000, 0.6845471059286788451, 0.7289686274214207673 ) ) ;
#9462=DIRECTION ( 'NONE',  ( -1.000000000000000000, 0.000000000000000000, -0.000000000000000000 ) ) ;
#9463=VERTEX_POINT ( 'NONE', #33273 ) ;
#9467=CIRCLE ( 'NONE', #2642, 2.525000000000001243 ) ;
#9469=CARTESIAN_POINT ( 'NONE',  ( 0.000000000000000000, -14.75935258146395412, -26.65732927035534416 ) ) ;
#9470=CARTESIAN_POINT ( 'NONE',  ( 0.02407890056655564992, 31.00221527374952046, 2.344426712874309260 ) ) ;
#9474=CARTESIAN_POINT ( 'NONE',  ( 2.589916064955228858, 29.62776403357759492, 13.00174666746595342 ) ) ;
#9477=CARTESIAN_POINT ( 'NONE',  ( 0.1859802913914470612, -27.68787216339148571, -16.59794162419619568 ) ) ;
#9488=EDGE_LOOP ( 'NONE', ( #29837, #9906, #21153, #12648, #15072, #5387 ) ) ;
#9511=CARTESIAN_POINT ( 'NONE',  ( 0.02407890056655695096, -26.45933846664182099, -16.32596387352474565 ) ) ;
#9516=DIRECTION ( 'NONE',  ( -1.000000000000000000, -0.000000000000000000, -0.000000000000000000 ) ) ;
#9520=CARTESIAN_POINT ( 'NONE',  ( 0.7564103440434756243, -2.658578268447333581, 33.81118535743536313 ) ) ;
#9534=CARTESIAN_POINT ( 'NONE',  ( 0.7564103432032210916, -18.61839266759128009, 28.34818773854056673 ) ) ;
#9542=EDGE_CURVE ( 'NONE', #14486, #18246, #33023, .T. ) ;
#9544=DIRECTION ( 'NONE',  ( 0.000000000000000000, -0.9980267284282717810, 0.06279051952931077873 ) ) ;
#9561=ORIENTED_EDGE ( 'NONE', *, *, #12159, .T. ) ;
#9575=CARTESIAN_POINT ( 'NONE',  ( 1.040000000000000258, 22.14447232807544452, -26.34405054495532639 ) ) ;
#9579=CARTESIAN_POINT ( 'NONE',  ( -10.00000000000000000, 0.000000000000000000, 0.000000000000000000 ) ) ;
#9587=CARTESIAN_POINT ( 'NONE',  ( 0.02407890056655738464, 26.03801215795517621, 16.98986790278620873 ) ) ;
#9593=CARTESIAN_POINT ( 'NONE',  ( 2.789999999999999147, -25.77598557799237255, -16.24962337825830616 ) ) ;
#9597=ORIENTED_EDGE ( 'NONE', *, *, #11078, .T. ) ;
#9599=AXIS2_PLACEMENT_3D ( 'NONE', #11957, #20138, #25630 ) ;
#9604=CARTESIAN_POINT ( 'NONE',  ( 0.02407890056655911937, -15.32140196853734970, -27.05343472113007763 ) ) ;
#9609=CARTESIAN_POINT ( 'NONE',  ( 0.006871061880576827090, -0.3206953221633991324, -30.86785892350566129 ) ) ;
#9626=ORIENTED_EDGE ( 'NONE', *, *, #18110, .T. ) ;
#9627=DIRECTION ( 'NONE',  ( -1.000000000000000000, -0.000000000000000000, 0.000000000000000000 ) ) ;
#9628=CARTESIAN_POINT ( 'NONE',  ( 2.789999999999999147, -15.78270255339054451, -26.02842157509105547 ) ) ;
#9629=DIRECTION ( 'NONE',  ( 0.000000000000000000, 0.000000000000000000, 1.000000000000000000 ) ) ;
#9635=CARTESIAN_POINT ( 'NONE',  ( 1.040000000000003810, -2.430610048905784915, -34.32897884578301984 ) ) ;
#9637=EDGE_CURVE ( 'NONE', #32232, #2295, #7627, .T. ) ;
#9638=CARTESIAN_POINT ( 'NONE',  ( 2.033800774102392683, 33.57713782924216872, 4.776499238012976711 ) ) ;
#9639=CARTESIAN_POINT ( 'NONE',  ( 50.00050000000000239, 12.80000000000000071, -3.000000000000000000 ) ) ;
#9648=ORIENTED_EDGE ( 'NONE', *, *, #29791, .F. ) ;
#9665=LINE ( 'NONE', #31377, #4037 ) ;
#9675=AXIS2_PLACEMENT_3D ( 'NONE', #20472, #6758, #14448 ) ;
#9677=CARTESIAN_POINT ( 'NONE',  ( 1.394999999999999574, 21.72796464722008380, 26.68861566460903489 ) ) ;
#9680=CARTESIAN_POINT ( 'NONE',  ( 2.765921099433441999, -0.3931553186915530129, 31.08824725498900321 ) ) ;
#9689=ORIENTED_EDGE ( 'NONE', *, *, #21684, .F. ) ;
#9703=DIRECTION ( 'NONE',  ( 0.000000000000000000, 0.000000000000000000, 1.000000000000000000 ) ) ;
#9708=FACE_OUTER_BOUND ( 'NONE', #34410, .T. ) ;
#9715=FACE_OUTER_BOUND ( 'NONE', #34562, .T. ) ;
#9719=AXIS2_PLACEMENT_3D ( 'NONE', #6506, #17408, #28237 ) ;
#9738=CARTESIAN_POINT ( 'NONE',  ( 2.789999999999999147, -0.09145294252654824485, -30.47036804522408460 ) ) ;
#9740=VECTOR ( 'NONE', #7121, 1000.000000000000000 ) ;
#9744=CARTESIAN_POINT ( 'NONE',  ( 1.040000000000002256, 27.68252950111368094, -20.44661865013457813 ) ) ;
#9760=ORIENTED_EDGE ( 'NONE', *, *, #5076, .F. ) ;
#9767=DIRECTION ( 'NONE',  ( -1.000000000000000000, 0.000000000000000000, 0.000000000000000000 ) ) ;
#9768=EDGE_CURVE ( 'NONE', #31064, #31497, #15734, .T. ) ;
#9775=ORIENTED_EDGE ( 'NONE', *, *, #6327, .F. ) ;
#9789=ADVANCED_FACE ( 'NONE', ( #11593 ), #8905, .T. ) ;
#9793=ORIENTED_EDGE ( 'NONE', *, *, #24341, .F. ) ;
#9798=DIRECTION ( 'NONE',  ( -1.000000000000000000, -0.000000000000000000, 0.000000000000000000 ) ) ;
#9806=CARTESIAN_POINT ( 'NONE',  ( 0.000000000000000000, 29.94779062842797401, -5.619744560738746841 ) ) ;
#9809=VECTOR ( 'NONE', #25964, 1000.000000000000000 ) ;
#9815=VERTEX_POINT ( 'NONE', #5866 ) ;
#9831=EDGE_LOOP ( 'NONE', ( #31530, #28247, #28011, #7008 ) ) ;
#9836=CARTESIAN_POINT ( 'NONE',  ( 0.02407890056655738464, -27.96208973699912548, 13.59246946040177129 ) ) ;
#9839=CARTESIAN_POINT ( 'NONE',  ( 2.790000000000081748, 25.77088461036980505, 16.61521147790390884 ) ) ;
#9840=VERTEX_POINT ( 'NONE', #24916 ) ;
#9845=EDGE_CURVE ( 'NONE', #23220, #32949, #6581, .T. ) ;
#9852=DIRECTION ( 'NONE',  ( -1.000000000000000000, -0.000000000000000000, -0.000000000000000000 ) ) ;
#9853=ORIENTED_EDGE ( 'NONE', *, *, #15855, .F. ) ;
#9860=AXIS2_PLACEMENT_3D ( 'NONE', #25826, #26351, #31852 ) ;
#9865=VERTEX_POINT ( 'NONE', #16947 ) ;
#9879=CARTESIAN_POINT ( 'NONE',  ( 0.006892406498510319189, -30.26126365281900732, -6.099214421700076549 ) ) ;
#9881=CARTESIAN_POINT ( 'NONE',  ( 2.783128942071183332, -30.82708482934415528, 1.618146408792505708 ) ) ;
#9887=AXIS2_PLACEMENT_3D ( 'NONE', #48, #13413, #27099 ) ;
#9889=CARTESIAN_POINT ( 'NONE',  ( 0.000000000000000000, -20.92506858792774338, 22.14933852381670221 ) ) ;
#9890=ORIENTED_EDGE ( 'NONE', *, *, #8713, .F. ) ;
#9893=CARTESIAN_POINT ( 'NONE',  ( 2.789999999999999147, -26.45933846664205902, 16.32596387352436551 ) ) ;
#9898=CARTESIAN_POINT ( 'NONE',  ( -5.210000000000000853, 0.000000000000000000, 0.000000000000000000 ) ) ;
#9899=DIRECTION ( 'NONE',  ( -1.000000000000000000, -0.000000000000000000, 0.000000000000000000 ) ) ;
#9906=ORIENTED_EDGE ( 'NONE', *, *, #24004, .F. ) ;
#9917=EDGE_CURVE ( 'NONE', #29345, #13451, #11051, .T. ) ;
#9923=ORIENTED_EDGE ( 'NONE', *, *, #34707, .T. ) ;
#9929=VECTOR ( 'NONE', #8595, 1000.000000000000000 ) ;
#9936=CARTESIAN_POINT ( 'NONE',  ( 1.749999999999999778, 32.09669216789236401, 12.41728656686386500 ) ) ;
#9938=CARTESIAN_POINT ( 'NONE',  ( 0.02407890056655911937, -15.32140196853734970, -27.05343472113007763 ) ) ;
#9941=STYLED_ITEM('',(#35289),#33586);
#9946=AXIS2_PLACEMENT_3D ( 'NONE', #3865, #6359, #1727 ) ;
#9953=VERTEX_POINT ( 'NONE', #17998 ) ;
#9974=CARTESIAN_POINT ( 'NONE',  ( 0.006892381195637166565, 30.78707849925352491, 2.258378142202824179 ) ) ;
#9975=CARTESIAN_POINT ( 'NONE',  ( -8.204391965473290931E-14, -21.14989222980530670, -22.20103112977927395 ) ) ;
#9981=CARTESIAN_POINT ( 'NONE',  ( 0.000000000000000000, 0.000000000000000000, 0.000000000000000000 ) ) ;
#9982=EDGE_CURVE ( 'NONE', #5461, #19524, #32225, .T. ) ;
#9986=CARTESIAN_POINT ( 'NONE',  ( 2.789999999999999147, 7.489092610871509237, -29.53582882395378562 ) ) ;
#9989=CARTESIAN_POINT ( 'NONE',  ( 1.040000000000001590, -30.02688531850382958, -16.81585001935613022 ) ) ;
#10006=DIRECTION ( 'NONE',  ( -1.000000000000000000, -0.000000000000000000, -0.000000000000000000 ) ) ;
#10013=DIRECTION ( 'NONE',  ( -1.000000000000000000, -0.000000000000000000, -0.000000000000000000 ) ) ;
#10014=CIRCLE ( 'NONE', #16851, 2.525000000000001688 ) ;
#10015=CARTESIAN_POINT ( 'NONE',  ( 0.02407890056655651728, 29.44518845714764765, 9.980709654879525772 ) ) ;
#10018=CARTESIAN_POINT ( 'NONE',  ( 2.783128888645070464, 25.89075856630346095, 16.81059844634668821 ) ) ;
#10029=CIRCLE ( 'NONE', #11183, 2.525000000000001688 ) ;
#10036=EDGE_CURVE ( 'NONE', #14959, #13078, #8420, .T. ) ;
#10046=CARTESIAN_POINT ( 'NONE',  ( 2.789999999999999147, -1.291199951813412738, 30.41225463960052267 ) ) ;
#10064=ORIENTED_EDGE ( 'NONE', *, *, #10081, .T. ) ;
#10081=EDGE_CURVE ( 'NONE', #4047, #6854, #16018, .T. ) ;
#10088=ORIENTED_EDGE ( 'NONE', *, *, #6083, .F. ) ;
#10092=CARTESIAN_POINT ( 'NONE',  ( 1.040000000000000924, -10.37741591188871482, -32.81304455236878681 ) ) ;
#10108=ORIENTED_EDGE ( 'NONE', *, *, #5899, .F. ) ;
#10109=CARTESIAN_POINT ( 'NONE',  ( 2.604019732385639330, 30.43784769162271076, 10.75394592869520594 ) ) ;
#10116=CARTESIAN_POINT ( 'NONE',  ( 8.000000000000000000, 0.000000000000000000, 0.000000000000000000 ) ) ;
#10117=EDGE_CURVE ( 'NONE', #31064, #14153, #35057, .T. ) ;
#10118=CARTESIAN_POINT ( 'NONE',  ( 2.790000000000083080, 14.57875922523665047, 26.97523840778890047 ) ) ;
#10125=EDGE_CURVE ( 'NONE', #14449, #25806, #689, .T. ) ;
#10132=EDGE_CURVE ( 'NONE', #30042, #527, #25858, .T. ) ;
#10144=EDGE_LOOP ( 'NONE', ( #8150, #5363, #7712, #19761 ) ) ;
#10147=ORIENTED_EDGE ( 'NONE', *, *, #20197, .T. ) ;
#10161=CARTESIAN_POINT ( 'NONE',  ( 2.765921099433443775, -26.45933846664182099, -16.32596387352474565 ) ) ;
#10165=DIRECTION ( 'NONE',  ( -1.000000000000000000, -0.000000000000000000, -0.000000000000000000 ) ) ;
#10167=EDGE_CURVE ( 'NONE', #9463, #16548, #22666, .T. ) ;
#10168=VECTOR ( 'NONE', #9187, 1000.000000000000000 ) ;
#10169=ORIENTED_EDGE ( 'NONE', *, *, #25348, .F. ) ;
#10177=DIRECTION ( 'NONE',  ( -1.000000000000000000, -0.000000000000000000, -0.000000000000000000 ) ) ;
#10181=EDGE_LOOP ( 'NONE', ( #13138, #25064, #16918, #21728 ) ) ;
#10188=CARTESIAN_POINT ( 'NONE',  ( 0.000000000000000000, 28.95078156989571738, -9.502838467757779739 ) ) ;
#10218=VERTEX_POINT ( 'NONE', #30754 ) ;
#10219=CARTESIAN_POINT ( 'NONE',  ( 2.783128948903274669, -29.45617853245872553, 9.233693611949725266 ) ) ;
#10227=ORIENTED_EDGE ( 'NONE', *, *, #24124, .T. ) ;
#10229=CARTESIAN_POINT ( 'NONE',  ( 2.789999999999999147, 0.000000000000000000, 0.000000000000000000 ) ) ;
#10233=DIRECTION ( 'NONE',  ( 1.000000000000000000, -0.000000000000000000, -0.000000000000000000 ) ) ;
#10236=VECTOR ( 'NONE', #16379, 1000.000000000000000 ) ;
#10241=DIRECTION ( 'NONE',  ( 1.000000000000000000, -0.000000000000000000, -0.000000000000000000 ) ) ;
#10256=ORIENTED_EDGE ( 'NONE', *, *, #3516, .T. ) ;
#10268=VERTEX_POINT ( 'NONE', #10092 ) ;
#10274=CARTESIAN_POINT ( 'NONE',  ( 2.765921099433441999, 7.350529080603541487, 30.20932655202940254 ) ) ;
#10281=CIRCLE ( 'NONE', #27318, 2.525000000000001243 ) ;
#10283=CARTESIAN_POINT ( 'NONE',  ( 1.749999999999999778, 0.000000000000000000, 0.000000000000000000 ) ) ;
#10287=CARTESIAN_POINT ( 'NONE',  ( 2.789999999999999147, 30.40449935640660684, -2.004522720844263084 ) ) ;
#10304=VECTOR ( 'NONE', #11738, 1000.000000000000000 ) ;
#10310=ORIENTED_EDGE ( 'NONE', *, *, #681, .T. ) ;
#10325=DIRECTION ( 'NONE',  ( 0.000000000000000000, 0.000000000000000000, 1.000000000000000000 ) ) ;
#10326=LINE ( 'NONE', #24194, #22242 ) ;
#10331=PLANE ( 'NONE',  #28822 ) ;
#10340=VERTEX_POINT ( 'NONE', #28438 ) ;
#10352=CARTESIAN_POINT ( 'NONE',  ( 2.719051665953501562, 21.26181984063893893, 23.50417665062026273 ) ) ;
#10365=CARTESIAN_POINT ( 'NONE',  ( 2.789999999999999147, -29.00730259674831757, -9.328884633909261481 ) ) ;
#10378=CARTESIAN_POINT ( 'NONE',  ( 2.789999999999999147, 31.93991905851385837, 0.000000000000000000 ) ) ;
#10388=B_SPLINE_CURVE_WITH_KNOTS ( 'NONE', 3,
 ( #11160, #32849, #27687, #24471, #5783, #27330 ),
 .UNSPECIFIED., .F., .F.,
 ( 4, 2, 4 ),
 ( 2.248981763129426848E-07, 0.001873423219693743378, 0.003746621541211173859 ),
 .UNSPECIFIED. ) ;
#10394=CARTESIAN_POINT ( 'NONE',  ( 2.765921099435497243, 28.29688452313399338, 12.88099432405614309 ) ) ;
#10401=ORIENTED_EDGE ( 'NONE', *, *, #9917, .F. ) ;
#10402=CARTESIAN_POINT ( 'NONE',  ( 0.1835379100341435199, -28.84240889917319706, -14.47562221546578343 ) ) ;
#10405=EDGE_CURVE ( 'NONE', #25011, #5512, #8473, .T. ) ;
#10409=CARTESIAN_POINT ( 'NONE',  ( 2.789999999999999147, -14.75935258146429341, 26.65732927035513811 ) ) ;
#10412=EDGE_CURVE ( 'NONE', #31468, #5130, #10546, .T. ) ;
#10414=ORIENTED_EDGE ( 'NONE', *, *, #26467, .F. ) ;
#10420=DIRECTION ( 'NONE',  ( -1.000000000000000000, -0.000000000000000000, -0.000000000000000000 ) ) ;
#10426=CARTESIAN_POINT ( 'NONE',  ( -1.250599194761023927E-17, -3.625355760179439280, -30.44651458975035396 ) ) ;
#10449=DIRECTION ( 'NONE',  ( -1.000000000000000000, -0.000000000000000000, -0.000000000000000000 ) ) ;
#10450=ORIENTED_EDGE ( 'NONE', *, *, #34381, .T. ) ;
#10454=ORIENTED_EDGE ( 'NONE', *, *, #30479, .T. ) ;
#10456=B_SPLINE_CURVE_WITH_KNOTS ( 'NONE', 3,
 ( #17890, #30003, #21807, #10960, #8107, #16492 ),
 .UNSPECIFIED., .F., .F.,
 ( 4, 2, 4 ),
 ( 4.404817080687146341E-07, 0.001874269664496245377, 0.003748098847284421931 ),
 .UNSPECIFIED. ) ;
#10461=ADVANCED_FACE ( 'NONE', ( #25007 ), #9175, .F. ) ;
#10462=ADVANCED_FACE ( 'NONE', ( #642 ), #19342, .T. ) ;
#10466=CARTESIAN_POINT ( 'NONE',  ( 1.395000000000002238, 34.10861917999622506, -4.581348211831717698 ) ) ;
#10467=CARTESIAN_POINT ( 'NONE',  ( -8.216995152909043008E-14, -30.07763130521195549, 5.961539033704580604 ) ) ;
#10468=EDGE_CURVE ( 'NONE', #7115, #21282, #3648, .T. ) ;
#10471=AXIS2_PLACEMENT_3D ( 'NONE', #294, #14362, #19519 ) ;
#10478=VECTOR ( 'NONE', #7299, 1000.000000000000000 ) ;
#10497=EDGE_CURVE ( 'NONE', #18208, #33010, #8836, .T. ) ;
#10502=CARTESIAN_POINT ( 'NONE',  ( 2.719010670160031395, -11.11630839801615167, 29.68118041677924168 ) ) ;
#10504=VERTEX_POINT ( 'NONE', #33382 ) ;
#10508=VERTEX_POINT ( 'NONE', #11687 ) ;
#10513=CARTESIAN_POINT ( 'NONE',  ( 2.789999999999999147, -22.61000311763331183, -20.38038735157106274 ) ) ;
#10524=CARTESIAN_POINT ( 'NONE',  ( 1.040000000000000924, 0.000000000000000000, 0.000000000000000000 ) ) ;
#10525=LINE ( 'NONE', #7841, #24025 ) ;
#10526=B_SPLINE_CURVE_WITH_KNOTS ( 'NONE', 3,
 ( #7658, #29212, #26707, #34724 ),
 .UNSPECIFIED., .F., .F.,
 ( 4, 4 ),
 ( 0.005298612564832130140, 0.005985477723952354126 ),
 .UNSPECIFIED. ) ;
#10529=CARTESIAN_POINT ( 'NONE',  ( 0.000000000000000000, -14.75935258146395412, -26.65732927035534416 ) ) ;
#10532=AXIS2_PLACEMENT_3D ( 'NONE', #320, #29207, #23855 ) ;
#10537=EDGE_LOOP ( 'NONE', ( #4655, #432, #13292, #24080 ) ) ;
#10545=CARTESIAN_POINT ( 'NONE',  ( 1.040000000000000924, 0.000000000000000000, 0.000000000000000000 ) ) ;
#10546=B_SPLINE_CURVE_WITH_KNOTS ( 'NONE', 3,
 ( #21819, #32675, #4909, #7761 ),
 .UNSPECIFIED., .F., .F.,
 ( 4, 4 ),
 ( 0.005298361175080958108, 0.005985229640890899275 ),
 .UNSPECIFIED. ) ;
#10547=ORIENTED_EDGE ( 'NONE', *, *, #8852, .T. ) ;
#10551=DIRECTION ( 'NONE',  ( -1.000000000000000000, -0.000000000000000000, -0.000000000000000000 ) ) ;
#10552=VECTOR ( 'NONE', #22551, 1000.000000000000000 ) ;
#10559=CARTESIAN_POINT ( 'NONE',  ( 2.765921099433441999, -15.32140196853772984, 27.05343472112986092 ) ) ;
#10564=CARTESIAN_POINT ( 'NONE',  ( 0.02407890056655695096, -23.70329957282599764, 20.11932597908820242 ) ) ;
#10575=ORIENTED_EDGE ( 'NONE', *, *, #19026, .T. ) ;
#10590=CARTESIAN_POINT ( 'NONE',  ( 1.749999999999999778, -30.02688531850381182, -16.81585001935615153 ) ) ;
#10597=ORIENTED_EDGE ( 'NONE', *, *, #29830, .F. ) ;
#10606=ORIENTED_EDGE ( 'NONE', *, *, #7697, .F. ) ;
#10610=EDGE_LOOP ( 'NONE', ( #19690, #26799, #25086, #13853 ) ) ;
#10611=CARTESIAN_POINT ( 'NONE',  ( 0.02407890056655521624, 28.29688452313399338, 12.88099432405614309 ) ) ;
#10618=AXIS2_PLACEMENT_3D ( 'NONE', #16789, #33485, #22986 ) ;
#10636=EDGE_CURVE ( 'NONE', #9815, #27727, #12219, .T. ) ;
#10638=DIRECTION ( 'NONE',  ( 1.000000000000000000, -0.000000000000000000, -0.000000000000000000 ) ) ;
#10639=DIRECTION ( 'NONE',  ( -1.000000000000000000, -0.000000000000000000, 0.000000000000000000 ) ) ;
#10660=DIRECTION ( 'NONE',  ( -1.000000000000000000, -0.000000000000000000, -0.000000000000000000 ) ) ;
#10661=B_SPLINE_CURVE_WITH_KNOTS ( 'NONE', 3,
 ( #13323, #18670, #35036, #18837, #2267, #15994 ),
 .UNSPECIFIED., .F., .F.,
 ( 4, 2, 4 ),
 ( 4.404817005620078000E-07, 0.001874269608671721770, 0.003748098735642881301 ),
 .UNSPECIFIED. ) ;
#10663=VERTEX_POINT ( 'NONE', #4822 ) ;
#10664=TOROIDAL_SURFACE ( 'NONE', #23742, 30.47050528711512030, 8.000000000000000000 ) ;
#10671=DIRECTION ( 'NONE',  ( 0.000000000000000000, 0.000000000000000000, 1.000000000000000000 ) ) ;
#10679=ADVANCED_FACE ( 'NONE', ( #18385 ), #21563, .T. ) ;
#10687=EDGE_CURVE ( 'NONE', #31399, #9316, #24509, .T. ) ;
#10688=CARTESIAN_POINT ( 'NONE',  ( 2.790000000000081748, -3.624739946993785988, -30.44774159452265039 ) ) ;
#10694=CYLINDRICAL_SURFACE ( 'NONE', #27170, 16.19999999999999574 ) ;
#10701=LINE ( 'NONE', #5333, #11581 ) ;
#10725=AXIS2_PLACEMENT_3D ( 'NONE', #26330, #1604, #4958 ) ;
#10727=DIRECTION ( 'NONE',  ( 0.000000000000000000, 0.000000000000000000, 1.000000000000000000 ) ) ;
#10728=B_SPLINE_CURVE_WITH_KNOTS ( 'NONE', 3,
 ( #23945, #18982, #21806, #32310 ),
 .UNSPECIFIED., .F., .F.,
 ( 4, 4 ),
 ( 2.250995564674898728E-07, 0.0006879610227482087616 ),
 .UNSPECIFIED. ) ;
#10729=CARTESIAN_POINT ( 'NONE',  ( -5.210000000000000853, 0.000000000000000000, 0.000000000000000000 ) ) ;
#10735=DIRECTION ( 'NONE',  ( 0.000000000000000000, 0.000000000000000000, 1.000000000000000000 ) ) ;
#10736=CARTESIAN_POINT ( 'NONE',  ( 2.604019705000863993, -30.94574698966636106, 9.190792961030121333 ) ) ;
#10739=CARTESIAN_POINT ( 'NONE',  ( 1.395000000000002238, -2.430610048905781806, -34.32897884578301984 ) ) ;
#10752=B_SPLINE_CURVE_WITH_KNOTS ( 'NONE', 3,
 ( #16729, #2824, #24522, #349 ),
 .UNSPECIFIED., .F., .F.,
 ( 4, 4 ),
 ( 2.042209043309391692E-07, 0.0006879399691688898233 ),
 .UNSPECIFIED. ) ;
#10759=CARTESIAN_POINT ( 'NONE',  ( 2.779215089232839109, 28.09152240582078974, -12.86217335695007868 ) ) ;
#10778=DIRECTION ( 'NONE',  ( -1.000000000000000000, -0.000000000000000000, 0.000000000000000000 ) ) ;
#10806=CARTESIAN_POINT ( 'NONE',  ( 1.749999999999999778, 0.000000000000000000, 0.000000000000000000 ) ) ;
#10824=CARTESIAN_POINT ( 'NONE',  ( 2.783107579261526965, 30.38148214875505104, 5.469007969453682172 ) ) ;
#10831=DIRECTION ( 'NONE',  ( -1.000000000000000000, 0.000000000000000000, -0.000000000000000000 ) ) ;
#10834=VECTOR ( 'NONE', #8126, 1000.000000000000000 ) ;
#10837=ORIENTED_EDGE ( 'NONE', *, *, #15005, .T. ) ;
#10845=AXIS2_PLACEMENT_3D ( 'NONE', #33782, #6883, #9047 ) ;
#10850=FACE_OUTER_BOUND ( 'NONE', #12874, .T. ) ;
#10855=ORIENTED_EDGE ( 'NONE', *, *, #17346, .T. ) ;
#10865=CARTESIAN_POINT ( 'NONE',  ( 2.789999999999999147, 28.29688452313399338, 12.88099432405614309 ) ) ;
#10868=DIRECTION ( 'NONE',  ( 1.000000000000000000, -0.000000000000000000, 0.000000000000000000 ) ) ;
#10871=EDGE_CURVE ( 'NONE', #9463, #18937, #14126, .T. ) ;
#10878=EDGE_CURVE ( 'NONE', #22891, #34395, #7862, .T. ) ;
#10880=DIRECTION ( 'NONE',  ( 0.000000000000000000, 0.000000000000000000, 1.000000000000000000 ) ) ;
#10882=AXIS2_PLACEMENT_3D ( 'NONE', #18330, #20804, #20633 ) ;
#10893=CYLINDRICAL_SURFACE ( 'NONE', #27070, 16.19999999999999574 ) ;
#10899=CIRCLE ( 'NONE', #2930, 30.47050528711511674 ) ;
#10903=EDGE_CURVE ( 'NONE', #12420, #19998, #31494, .T. ) ;
#10904=EDGE_CURVE ( 'NONE', #32472, #6239, #21174, .T. ) ;
#10906=CARTESIAN_POINT ( 'NONE',  ( 1.040000000000002922, 34.17636915695680244, -4.045051921974834208 ) ) ;
#10907=CARTESIAN_POINT ( 'NONE',  ( 2.789999999999999147, 0.000000000000000000, 0.000000000000000000 ) ) ;
#10918=CARTESIAN_POINT ( 'NONE',  ( 2.765921099433443775, -31.05158812718220673, -1.559667679918931738 ) ) ;
#10921=ORIENTED_EDGE ( 'NONE', *, *, #2101, .T. ) ;
#10923=EDGE_CURVE ( 'NONE', #15056, #19998, #34010, .T. ) ;
#10928=CARTESIAN_POINT ( 'NONE',  ( 2.765921099433442443, 20.99477179376825120, 22.93149026599753526 ) ) ;
#10939=CARTESIAN_POINT ( 'NONE',  ( 0.000000000000000000, 0.000000000000000000, 0.000000000000000000 ) ) ;
#10945=PLANE ( 'NONE',  #5216 ) ;
#10947=CARTESIAN_POINT ( 'NONE',  ( 2.789999999999999147, 17.11426446101236820, -26.96776559937708129 ) ) ;
#10954=( GEOMETRIC_REPRESENTATION_CONTEXT ( 3 ) GLOBAL_UNCERTAINTY_ASSIGNED_CONTEXT ( ( #3895 ) ) GLOBAL_UNIT_ASSIGNED_CONTEXT ( ( #25844, #28859, #1630 ) ) REPRESENTATION_CONTEXT ( 'NONE', 'WORKASPACE' ) );
#10960=CARTESIAN_POINT ( 'NONE',  ( 2.604019721411119370, -31.54566302605122630, -6.854274004868179837 ) ) ;
#10962=ORIENTED_EDGE ( 'NONE', *, *, #6299, .F. ) ;
#10987=CARTESIAN_POINT ( 'NONE',  ( 1.039999999999999813, 21.72796464722045684, -26.68861566460872226 ) ) ;
#10991=DIRECTION ( 'NONE',  ( 1.000000000000000000, 0.000000000000000000, 0.000000000000000000 ) ) ;
#11011=ORIENTED_EDGE ( 'NONE', *, *, #26867, .F. ) ;
#11028=B_SPLINE_CURVE_WITH_KNOTS ( 'NONE', 3,
 ( #9806, #4799, #2146, #20671 ),
 .UNSPECIFIED., .F., .F.,
 ( 4, 4 ),
 ( 0.005298484651059805900, 0.005985351487543621660 ),
 .UNSPECIFIED. ) ;
#11032=PRODUCT_DEFINITION_FORMATION_WITH_SPECIFIED_SOURCE ( 'ANY', '', #27382, .NOT_KNOWN. ) ;
#11039=DIRECTION ( 'NONE',  ( -1.000000000000000000, -0.000000000000000000, -0.000000000000000000 ) ) ;
#11040=FACE_OUTER_BOUND ( 'NONE', #34896, .T. ) ;
#11041=CIRCLE ( 'NONE', #12780, 34.41491905851385269 ) ;
#11045=DIRECTION ( 'NONE',  ( 0.000000000000000000, 0.000000000000000000, 1.000000000000000000 ) ) ;
#11050=B_SPLINE_CURVE_WITH_KNOTS ( 'NONE', 3,
 ( #4361, #1537, #31255, #33753 ),
 .UNSPECIFIED., .F., .F.,
 ( 4, 4 ),
 ( 0.005298346101779248009, 0.005985214792935097776 ),
 .UNSPECIFIED. ) ;
#11051=B_SPLINE_CURVE_WITH_KNOTS ( 'NONE', 3,
 ( #4072, #34338, #18341, #28649 ),
 .UNSPECIFIED., .F., .F.,
 ( 4, 4 ),
 ( 0.005298437004852339476, 0.005985304466813749433 ),
 .UNSPECIFIED. ) ;
#11054=B_SPLINE_CURVE_WITH_KNOTS ( 'NONE', 3,
 ( #9889, #31598, #18107, #28931 ),
 .UNSPECIFIED., .F., .F.,
 ( 4, 4 ),
 ( 0.005298355823470672979, 0.005985224365431036052 ),
 .UNSPECIFIED. ) ;
#11064=EDGE_CURVE ( 'NONE', #31361, #6257, #25471, .T. ) ;
#11071=CYLINDRICAL_SURFACE ( 'NONE', #24917, 16.19999999999999574 ) ;
#11078=EDGE_CURVE ( 'NONE', #26400, #28097, #27679, .T. ) ;
#11082=CARTESIAN_POINT ( 'NONE',  ( 1.749999999999999778, 21.72796464722046039, -26.68861566460872226 ) ) ;
#11095=ORIENTED_EDGE ( 'NONE', *, *, #6083, .T. ) ;
#11096=DIRECTION ( 'NONE',  ( 0.000000000000000000, 0.000000000000000000, 1.000000000000000000 ) ) ;
#11102=AXIS2_PLACEMENT_3D ( 'NONE', #13909, #24921, #8553 ) ;
#11107=B_SPLINE_CURVE_WITH_KNOTS ( 'NONE', 3,
 ( #3633, #26403, #21062, #18074 ),
 .UNSPECIFIED., .F., .F.,
 ( 4, 4 ),
 ( 1.992873153269126117E-07, 0.0006879349942371536155 ),
 .UNSPECIFIED. ) ;
#11110=CARTESIAN_POINT ( 'NONE',  ( 0.000000000000000000, -29.00730259674833178, -9.328884633909240165 ) ) ;
#11120=CIRCLE ( 'NONE', #4842, 2.525000000000000355 ) ;
#11128=EDGE_LOOP ( 'NONE', ( #29034, #16237, #26499, #28864 ) ) ;
#11132=CARTESIAN_POINT ( 'NONE',  ( 2.265105725890352861, -32.12939361471795507, -9.050569439367922797 ) ) ;
#11135=ORIENTED_EDGE ( 'NONE', *, *, #11218, .F. ) ;
#11157=CARTESIAN_POINT ( 'NONE',  ( 0.000000000000000000, -3.728217946243090886, 30.24156218513556738 ) ) ;
#11158=CARTESIAN_POINT ( 'NONE',  ( 1.394999999999999574, 34.10861917999616111, 4.581348211832198203 ) ) ;
#11160=CARTESIAN_POINT ( 'NONE',  ( 2.765921099433442887, -21.56796757982795043, -22.39322359481629476 ) ) ;
#11164=CARTESIAN_POINT ( 'NONE',  ( 1.040000000000000924, 0.000000000000000000, 0.000000000000000000 ) ) ;
#11166=DIRECTION ( 'NONE',  ( -1.000000000000000000, -0.000000000000000000, -0.000000000000000000 ) ) ;
#11167=VECTOR ( 'NONE', #34494, 1000.000000000000000 ) ;
#11179=ORIENTED_EDGE ( 'NONE', *, *, #5807, .T. ) ;
#11183=AXIS2_PLACEMENT_3D ( 'NONE', #3917, #14981, #9460 ) ;
#11187=CARTESIAN_POINT ( 'NONE',  ( 2.789999999999999147, -13.59935610937992401, 28.90010281771827039 ) ) ;
#11189=VECTOR ( 'NONE', #10241, 1000.000000000000000 ) ;
#11195=TOROIDAL_SURFACE ( 'NONE', #34485, 30.47050528711511674, 8.000000000000000000 ) ;
#11207=CARTESIAN_POINT ( 'NONE',  ( 2.765921099433441110, -27.96208973699912548, 13.59246946040177129 ) ) ;
#11209=ORIENTED_EDGE ( 'NONE', *, *, #30579, .F. ) ;
#11218=EDGE_CURVE ( 'NONE', #23413, #32949, #8144, .T. ) ;
#11224=DIRECTION ( 'NONE',  ( -1.000000000000000000, 0.000000000000000000, 0.000000000000000000 ) ) ;
#11225=CARTESIAN_POINT ( 'NONE',  ( 0.000000000000000000, 12.80000000000000071, 0.000000000000000000 ) ) ;
#11227=CARTESIAN_POINT ( 'NONE',  ( 2.261199742025449044, -2.866095775113887356, -33.26657006572086317 ) ) ;
#11228=DIRECTION ( 'NONE',  ( 0.000000000000000000, 0.000000000000000000, 1.000000000000000000 ) ) ;
#11248=DIRECTION ( 'NONE',  ( -1.000000000000000000, 0.000000000000000000, 0.000000000000000000 ) ) ;
#11250=ADVANCED_FACE ( 'NONE', ( #25949 ), #14661, .T. ) ;
#11265=EDGE_CURVE ( 'NONE', #939, #30843, #27689, .T. ) ;
#11271=EDGE_CURVE ( 'NONE', #14020, #25735, #11571, .T. ) ;
#11272=DIRECTION ( 'NONE',  ( -1.000000000000000000, 0.000000000000000000, 0.000000000000000000 ) ) ;
#11275=CARTESIAN_POINT ( 'NONE',  ( 0.000000000000000000, 0.000000000000000000, 0.000000000000000000 ) ) ;
#11277=CIRCLE ( 'NONE', #25459, 34.41491905851385269 ) ;
#11287=LINE ( 'NONE', #3080, #9929 ) ;
#11290=VERTEX_POINT ( 'NONE', #33961 ) ;
#11296=CARTESIAN_POINT ( 'NONE',  ( 2.765921099433441999, 7.350529080603541487, 30.20932655202940254 ) ) ;
#11303=FACE_BOUND ( 'NONE', #32281, .T. ) ;
#11315=VECTOR ( 'NONE', #485, 1000.000000000000000 ) ;
#11316=ORIENTED_EDGE ( 'NONE', *, *, #28690, .T. ) ;
#11319=ORIENTED_EDGE ( 'NONE', *, *, #15727, .F. ) ;
#11337=ORIENTED_EDGE ( 'NONE', *, *, #1099, .T. ) ;
#11344=CARTESIAN_POINT ( 'NONE',  ( 0.5288002580638561101, 14.91106968280097078, -29.87539438830504324 ) ) ;
#11348=CYLINDRICAL_SURFACE ( 'NONE', #4329, 16.19999999999999574 ) ;
#11350=DIRECTION ( 'NONE',  ( 0.000000000000000000, 0.000000000000000000, 1.000000000000000000 ) ) ;
#11379=CARTESIAN_POINT ( 'NONE',  ( 1.394999999999999574, -30.02688531850382958, -16.81585001935612667 ) ) ;
#11380=ORIENTED_EDGE ( 'NONE', *, *, #11265, .F. ) ;
#11384=AXIS2_PLACEMENT_3D ( 'NONE', #13558, #18, #10880 ) ;
#11387=CARTESIAN_POINT ( 'NONE',  ( 2.783107605771416804, 29.25821015115265311, -9.843862221887864195 ) ) ;
#11389=CARTESIAN_POINT ( 'NONE',  ( 1.749999999999999778, 0.000000000000000000, 0.000000000000000000 ) ) ;
#11390=CARTESIAN_POINT ( 'NONE',  ( 2.789999999999999147, -31.68806325674609781, 4.003133335385473224 ) ) ;
#11399=VERTEX_POINT ( 'NONE', #27339 ) ;
#11402=AXIS2_PLACEMENT_3D ( 'NONE', #9579, #3695, #22756 ) ;
#11414=FACE_OUTER_BOUND ( 'NONE', #5731, .T. ) ;
#11423=VERTEX_POINT ( 'NONE', #24479 ) ;
#11430=CARTESIAN_POINT ( 'NONE',  ( 2.789999999999999147, -15.32140196853734970, -27.05343472113007763 ) ) ;
#11431=CIRCLE ( 'NONE', #31315, 2.525000000000003020 ) ;
#11433=DIRECTION ( 'NONE',  ( -1.000000000000000000, -0.000000000000000000, -0.000000000000000000 ) ) ;
#11442=ADVANCED_FACE ( 'NONE', ( #24140 ), #13353, .F. ) ;
#11449=VERTEX_POINT ( 'NONE', #26647 ) ;
#11452=ADVANCED_FACE ( 'NONE', ( #32160 ), #2783, .T. ) ;
#11460=EDGE_LOOP ( 'NONE', ( #33162, #34261, #8467, #31279, #117, #1515 ) ) ;
#11463=CARTESIAN_POINT ( 'NONE',  ( 2.765921099433441555, -0.3931553186911057041, -31.08824725498900676 ) ) ;
#11468=ORIENTED_EDGE ( 'NONE', *, *, #11271, .F. ) ;
#11472=CARTESIAN_POINT ( 'NONE',  ( 0.02407890056655825201, -3.506335382740311868, -30.89238256715869468 ) ) ;
#11475=VECTOR ( 'NONE', #31958, 1000.000000000000000 ) ;
#11486=DIRECTION ( 'NONE',  ( 0.000000000000000000, 0.000000000000000000, 1.000000000000000000 ) ) ;
#11488=ORIENTED_EDGE ( 'NONE', *, *, #14919, .F. ) ;
#11499=DIRECTION ( 'NONE',  ( 0.000000000000000000, 0.000000000000000000, 1.000000000000000000 ) ) ;
#11500=ORIENTED_EDGE ( 'NONE', *, *, #26670, .F. ) ;
#11503=EDGE_CURVE ( 'NONE', #34660, #16525, #28234, .T. ) ;
#11505=CARTESIAN_POINT ( 'NONE',  ( 0.02407890056655868569, -17.95514392185398833, -25.38201125280375692 ) ) ;
#11507=EDGE_CURVE ( 'NONE', #7193, #14739, #32814, .T. ) ;
#11509=EDGE_CURVE ( 'NONE', #19421, #32336, #22600, .T. ) ;
#11511=CARTESIAN_POINT ( 'NONE',  ( -6.927285360088501365E-16, 29.09243261715493034, 9.683176917503475423 ) ) ;
#11520=DIRECTION ( 'NONE',  ( -1.000000000000000000, 0.000000000000000000, -0.000000000000000000 ) ) ;
#11521=CARTESIAN_POINT ( 'NONE',  ( 0.02407890056655651728, -3.506335382740735529, 30.89238256715863784 ) ) ;
#11524=CARTESIAN_POINT ( 'NONE',  ( 0.3923936511923831194, 30.27116788629744804, 13.00174666746672969 ) ) ;
#11540=VERTEX_POINT ( 'NONE', #3312 ) ;
#11547=CARTESIAN_POINT ( 'NONE',  ( 2.765921099433441555, 11.80989368511502846, -28.76039115933972923 ) ) ;
#11552=ORIENTED_EDGE ( 'NONE', *, *, #20176, .F. ) ;
#11563=CARTESIAN_POINT ( 'NONE',  ( 2.789999999999999147, -17.83604598421647935, -24.70480026434183429 ) ) ;
#11571=B_SPLINE_CURVE_WITH_KNOTS ( 'NONE', 3,
 ( #28621, #1395, #15454, #26291 ),
 .UNSPECIFIED., .F., .F.,
 ( 4, 4 ),
 ( 2.122664452422479579E-07, 0.0006879480821238842655 ),
 .UNSPECIFIED. ) ;
#11581=VECTOR ( 'NONE', #32222, 1000.000000000000000 ) ;
#11586=ORIENTED_EDGE ( 'NONE', *, *, #24252, .T. ) ;
#11593=FACE_OUTER_BOUND ( 'NONE', #1749, .T. ) ;
#11601=CARTESIAN_POINT ( 'NONE',  ( 2.789999999999999147, 0.000000000000000000, 0.000000000000000000 ) ) ;
#11602=DIRECTION ( 'NONE',  ( 0.000000000000000000, 0.000000000000000000, 1.000000000000000000 ) ) ;
#11609=CYLINDRICAL_SURFACE ( 'NONE', #4503, 16.19999999999999574 ) ;
#11611=CARTESIAN_POINT ( 'NONE',  ( 0.02407890056655608360, -31.05158812718222450, 1.559667679918499417 ) ) ;
#11620=CARTESIAN_POINT ( 'NONE',  ( 1.040000000000000924, 0.000000000000000000, 0.000000000000000000 ) ) ;
#11642=AXIS2_PLACEMENT_3D ( 'NONE', #20049, #34967, #2376 ) ;
#11652=DIRECTION ( 'NONE',  ( 0.000000000000000000, 0.000000000000000000, 1.000000000000000000 ) ) ;
#11656=FACE_OUTER_BOUND ( 'NONE', #26220, .T. ) ;
#11665=CARTESIAN_POINT ( 'NONE',  ( 0.000000000000000000, -23.41952779159748843, -19.49300927180572529 ) ) ;
#11668=CARTESIAN_POINT ( 'NONE',  ( 2.789999999999999147, 5.092684668492570843, 30.01061466292829394 ) ) ;
#11669=ORIENTED_EDGE ( 'NONE', *, *, #30169, .T. ) ;
#11673=CARTESIAN_POINT ( 'NONE',  ( 0.07094833952453778736, -3.385765165811753352, 31.51266256086713469 ) ) ;
#11678=AXIS2_PLACEMENT_3D ( 'NONE', #32332, #18829, #29672 ) ;
#11679=ADVANCED_FACE ( 'NONE', ( #15410 ), #33408, .T. ) ;
#11686=CARTESIAN_POINT ( 'NONE',  ( 2.789999999999999147, -3.728217946242703196, -30.24156218513559935 ) ) ;
#11687=CARTESIAN_POINT ( 'NONE',  ( 0.000000000000000000, -27.53147453683434520, 13.05640081644832939 ) ) ;
#11691=VERTEX_POINT ( 'NONE', #23409 ) ;
#11692=CARTESIAN_POINT ( 'NONE',  ( 1.039999999999999147, -33.39989884085096605, 8.296590337300141726 ) ) ;
#11695=CARTESIAN_POINT ( 'NONE',  ( 2.265105726929532270, -11.05013152551644851, 31.49770363594203104 ) ) ;
#11696=CYLINDRICAL_SURFACE ( 'NONE', #9719, 16.19999999999999574 ) ;
#11702=CARTESIAN_POINT ( 'NONE',  ( 2.789999999999999147, 28.52477022197315648, -10.62590764890695283 ) ) ;
#11715=EDGE_CURVE ( 'NONE', #21769, #15766, #12740, .T. ) ;
#11719=CARTESIAN_POINT ( 'NONE',  ( 1.749999999999999778, -18.21166265554766994, -29.20140402659760070 ) ) ;
#11723=CARTESIAN_POINT ( 'NONE',  ( 2.789999999999999147, -9.994970281559535152, 28.75192165143414869 ) ) ;
#11726=CARTESIAN_POINT ( 'NONE',  ( 1.749999999999999778, 6.183021911002332338, -33.85493898757056286 ) ) ;
#11728=CARTESIAN_POINT ( 'NONE',  ( 1.749999999999999778, -34.41385771548413430, 0.2702793785568976537 ) ) ;
#11738=DIRECTION ( 'NONE',  ( -1.000000000000000000, -0.000000000000000000, 0.000000000000000000 ) ) ;
#11752=CARTESIAN_POINT ( 'NONE',  ( 1.040000000000002922, -34.41385771548413430, 0.2702793785568980978 ) ) ;
#11753=B_SPLINE_CURVE_WITH_KNOTS ( 'NONE', 3,
 ( #12567, #34270, #30905, #20752 ),
 .UNSPECIFIED., .F., .F.,
 ( 4, 4 ),
 ( 1.992873153269112882E-07, 0.0006879349942371712880 ),
 .UNSPECIFIED. ) ;
#11758=CARTESIAN_POINT ( 'NONE',  ( 0.000000000000000000, -25.77598557799263901, 16.24962337825793313 ) ) ;
#11765=CARTESIAN_POINT ( 'NONE',  ( 2.765921099433442443, 30.61125888652961891, 5.439165181699118889 ) ) ;
#11768=ORIENTED_EDGE ( 'NONE', *, *, #13434, .T. ) ;
#11772=CIRCLE ( 'NONE', #31708, 34.41491905851385269 ) ;
#11773=EDGE_CURVE ( 'NONE', #27137, #33378, #18091, .T. ) ;
#11783=EDGE_CURVE ( 'NONE', #5077, #26849, #29457, .T. ) ;
#11790=CARTESIAN_POINT ( 'NONE',  ( 2.789999999999999147, 0.000000000000000000, 0.000000000000000000 ) ) ;
#11797=VERTEX_POINT ( 'NONE', #5051 ) ;
#11798=B_SPLINE_CURVE_WITH_KNOTS ( 'NONE', 3,
 ( #34021, #7475, #18198, #31523, #23514, #29022 ),
 .UNSPECIFIED., .F., .F.,
 ( 4, 2, 4 ),
 ( 2.343813143900254662E-07, 0.001873432713173583302, 0.003746631045032785060 ),
 .UNSPECIFIED. ) ;
#11819=VECTOR ( 'NONE', #26597, 1000.000000000000000 ) ;
#11823=ORIENTED_EDGE ( 'NONE', *, *, #34508, .F. ) ;
#11826=VECTOR ( 'NONE', #22363, 1000.000000000000000 ) ;
#11827=ADVANCED_FACE ( 'NONE', ( #21085 ), #29279, .F. ) ;
#11832=ORIENTED_EDGE ( 'NONE', *, *, #1100, .F. ) ;
#11853=CARTESIAN_POINT ( 'NONE',  ( 2.765921099433441555, 4.286445725888036407, 30.79383171238946204 ) ) ;
#11861=EDGE_LOOP ( 'NONE', ( #33079, #26442, #12615, #23525, #32896, #31533 ) ) ;
#11863=VERTEX_POINT ( 'NONE', #5404 ) ;
#11866=EDGE_CURVE ( 'NONE', #23276, #2234, #12970, .T. ) ;
#11867=AXIS2_PLACEMENT_3D ( 'NONE', #11790, #33654, #31334 ) ;
#11868=CARTESIAN_POINT ( 'NONE',  ( 2.789999999999999147, 19.87737664170521867, -23.05346671160885563 ) ) ;
#11873=ORIENTED_EDGE ( 'NONE', *, *, #34265, .F. ) ;
#11881=CARTESIAN_POINT ( 'NONE',  ( 2.789999999999999147, -20.35927063852789232, -22.08513060777193004 ) ) ;
#11884=DIRECTION ( 'NONE',  ( 0.000000000000000000, 0.000000000000000000, 1.000000000000000000 ) ) ;
#11893=AXIS2_PLACEMENT_3D ( 'NONE', #31249, #34090, #14898 ) ;
#11902=CARTESIAN_POINT ( 'NONE',  ( 1.040000000000000924, 0.000000000000000000, 0.000000000000000000 ) ) ;
#11903=ORIENTED_EDGE ( 'NONE', *, *, #2611, .F. ) ;
#11911=ORIENTED_EDGE ( 'NONE', *, *, #25136, .F. ) ;
#11913=EDGE_CURVE ( 'NONE', #13600, #8194, #22623, .T. ) ;
#11923=CARTESIAN_POINT ( 'NONE',  ( 2.790000000000000924, 1.224646799147353256E-15, -10.00000000000000000 ) ) ;
#11941=AXIS2_PLACEMENT_3D ( 'NONE', #10729, #8396, #21578 ) ;
#11945=ORIENTED_EDGE ( 'NONE', *, *, #6915, .T. ) ;
#11946=CARTESIAN_POINT ( 'NONE',  ( 2.765921099433441110, 11.80989368511462523, 28.76039115933989976 ) ) ;
#11950=B_SPLINE_CURVE_WITH_KNOTS ( 'NONE', 3,
 ( #11472, #33172, #8976, #3441, #22326, #612 ),
 .UNSPECIFIED., .F., .F.,
 ( 4, 2, 4 ),
 ( 2.011514595355519563E-07, 0.001873399447076926029, 0.003746597742694316585 ),
 .UNSPECIFIED. ) ;
#11956=CARTESIAN_POINT ( 'NONE',  ( 2.265105755614663874, -18.53613167721979949, 27.76008932203575696 ) ) ;
#11957=CARTESIAN_POINT ( 'NONE',  ( -5.210000000000000853, 0.000000000000000000, 0.000000000000000000 ) ) ;
#11960=EDGE_CURVE ( 'NONE', #6373, #18937, #1026, .T. ) ;
#11964=CARTESIAN_POINT ( 'NONE',  ( 2.033589655681871111, 33.57753319639237333, -4.776354065834818030 ) ) ;
#11969=ORIENTED_EDGE ( 'NONE', *, *, #13503, .F. ) ;
#11984=EDGE_CURVE ( 'NONE', #509, #34660, #27247, .T. ) ;
#11985=ORIENTED_EDGE ( 'NONE', *, *, #24378, .T. ) ;
#11993=ORIENTED_EDGE ( 'NONE', *, *, #30244, .F. ) ;
#11995=DIRECTION ( 'NONE',  ( 0.000000000000000000, 0.000000000000000000, 1.000000000000000000 ) ) ;
#12000=DIRECTION ( 'NONE',  ( 0.000000000000000000, 0.000000000000000000, 1.000000000000000000 ) ) ;
#12001=CARTESIAN_POINT ( 'NONE',  ( 0.7564103345238918363, -29.97226545381531082, 15.87222719455781750 ) ) ;
#12005=ORIENTED_EDGE ( 'NONE', *, *, #22191, .T. ) ;
#12009=CARTESIAN_POINT ( 'NONE',  ( 2.789999999999999147, 4.286445725888036407, 30.79383171238946204 ) ) ;
#12012=CARTESIAN_POINT ( 'NONE',  ( 0.008463494849040043358, -26.25524549613186309, -16.27432041257312179 ) ) ;
#12022=B_SPLINE_CURVE_WITH_KNOTS ( 'NONE', 3,
 ( #34401, #5702, #14099, #19272, #16782, #27610 ),
 .UNSPECIFIED., .F., .F.,
 ( 4, 2, 4 ),
 ( 4.404817168184892227E-07, 0.001874269729529006020, 0.003748098977341193273 ),
 .UNSPECIFIED. ) ;
#12024=CARTESIAN_POINT ( 'NONE',  ( 2.719010729300724627, 26.43944202223378426, -17.47857661787091743 ) ) ;
#12027=ADVANCED_FACE ( 'NONE', ( #14850 ), #26040, .T. ) ;
#12033=AXIS2_PLACEMENT_3D ( 'NONE', #12873, #1476, #21038 ) ;
#12042=DIRECTION ( 'NONE',  ( 0.000000000000000000, 0.000000000000000000, 1.000000000000000000 ) ) ;
#12043=AXIS2_PLACEMENT_3D ( 'NONE', #3754, #28495, #33655 ) ;
#12048=CARTESIAN_POINT ( 'NONE',  ( 0.7564103444830446721, 6.875279775961484319, -33.21136585175263178 ) ) ;
#12067=EDGE_CURVE ( 'NONE', #34039, #23769, #1481, .T. ) ;
#12073=CIRCLE ( 'NONE', #31925, 2.524999999999999467 ) ;
#12077=CIRCLE ( 'NONE', #31357, 34.41491905851385269 ) ;
#12081=EDGE_LOOP ( 'NONE', ( #26547, #25326, #14108, #25082, #10575, #27217, #20655, #1845 ) ) ;
#12084=CARTESIAN_POINT ( 'NONE',  ( 0.7561992243675458303, -29.46088656861464017, 16.80164552011240531 ) ) ;
#12097=CARTESIAN_POINT ( 'NONE',  ( 2.265105810640112072, -32.51534716424843907, 7.547378828040344878 ) ) ;
#12106=LINE ( 'NONE', #1582, #9809 ) ;
#12107=ORIENTED_EDGE ( 'NONE', *, *, #27407, .T. ) ;
#12111=CARTESIAN_POINT ( 'NONE',  ( 1.039999999999999369, -18.21166265554768060, -29.20140402659759360 ) ) ;
#12112=ADVANCED_FACE ( 'NONE', ( #3790 ), #34220, .T. ) ;
#12120=ORIENTED_EDGE ( 'NONE', *, *, #11218, .T. ) ;
#12125=EDGE_CURVE ( 'NONE', #14959, #16209, #31112, .T. ) ;
#12131=AXIS2_PLACEMENT_3D ( 'NONE', #29245, #26392, #15918 ) ;
#12136=DIRECTION ( 'NONE',  ( -1.000000000000000000, -0.000000000000000000, -0.000000000000000000 ) ) ;
#12139=ORIENTED_EDGE ( 'NONE', *, *, #26867, .T. ) ;
#12144=CIRCLE ( 'NONE', #6421, 34.41491905851385269 ) ;
#12152=APPLICATION_CONTEXT ( 'automotive_design' ) ;
#12159=EDGE_CURVE ( 'NONE', #33898, #11399, #19646, .T. ) ;
#12165=ORIENTED_EDGE ( 'NONE', *, *, #20382, .F. ) ;
#12167=DIRECTION ( 'NONE',  ( -1.000000000000000000, 0.000000000000000000, 0.000000000000000000 ) ) ;
#12170=EDGE_LOOP ( 'NONE', ( #19156, #8729, #9162, #5091, #14056, #1544 ) ) ;
#12190=EDGE_CURVE ( 'NONE', #527, #9865, #23716, .T. ) ;
#12194=LINE ( 'NONE', #25696, #14356 ) ;
#12198=CARTESIAN_POINT ( 'NONE',  ( 0.02407890056655825201, 14.63235270440936731, 27.43224275967444470 ) ) ;
#12208=EDGE_CURVE ( 'NONE', #23769, #13768, #8587, .T. ) ;
#12209=EDGE_CURVE ( 'NONE', #32759, #13324, #28337, .T. ) ;
#12214=ORIENTED_EDGE ( 'NONE', *, *, #5194, .F. ) ;
#12219=B_SPLINE_CURVE_WITH_KNOTS ( 'NONE', 3,
 ( #28225, #21034, #1519, #17397, #14718, #1348 ),
 .UNSPECIFIED., .F., .F.,
 ( 4, 2, 4 ),
 ( 4.404817002564675576E-07, 0.001874269606309967098, 0.003748098730919677702 ),
 .UNSPECIFIED. ) ;
#12223=DIRECTION ( 'NONE',  ( -1.000000000000000000, -0.000000000000000000, -0.000000000000000000 ) ) ;
#12226=TOROIDAL_SURFACE ( 'NONE', #8793, 30.47050528711512030, 8.000000000000000000 ) ;
#12227=CARTESIAN_POINT ( 'NONE',  ( 2.765921099433441999, -15.32140196853772984, 27.05343472112986092 ) ) ;
#12233=EDGE_CURVE ( 'NONE', #3012, #11540, #5564, .T. ) ;
#12237=ORIENTED_EDGE ( 'NONE', *, *, #30869, .F. ) ;
#12249=CIRCLE ( 'NONE', #32105, 30.47050528711511674 ) ;
#12250=ORIENTED_EDGE ( 'NONE', *, *, #11913, .T. ) ;
#12257=ORIENTED_EDGE ( 'NONE', *, *, #29248, .F. ) ;
#12262=CYLINDRICAL_SURFACE ( 'NONE', #11402, 34.41491905851385269 ) ;
#12267=B_SPLINE_CURVE_WITH_KNOTS ( 'NONE', 3,
 ( #3346, #19914, #14223, #25582 ),
 .UNSPECIFIED., .F., .F.,
 ( 4, 4 ),
 ( 0.005298404680630649545, 0.005985272568144306589 ),
 .UNSPECIFIED. ) ;
#12271=EDGE_CURVE ( 'NONE', #15134, #8335, #491, .T. ) ;
#12274=DIRECTION ( 'NONE',  ( 0.000000000000000000, 0.000000000000000000, 1.000000000000000000 ) ) ;
#12276=DIRECTION ( 'NONE',  ( -1.000000000000000000, -0.000000000000000000, -0.000000000000000000 ) ) ;
#12293=ORIENTED_EDGE ( 'NONE', *, *, #32968, .F. ) ;
#12297=VECTOR ( 'NONE', #26443, 1000.000000000000000 ) ;
#12301=ORIENTED_EDGE ( 'NONE', *, *, #34159, .T. ) ;
#12303=CARTESIAN_POINT ( 'NONE',  ( 2.789999999999999147, -5.984944020945660803, -31.37417528048448645 ) ) ;
#12314=DIRECTION ( 'NONE',  ( -1.000000000000000000, 0.000000000000000000, -0.000000000000000000 ) ) ;
#12317=B_SPLINE_CURVE_WITH_KNOTS ( 'NONE', 3,
 ( #32393, #31858, #21383, #2316, #29917, #16049 ),
 .UNSPECIFIED., .F., .F.,
 ( 4, 2, 4 ),
 ( 2.185847997378462515E-07, 0.001873416899431755780, 0.003746615214063773666 ),
 .UNSPECIFIED. ) ;
#12318=CARTESIAN_POINT ( 'NONE',  ( 2.765921099433441999, -23.70329957282570632, -20.11932597908854703 ) ) ;
#12320=AXIS2_PLACEMENT_3D ( 'NONE', #1333, #6656, #22874 ) ;
#12324=LINE ( 'NONE', #12494, #34971 ) ;
#12326=B_SPLINE_CURVE_WITH_KNOTS ( 'NONE', 3,
 ( #24151, #16168, #18834, #15992, #26829, #10987 ),
 .UNSPECIFIED., .F., .F.,
 ( 4, 2, 4 ),
 ( 2.434544809777742014E-07, 0.001873441796234163450, 0.003746640137987348844 ),
 .UNSPECIFIED. ) ;
#12328=CARTESIAN_POINT ( 'NONE',  ( 0.000000000000000000, -14.75935258146432005, 26.65732927035515232 ) ) ;
#12335=VERTEX_POINT ( 'NONE', #27435 ) ;
#12337=EDGE_LOOP ( 'NONE', ( #4632, #8523, #27391, #33417 ) ) ;
#12338=ORIENTED_EDGE ( 'NONE', *, *, #35018, .T. ) ;
#12340=CARTESIAN_POINT ( 'NONE',  ( -10.00000000000000000, 0.000000000000000000, 0.000000000000000000 ) ) ;
#12358=VECTOR ( 'NONE', #34698, 1000.000000000000000 ) ;
#12361=EDGE_CURVE ( 'NONE', #6345, #34702, #2732, .T. ) ;
#12369=CARTESIAN_POINT ( 'NONE',  ( 0.006892389992011671226, 14.58972988903167689, 27.20448975989783946 ) ) ;
#12370=DIRECTION ( 'NONE',  ( -1.000000000000000000, -0.000000000000000000, -0.000000000000000000 ) ) ;
#12371=FACE_OUTER_BOUND ( 'NONE', #4858, .T. ) ;
#12375=CARTESIAN_POINT ( 'NONE',  ( 1.749999999999999778, 27.68252950111338251, 20.44661865013498669 ) ) ;
#12381=AXIS2_PLACEMENT_3D ( 'NONE', #26126, #34854, #31635 ) ;
#12383=B_SPLINE_CURVE_WITH_KNOTS ( 'NONE', 3,
 ( #19977, #31344, #7123, #1106, #9638, #12668 ),
 .UNSPECIFIED., .F., .F.,
 ( 4, 2, 4 ),
 ( 1.991142096567175704E-07, 0.001873397407604852384, 0.003746595701000048073 ),
 .UNSPECIFIED. ) ;
#12389=AXIS2_PLACEMENT_3D ( 'NONE', #15286, #7239, #12606 ) ;
#12391=CARTESIAN_POINT ( 'NONE',  ( 2.789999999999999147, 3.909681563761668421, 30.21863799912384962 ) ) ;
#12402=CIRCLE ( 'NONE', #32268, 34.41491905851385269 ) ;
#12410=ORIENTED_EDGE ( 'NONE', *, *, #16611, .T. ) ;
#12411=AXIS2_PLACEMENT_3D ( 'NONE', #570, #24579, #401 ) ;
#12414=DIRECTION ( 'NONE',  ( 0.000000000000000000, 0.000000000000000000, 1.000000000000000000 ) ) ;
#12416=CARTESIAN_POINT ( 'NONE',  ( 2.789999999999999147, -3.506335382740311868, -30.89238256715869468 ) ) ;
#12420=VERTEX_POINT ( 'NONE', #13739 ) ;
#12431=ORIENTED_EDGE ( 'NONE', *, *, #20927, .T. ) ;
#12451=CARTESIAN_POINT ( 'NONE',  ( 0.02407890056655695096, -8.112136323389137260, 30.01377904834206589 ) ) ;
#12458=CARTESIAN_POINT ( 'NONE',  ( 2.789999999999999147, 14.59907093257217170, 26.74544485249471393 ) ) ;
#12460=CARTESIAN_POINT ( 'NONE',  ( -1.866546971192134421E-16, -26.00523011835690923, 16.24381534199252286 ) ) ;
#12466=EDGE_CURVE ( 'NONE', #32621, #3111, #5592, .T. ) ;
#12470=CARTESIAN_POINT ( 'NONE',  ( 0.1835380929791717852, -31.53621309121726313, -6.848028948310281194 ) ) ;
#12478=FACE_OUTER_BOUND ( 'NONE', #7437, .T. ) ;
#12483=CARTESIAN_POINT ( 'NONE',  ( 1.749999999999999778, 21.72796464722046039, -26.68861566460872226 ) ) ;
#12484=CYLINDRICAL_SURFACE ( 'NONE', #31899, 2.524999999999999467 ) ;
#12486=CIRCLE ( 'NONE', #28935, 34.41491905851385269 ) ;
#12494=CARTESIAN_POINT ( 'NONE',  ( 2.789999999999999147, 31.00221527374952046, -2.344426712874310148 ) ) ;
#12497=CARTESIAN_POINT ( 'NONE',  ( 0.000000000000000000, 7.489092610871091793, 29.53582882395389930 ) ) ;
#12503=ADVANCED_FACE ( 'NONE', ( #12614 ), #15639, .F. ) ;
#12504=ORIENTED_EDGE ( 'NONE', *, *, #32403, .F. ) ;
#12515=CARTESIAN_POINT ( 'NONE',  ( 1.040000000000001590, 27.68252950111337896, 20.44661865013498314 ) ) ;
#12523=VERTEX_POINT ( 'NONE', #4924 ) ;
#12525=CARTESIAN_POINT ( 'NONE',  ( 1.040000000000000480, 6.183021911001836735, 33.85493898757064812 ) ) ;
#12530=CIRCLE ( 'NONE', #1150, 34.41491905851385269 ) ;
#12533=DIRECTION ( 'NONE',  ( 0.000000000000000000, 0.000000000000000000, 1.000000000000000000 ) ) ;
#12535=CARTESIAN_POINT ( 'NONE',  ( 2.765921099433441555, 24.20451283648857554, -19.51346322004903300 ) ) ;
#12538=DIRECTION ( 'NONE',  ( -1.000000000000000000, -0.000000000000000000, -0.000000000000000000 ) ) ;
#12540=EDGE_CURVE ( 'NONE', #32759, #10218, #21341, .T. ) ;
#12547=B_SPLINE_CURVE_WITH_KNOTS ( 'NONE', 3,
 ( #15754, #10219, #31914, #7530 ),
 .UNSPECIFIED., .F., .F.,
 ( 4, 4 ),
 ( 1.976296719774608551E-07, 0.0006879333227023559953 ),
 .UNSPECIFIED. ) ;
#12549=DIRECTION ( 'NONE',  ( 0.000000000000000000, 0.7705132427757948044, -0.6374239897486828621 ) ) ;
#12558=ORIENTED_EDGE ( 'NONE', *, *, #32968, .T. ) ;
#12560=DIRECTION ( 'NONE',  ( -1.000000000000000000, 0.000000000000000000, -0.000000000000000000 ) ) ;
#12567=CARTESIAN_POINT ( 'NONE',  ( 2.765921099433442443, 30.61125888652969707, -5.439165181698684570 ) ) ;
#12568=VECTOR ( 'NONE', #34402, 1000.000000000000000 ) ;
#12569=DIRECTION ( 'NONE',  ( 0.000000000000000000, 0.000000000000000000, 1.000000000000000000 ) ) ;
#12570=EDGE_LOOP ( 'NONE', ( #24083, #11768, #6987, #23211, #25515, #24606, #22569, #3079 ) ) ;
#12572=MECHANICAL_DESIGN_GEOMETRIC_PRESENTATION_REPRESENTATION('',(#9941),#622);
#12573=CARTESIAN_POINT ( 'NONE',  ( 0.07094834019209503295, 31.23788557484574113, 5.357780584451035999 ) ) ;
#12578=ORIENTED_EDGE ( 'NONE', *, *, #1686, .F. ) ;
#12579=AXIS2_PLACEMENT_3D ( 'NONE', #10939, #21786, #32634 ) ;
#12604=ORIENTED_EDGE ( 'NONE', *, *, #34862, .F. ) ;
#12605=ORIENTED_EDGE ( 'NONE', *, *, #13434, .F. ) ;
#12606=DIRECTION ( 'NONE',  ( 0.000000000000000000, 0.000000000000000000, 1.000000000000000000 ) ) ;
#12614=FACE_OUTER_BOUND ( 'NONE', #22713, .T. ) ;
#12615=ORIENTED_EDGE ( 'NONE', *, *, #20251, .F. ) ;
#12626=AXIS2_PLACEMENT_3D ( 'NONE', #2610, #10639, #17176 ) ;
#12648=ORIENTED_EDGE ( 'NONE', *, *, #20513, .F. ) ;
#12649=CARTESIAN_POINT ( 'NONE',  ( 1.394999999999999574, -30.28730148581150416, -16.34215476954067015 ) ) ;
#12663=ORIENTED_EDGE ( 'NONE', *, *, #22437, .F. ) ;
#12664=FACE_BOUND ( 'NONE', #9225, .T. ) ;
#12668=CARTESIAN_POINT ( 'NONE',  ( 1.749999999999999778, 34.10861917999616111, 4.581348211832198203 ) ) ;
#12669=CARTESIAN_POINT ( 'NONE',  ( 2.765921099433441999, -31.05158812718222450, 1.559667679918499417 ) ) ;
#12673=VECTOR ( 'NONE', #14157, 1000.000000000000000 ) ;
#12693=LINE ( 'NONE', #29407, #26630 ) ;
#12694=AXIS2_PLACEMENT_3D ( 'NONE', #1371, #3844, #12414 ) ;
#12702=EDGE_CURVE ( 'NONE', #32635, #32497, #25935, .T. ) ;
#12703=CARTESIAN_POINT ( 'NONE',  ( 0.07098928180586180914, 29.95554370010543366, 10.35423322779187316 ) ) ;
#12704=CARTESIAN_POINT ( 'NONE',  ( 0.000000000000000000, 27.60935207499572996, -12.89090262359622585 ) ) ;
#12710=EDGE_CURVE ( 'NONE', #797, #34043, #33218, .T. ) ;
#12713=CARTESIAN_POINT ( 'NONE',  ( 8.000000000000000000, 0.000000000000000000, 0.000000000000000000 ) ) ;
#12715=DIRECTION ( 'NONE',  ( 0.000000000000000000, 0.000000000000000000, 1.000000000000000000 ) ) ;
#12729=DIRECTION ( 'NONE',  ( 0.000000000000000000, 0.000000000000000000, 1.000000000000000000 ) ) ;
#12734=CARTESIAN_POINT ( 'NONE',  ( 2.789999999999999147, -27.53147453683434520, 13.05640081644830097 ) ) ;
#12740=LINE ( 'NONE', #4351, #2155 ) ;
#12741=B_SPLINE_CURVE_WITH_KNOTS ( 'NONE', 3,
 ( #9470, #3764, #6603, #1277, #9289, #30655 ),
 .UNSPECIFIED., .F., .F.,
 ( 4, 2, 4 ),
 ( 2.126639591840487065E-07, 0.001873410972133594376, 0.003746609280308004809 ),
 .UNSPECIFIED. ) ;
#12749=CARTESIAN_POINT ( 'NONE',  ( 1.749999999999999778, 34.10861917999616111, 4.581348211832198203 ) ) ;
#12750=ADVANCED_FACE ( 'NONE', ( #30729 ), #17051, .T. ) ;
#12757=DIRECTION ( 'NONE',  ( -1.000000000000000000, -0.000000000000000000, -0.000000000000000000 ) ) ;
#12776=ORIENTED_EDGE ( 'NONE', *, *, #12209, .F. ) ;
#12780=AXIS2_PLACEMENT_3D ( 'NONE', #23393, #15228, #26067 ) ;
#12785=VERTEX_POINT ( 'NONE', #8655 ) ;
#12791=CIRCLE ( 'NONE', #23600, 10.00000000000000000 ) ;
#12793=CARTESIAN_POINT ( 'NONE',  ( 1.749999999999999778, 6.183021911002332338, -33.85493898757056286 ) ) ;
#12797=EDGE_CURVE ( 'NONE', #33874, #7570, #22193, .T. ) ;
#12809=DIRECTION ( 'NONE',  ( 0.000000000000000000, 0.000000000000000000, 1.000000000000000000 ) ) ;
#12815=EDGE_LOOP ( 'NONE', ( #21504, #27109, #16380, #16175, #7688, #28355, #19688, #13744 ) ) ;
#12821=VERTEX_POINT ( 'NONE', #33396 ) ;
#12823=CARTESIAN_POINT ( 'NONE',  ( 0.07098930119792198901, -31.01706505092331057, -6.518161977769946880 ) ) ;
#12834=CARTESIAN_POINT ( 'NONE',  ( 2.033800780387780449, 22.02446183774672761, -25.79073883748058549 ) ) ;
#12837=DIRECTION ( 'NONE',  ( -1.000000000000000000, -0.000000000000000000, -0.000000000000000000 ) ) ;
#12850=CARTESIAN_POINT ( 'NONE',  ( 0.000000000000000000, 29.94779062842797401, -5.619744560738746841 ) ) ;
#12852=DIRECTION ( 'NONE',  ( -1.000000000000000000, 0.000000000000000000, -0.000000000000000000 ) ) ;
#12856=ORIENTED_EDGE ( 'NONE', *, *, #32657, .T. ) ;
#12857=EDGE_CURVE ( 'NONE', #25712, #4047, #5109, .T. ) ;
#12858=ORIENTED_EDGE ( 'NONE', *, *, #16494, .F. ) ;
#12860=ADVANCED_FACE ( 'NONE', ( #9708 ), #15900, .T. ) ;
#12867=CARTESIAN_POINT ( 'NONE',  ( 1.749999999999999778, 27.68252950111368094, -20.44661865013457458 ) ) ;
#12873=CARTESIAN_POINT ( 'NONE',  ( 2.789999999999999147, 0.000000000000000000, 0.000000000000000000 ) ) ;
#12874=EDGE_LOOP ( 'NONE', ( #992, #289, #9171, #2590 ) ) ;
#12878=CARTESIAN_POINT ( 'NONE',  ( -8.214752480152773925E-14, 25.77088461037005729, -16.61521147790355002 ) ) ;
#12879=B_SPLINE_CURVE_WITH_KNOTS ( 'NONE', 3,
 ( #26097, #4712, #23096, #17759 ),
 .UNSPECIFIED., .F., .F.,
 ( 4, 4 ),
 ( 2.122664452422532254E-07, 0.0006879480821238661593 ),
 .UNSPECIFIED. ) ;
#12884=EDGE_LOOP ( 'NONE', ( #28990, #30063, #12604, #32934 ) ) ;
#12892=CARTESIAN_POINT ( 'NONE',  ( 1.749999999999999778, 21.72796464722008380, 26.68861566460903489 ) ) ;
#12895=B_SPLINE_CURVE_WITH_KNOTS ( 'NONE', 3,
 ( #20377, #31225, #20207, #23219, #3975, #9680 ),
 .UNSPECIFIED., .F., .F.,
 ( 4, 2, 4 ),
 ( 4.404817030623842623E-07, 0.001874269627226452005, 0.003748098772749841601 ),
 .UNSPECIFIED. ) ;
#12921=CARTESIAN_POINT ( 'NONE',  ( 2.789999999999999147, 23.28319895603578971, 21.86437915510226659 ) ) ;
#12923=LINE ( 'NONE', #4518, #4566 ) ;
#12927=EDGE_LOOP ( 'NONE', ( #33102, #4335, #3099, #14793 ) ) ;
#12930=CARTESIAN_POINT ( 'NONE',  ( 2.790000000000082636, -7.838364976555836527, 29.64395146466208431 ) ) ;
#12933=CARTESIAN_POINT ( 'NONE',  ( 2.789999999999999147, 12.39602498911143869, 27.80127684205872285 ) ) ;
#12943=CARTESIAN_POINT ( 'NONE',  ( 2.261199760199078757, 27.45925096103250240, 18.99654502929957900 ) ) ;
#12944=EDGE_CURVE ( 'NONE', #34260, #12785, #11054, .T. ) ;
#12946=VECTOR ( 'NONE', #3830, 1000.000000000000000 ) ;
#12947=ADVANCED_FACE ( 'NONE', ( #31938 ), #27231, .T. ) ;
#12957=CARTESIAN_POINT ( 'NONE',  ( 2.789999999999999147, -26.96806452364372575, -14.11722088188941804 ) ) ;
#12962=DIRECTION ( 'NONE',  ( 0.000000000000000000, 0.000000000000000000, -1.000000000000000000 ) ) ;
#12964=FACE_OUTER_BOUND ( 'NONE', #6130, .T. ) ;
#12969=DIRECTION ( 'NONE',  ( -1.000000000000000000, -0.000000000000000000, -0.000000000000000000 ) ) ;
#12970=CIRCLE ( 'NONE', #16386, 30.47050528711511674 ) ;
#12978=EDGE_LOOP ( 'NONE', ( #16606, #34035, #21068, #2241 ) ) ;
#12989=ADVANCED_FACE ( 'NONE', ( #33929 ), #32640, .F. ) ;
#12990=ORIENTED_EDGE ( 'NONE', *, *, #27186, .T. ) ;
#12992=B_SPLINE_CURVE_WITH_KNOTS ( 'NONE', 3,
 ( #19827, #589, #20818, #20646 ),
 .UNSPECIFIED., .F., .F.,
 ( 4, 4 ),
 ( 0.005298517298376331439, 0.005985383706685557664 ),
 .UNSPECIFIED. ) ;
#12997=EDGE_CURVE ( 'NONE', #23325, #2234, #30085, .T. ) ;
#12999=ORIENTED_EDGE ( 'NONE', *, *, #1833, .T. ) ;
#13013=ORIENTED_EDGE ( 'NONE', *, *, #1959, .T. ) ;
#13017=B_SPLINE_CURVE_WITH_KNOTS ( 'NONE', 3,
 ( #30768, #3877, #1052, #12097, #23293, #19754 ),
 .UNSPECIFIED., .F., .F.,
 ( 4, 2, 4 ),
 ( 2.257612537733862618E-07, 0.001873424083712457808, 0.003746622406171142526 ),
 .UNSPECIFIED. ) ;
#13018=CARTESIAN_POINT ( 'NONE',  ( -5.210000000000000853, 0.000000000000000000, 0.000000000000000000 ) ) ;
#13021=CARTESIAN_POINT ( 'NONE',  ( 2.789999999999999147, 11.30192140231272191, -28.29696565125058072 ) ) ;
#13028=CARTESIAN_POINT ( 'NONE',  ( 2.790000000000080860, 18.20059223136379600, -24.67675383855231885 ) ) ;
#13036=CARTESIAN_POINT ( 'NONE',  ( 0.000000000000000000, 0.000000000000000000, 0.000000000000000000 ) ) ;
#13039=VERTEX_POINT ( 'NONE', #2915 ) ;
#13043=DIRECTION ( 'NONE',  ( 0.000000000000000000, 0.000000000000000000, 1.000000000000000000 ) ) ;
#13050=CARTESIAN_POINT ( 'NONE',  ( 2.789999999999999147, -27.53147453683434520, 13.05640081644830097 ) ) ;
#13057=DIRECTION ( 'NONE',  ( 0.000000000000000000, 0.000000000000000000, 1.000000000000000000 ) ) ;
#13064=EDGE_CURVE ( 'NONE', #9815, #32472, #12486, .T. ) ;
#13065=CARTESIAN_POINT ( 'NONE',  ( 1.394999999999999574, 14.40815186467776243, 31.25366880301324457 ) ) ;
#13073=DIRECTION ( 'NONE',  ( 1.000000000000000000, 0.000000000000000000, 0.000000000000000000 ) ) ;
#13078=VERTEX_POINT ( 'NONE', #5579 ) ;
#13080=ORIENTED_EDGE ( 'NONE', *, *, #25550, .F. ) ;
#13084=CARTESIAN_POINT ( 'NONE',  ( 2.789999999999999591, 0.000000000000000000, 3.000000000000000000 ) ) ;
#13106=EDGE_LOOP ( 'NONE', ( #7308, #1215, #32524, #25166 ) ) ;
#13107=CARTESIAN_POINT ( 'NONE',  ( 0.07406964051085589140, 28.96583153378254849, 12.96313068902594878 ) ) ;
#13110=EDGE_CURVE ( 'NONE', #6878, #22746, #11950, .T. ) ;
#13129=EDGE_LOOP ( 'NONE', ( #7506, #21027, #8446, #8378 ) ) ;
#13138=ORIENTED_EDGE ( 'NONE', *, *, #2196, .T. ) ;
#13146=VERTEX_POINT ( 'NONE', #33355 ) ;
#13156=DIRECTION ( 'NONE',  ( 0.000000000000000000, 0.000000000000000000, 1.000000000000000000 ) ) ;
#13159=VERTEX_POINT ( 'NONE', #19847 ) ;
#13160=EDGE_LOOP ( 'NONE', ( #16926, #18776, #20340, #13686, #18608, #5113 ) ) ;
#13178=EDGE_CURVE ( 'NONE', #33934, #20222, #25336, .T. ) ;
#13186=DIRECTION ( 'NONE',  ( 0.000000000000000000, 0.000000000000000000, 1.000000000000000000 ) ) ;
#13193=AXIS2_PLACEMENT_3D ( 'NONE', #831, #9017, #20407 ) ;
#13194=CARTESIAN_POINT ( 'NONE',  ( -10.00000000000000000, 0.000000000000000000, 0.000000000000000000 ) ) ;
#13196=CARTESIAN_POINT ( 'NONE',  ( 2.789999999999999147, -31.68806325674604452, -4.003133335385915537 ) ) ;
#13198=DIRECTION ( 'NONE',  ( 0.000000000000000000, 0.000000000000000000, 1.000000000000000000 ) ) ;
#13213=ORIENTED_EDGE ( 'NONE', *, *, #18459, .T. ) ;
#13227=DIRECTION ( 'NONE',  ( -1.000000000000000000, -0.000000000000000000, -0.000000000000000000 ) ) ;
#13229=DIRECTION ( 'NONE',  ( -1.000000000000000000, 0.000000000000000000, 0.000000000000000000 ) ) ;
#13238=CARTESIAN_POINT ( 'NONE',  ( 0.02407890056655695096, 30.61125888652961891, 5.439165181699118889 ) ) ;
#13241=CARTESIAN_POINT ( 'NONE',  ( 2.719051664055850637, 24.79283726477138217, -19.74402504231769129 ) ) ;
#13246=CARTESIAN_POINT ( 'NONE',  ( 2.789999999999999147, 9.869977788041397915, -30.37666815053925973 ) ) ;
#13252=AXIS2_PLACEMENT_3D ( 'NONE', #27269, #30118, #5374 ) ;
#13256=VERTEX_POINT ( 'NONE', #1490 ) ;
#13257=CARTESIAN_POINT ( 'NONE',  ( 1.749999999999999778, 0.000000000000000000, 0.000000000000000000 ) ) ;
#13260=ADVANCED_FACE ( 'NONE', ( #23036 ), #4486, .T. ) ;
#13262=EDGE_LOOP ( 'NONE', ( #21144, #206, #19035, #32374, #11903, #8173 ) ) ;
#13279=ORIENTED_EDGE ( 'NONE', *, *, #26224, .F. ) ;
#13286=CARTESIAN_POINT ( 'NONE',  ( 0.006892432010618929766, -3.550547054313539341, -30.66493323461388698 ) ) ;
#13292=ORIENTED_EDGE ( 'NONE', *, *, #33893, .F. ) ;
#13294=CIRCLE ( 'NONE', #20678, 2.525000000000000355 ) ;
#13315=CARTESIAN_POINT ( 'NONE',  ( 0.02407890056655651728, -3.506335382740735529, 30.89238256715863784 ) ) ;
#13316=CARTESIAN_POINT ( 'NONE',  ( 1.395000000000002238, 32.09669216789236401, 12.41728656686386500 ) ) ;
#13323=CARTESIAN_POINT ( 'NONE',  ( 1.749999999999999778, 31.89769921723006263, -12.91988538846924151 ) ) ;
#13324=VERTEX_POINT ( 'NONE', #9325 ) ;
#13327=ORIENTED_EDGE ( 'NONE', *, *, #30783, .F. ) ;
#13334=DIRECTION ( 'NONE',  ( -1.000000000000000000, -0.000000000000000000, -0.000000000000000000 ) ) ;
#13335=CARTESIAN_POINT ( 'NONE',  ( -5.210000000000000853, 0.000000000000000000, 0.000000000000000000 ) ) ;
#13347=ADVANCED_FACE ( 'NONE', ( #3340 ), #1033, .T. ) ;
#13353=CYLINDRICAL_SURFACE ( 'NONE', #20337, 2.524999999999999467 ) ;
#13357=EDGE_LOOP ( 'NONE', ( #15065, #32264, #326, #35078 ) ) ;
#13358=ORIENTED_EDGE ( 'NONE', *, *, #24493, .F. ) ;
#13363=DIRECTION ( 'NONE',  ( 1.000000000000000000, 0.000000000000000000, 0.000000000000000000 ) ) ;
#13370=CYLINDRICAL_SURFACE ( 'NONE', #7006, 34.41491905851385269 ) ;
#13379=AXIS2_PLACEMENT_3D ( 'NONE', #31147, #3199, #28117 ) ;
#13386=DIRECTION ( 'NONE',  ( 0.000000000000000000, 0.000000000000000000, 1.000000000000000000 ) ) ;
#13400=CARTESIAN_POINT ( 'NONE',  ( 0.000000000000000000, 2.005524111408653720, -31.87689292423236154 ) ) ;
#13401=CARTESIAN_POINT ( 'NONE',  ( 0.5248942638477641642, 14.91070698422159779, 29.86438609618750561 ) ) ;
#13406=CARTESIAN_POINT ( 'NONE',  ( 2.789999999999999147, -17.95514392185434360, 25.38201125280350468 ) ) ;
#13413=DIRECTION ( 'NONE',  ( -1.000000000000000000, -0.000000000000000000, -0.000000000000000000 ) ) ;
#13416=CARTESIAN_POINT ( 'NONE',  ( 8.000000000000000000, 0.000000000000000000, 0.000000000000000000 ) ) ;
#13419=EDGE_LOOP ( 'NONE', ( #23438, #17052, #26256, #3301 ) ) ;
#13428=EDGE_CURVE ( 'NONE', #23263, #1567, #25483, .T. ) ;
#13432=CARTESIAN_POINT ( 'NONE',  ( 50.00050000000000239, 0.000000000000000000, 0.000000000000000000 ) ) ;
#13433=ORIENTED_EDGE ( 'NONE', *, *, #26467, .T. ) ;
#13434=EDGE_CURVE ( 'NONE', #10218, #5629, #25403, .T. ) ;
#13444=DIRECTION ( 'NONE',  ( 0.000000000000000000, 4.122115190439938353E-15, -1.000000000000000000 ) ) ;
#13445=VERTEX_POINT ( 'NONE', #20262 ) ;
#13448=CARTESIAN_POINT ( 'NONE',  ( 2.606461794449805858, -30.93445778156022641, -9.191712967691181291 ) ) ;
#13449=ORIENTED_EDGE ( 'NONE', *, *, #15855, .T. ) ;
#13451=VERTEX_POINT ( 'NONE', #19730 ) ;
#13463=FACE_OUTER_BOUND ( 'NONE', #27191, .T. ) ;
#13471=EDGE_CURVE ( 'NONE', #20282, #12420, #17634, .T. ) ;
#13473=ADVANCED_FACE ( 'NONE', ( #22750 ), #31111, .T. ) ;
#13492=CARTESIAN_POINT ( 'NONE',  ( 0.000000000000000000, 30.40449935640659973, -2.004522720844279959 ) ) ;
#13503=EDGE_CURVE ( 'NONE', #33936, #509, #9353, .T. ) ;
#13508=CARTESIAN_POINT ( 'NONE',  ( 1.040000000000002922, -34.41385771548413430, 0.2702793785568980978 ) ) ;
#13511=DIRECTION ( 'NONE',  ( -1.000000000000000000, -0.000000000000000000, -0.000000000000000000 ) ) ;
#13514=CARTESIAN_POINT ( 'NONE',  ( 0.0001801434340936737804, -25.83993731729792742, -16.24881338200996694 ) ) ;
#13525=ORIENTED_EDGE ( 'NONE', *, *, #9542, .F. ) ;
#13548=CARTESIAN_POINT ( 'NONE',  ( 2.789999999999999147, 24.98605633783575897, 17.38589710834512658 ) ) ;
#13550=ORIENTED_EDGE ( 'NONE', *, *, #24252, .F. ) ;
#13551=CARTESIAN_POINT ( 'NONE',  ( 0.000000000000000000, -11.13185981125894486, 28.36429779836949194 ) ) ;
#13558=CARTESIAN_POINT ( 'NONE',  ( 1.749999999999999778, 0.000000000000000000, 0.000000000000000000 ) ) ;
#13560=ORIENTED_EDGE ( 'NONE', *, *, #4669, .T. ) ;
#13561=FACE_OUTER_BOUND ( 'NONE', #12570, .T. ) ;
#13564=VECTOR ( 'NONE', #18525, 1000.000000000000000 ) ;
#13567=EDGE_LOOP ( 'NONE', ( #8524, #21708, #31458, #34872, #6024, #28151 ) ) ;
#13573=CARTESIAN_POINT ( 'NONE',  ( -10.00000000000000000, 0.000000000000000000, 0.000000000000000000 ) ) ;
#13574=EDGE_LOOP ( 'NONE', ( #29565, #8088, #15285, #537 ) ) ;
#13581=CARTESIAN_POINT ( 'NONE',  ( 0.1835382038249109005, 7.231184547465314694, 31.45056812073516994 ) ) ;
#13590=DIRECTION ( 'NONE',  ( -1.000000000000000000, -0.000000000000000000, -0.000000000000000000 ) ) ;
#13593=CARTESIAN_POINT ( 'NONE',  ( 2.783107618865146016, -23.57982834652860049, 19.92325699910536940 ) ) ;
#13600=VERTEX_POINT ( 'NONE', #107 ) ;
#13604=CARTESIAN_POINT ( 'NONE',  ( 2.790000000000082192, -27.65011189337340625, -13.25424764731434557 ) ) ;
#13610=CARTESIAN_POINT ( 'NONE',  ( 2.783128948453668983, 7.365904273040312589, 29.97784191786588082 ) ) ;
#13619=DIRECTION ( 'NONE',  ( 1.000000000000000000, -0.000000000000000000, 0.000000000000000000 ) ) ;
#13622=ORIENTED_EDGE ( 'NONE', *, *, #6086, .T. ) ;
#13633=ADVANCED_FACE ( 'NONE', ( #33862 ), #6966, .T. ) ;
#13651=CARTESIAN_POINT ( 'NONE',  ( 50.00050000000000239, 0.000000000000000000, 10.00000000000000000 ) ) ;
#13656=DIRECTION ( 'NONE',  ( -1.000000000000000000, 0.000000000000000000, 0.000000000000000000 ) ) ;
#13658=ORIENTED_EDGE ( 'NONE', *, *, #17443, .T. ) ;
#13661=EDGE_CURVE ( 'NONE', #4938, #29908, #13995, .T. ) ;
#13669=CARTESIAN_POINT ( 'NONE',  ( 1.394999999999999574, 14.89726405156260292, -31.02351007835962093 ) ) ;
#13670=DIRECTION ( 'NONE',  ( 0.000000000000000000, 0.000000000000000000, 1.000000000000000000 ) ) ;
#13676=CARTESIAN_POINT ( 'NONE',  ( 0.000000000000000000, -7.666252171205713672, 29.49034198003804974 ) ) ;
#13678=B_SPLINE_CURVE_WITH_KNOTS ( 'NONE', 3,
 ( #13713, #8369, #11227, #22078, #32919, #8540 ),
 .UNSPECIFIED., .F., .F.,
 ( 4, 2, 4 ),
 ( 4.404817011858791706E-07, 0.001874269613276467825, 0.003748098744851749778 ),
 .UNSPECIFIED. ) ;
#13681=CARTESIAN_POINT ( 'NONE',  ( 2.789999999999999147, 11.80989368511462523, 28.76039115933989976 ) ) ;
#13682=CARTESIAN_POINT ( 'NONE',  ( 1.749999999999999778, 14.89726405156260469, -31.02351007835961383 ) ) ;
#13686=ORIENTED_EDGE ( 'NONE', *, *, #30619, .F. ) ;
#13689=LINE ( 'NONE', #24884, #34188 ) ;
#13694=VERTEX_POINT ( 'NONE', #15180 ) ;
#13698=CARTESIAN_POINT ( 'NONE',  ( 2.765921099433443331, 18.59128259035506758, -24.91982945642901726 ) ) ;
#13706=ORIENTED_EDGE ( 'NONE', *, *, #1640, .F. ) ;
#13709=CARTESIAN_POINT ( 'NONE',  ( 2.261199742870364293, -28.88016830755709563, 16.75753762755134701 ) ) ;
#13711=EDGE_CURVE ( 'NONE', #8526, #23276, #29266, .T. ) ;
#13713=CARTESIAN_POINT ( 'NONE',  ( 1.749999999999999778, -2.430610048905780030, -34.32897884578301984 ) ) ;
#13731=ADVANCED_FACE ( 'NONE', ( #1293 ), #28691, .T. ) ;
#13738=FACE_OUTER_BOUND ( 'NONE', #25317, .T. ) ;
#13739=CARTESIAN_POINT ( 'NONE',  ( 1.040000000000001368, -30.28730148581149706, -16.34215476954066304 ) ) ;
#13740=EDGE_CURVE ( 'NONE', #34596, #292, #25669, .T. ) ;
#13742=CARTESIAN_POINT ( 'NONE',  ( 2.765921099433441110, -27.96208973699912548, 13.59246946040177129 ) ) ;
#13744=ORIENTED_EDGE ( 'NONE', *, *, #4129, .F. ) ;
#13748=CARTESIAN_POINT ( 'NONE',  ( 2.033589665237263144, -17.72288109958232383, 28.91649664306117629 ) ) ;
#13752=B_SPLINE_CURVE_WITH_KNOTS ( 'NONE', 3,
 ( #31008, #938, #8457, #9112, #13803, #30833 ),
 .UNSPECIFIED., .F., .F.,
 ( 4, 2, 4 ),
 ( 2.248981763129687575E-07, 0.001873423219693742293, 0.003746621541211171691 ),
 .UNSPECIFIED. ) ;
#13761=CARTESIAN_POINT ( 'NONE',  ( 1.040000000000000702, -10.37741591188916779, 32.81304455236864470 ) ) ;
#13763=ORIENTED_EDGE ( 'NONE', *, *, #23923, .F. ) ;
#13768=VERTEX_POINT ( 'NONE', #4818 ) ;
#13776=EDGE_CURVE ( 'NONE', #32621, #25011, #17093, .T. ) ;
#13779=EDGE_CURVE ( 'NONE', #16592, #30042, #15949, .T. ) ;
#13798=ORIENTED_EDGE ( 'NONE', *, *, #14644, .T. ) ;
#13803=CARTESIAN_POINT ( 'NONE',  ( 0.7561992172567417736, -24.35691930005274131, 23.60041548268705114 ) ) ;
#13808=CARTESIAN_POINT ( 'NONE',  ( 1.040000000000000924, 0.000000000000000000, 0.000000000000000000 ) ) ;
#13810=ORIENTED_EDGE ( 'NONE', *, *, #6815, .F. ) ;
#13812=VERTEX_POINT ( 'NONE', #15710 ) ;
#13820=EDGE_CURVE ( 'NONE', #22622, #8018, #4542, .T. ) ;
#13832=CARTESIAN_POINT ( 'NONE',  ( 8.000000000000000000, 0.000000000000000000, 0.000000000000000000 ) ) ;
#13839=LINE ( 'NONE', #312, #17181 ) ;
#13840=FACE_OUTER_BOUND ( 'NONE', #2117, .T. ) ;
#13846=CIRCLE ( 'NONE', #16708, 34.41491905851385269 ) ;
#13853=ORIENTED_EDGE ( 'NONE', *, *, #3591, .F. ) ;
#13857=DIRECTION ( 'NONE',  ( 0.000000000000000000, 0.000000000000000000, 1.000000000000000000 ) ) ;
#13858=EDGE_LOOP ( 'NONE', ( #3121, #11337, #33960, #29738 ) ) ;
#13866=VERTEX_POINT ( 'NONE', #29032 ) ;
#13867=EDGE_CURVE ( 'NONE', #29138, #5785, #18787, .T. ) ;
#13870=CARTESIAN_POINT ( 'NONE',  ( 2.783107618352422374, 18.40335333576878440, 24.78429060331947298 ) ) ;
#13872=CARTESIAN_POINT ( 'NONE',  ( 1.749999999999999778, -24.90160365674886478, 23.75493189058330756 ) ) ;
#13876=ADVANCED_FACE ( 'NONE', ( #4633 ), #2274, .T. ) ;
#13877=DIRECTION ( 'NONE',  ( -1.000000000000000000, -0.000000000000000000, -0.000000000000000000 ) ) ;
#13889=DIRECTION ( 'NONE',  ( -1.000000000000000000, 0.000000000000000000, -0.000000000000000000 ) ) ;
#13908=ORIENTED_EDGE ( 'NONE', *, *, #5114, .T. ) ;
#13909=CARTESIAN_POINT ( 'NONE',  ( 2.789999999999999147, -25.83993731729781729, -18.77381338200996552 ) ) ;
#13913=CARTESIAN_POINT ( 'NONE',  ( 2.719051662517718793, -18.14830959286877388, -25.98365187356541028 ) ) ;
#13922=DIRECTION ( 'NONE',  ( 0.000000000000000000, 0.5877852522924797984, -0.8090169943749424553 ) ) ;
#13926=VECTOR ( 'NONE', #16282, 1000.000000000000000 ) ;
#13928=B_SPLINE_CURVE_WITH_KNOTS ( 'NONE', 3,
 ( #28988, #9609, #31482, #15481 ),
 .UNSPECIFIED., .F., .F.,
 ( 4, 4 ),
 ( 2.080333525986984783E-07, 0.0006879438135628625824 ),
 .UNSPECIFIED. ) ;
#13930=CYLINDRICAL_SURFACE ( 'NONE', #31127, 16.19999999999999574 ) ;
#13946=ADVANCED_FACE ( 'NONE', ( #30097 ), #27422, .T. ) ;
#13952=B_SPLINE_CURVE_WITH_KNOTS ( 'NONE', 3,
 ( #27220, #32210, #10688, #7823 ),
 .UNSPECIFIED., .F., .F.,
 ( 4, 4 ),
 ( 2.013258991796058355E-07, 0.0006879370499044200164 ),
 .UNSPECIFIED. ) ;
#13957=EDGE_LOOP ( 'NONE', ( #31535, #7893, #3902, #2695 ) ) ;
#13961=DIRECTION ( 'NONE',  ( -1.000000000000000000, -0.000000000000000000, -0.000000000000000000 ) ) ;
#13979=CARTESIAN_POINT ( 'NONE',  ( 2.719010670248903416, 7.308614668456580254, -30.84037831947987485 ) ) ;
#13987=EDGE_CURVE ( 'NONE', #34921, #6854, #26716, .T. ) ;
#13995=LINE ( 'NONE', #23013, #34655 ) ;
#13996=ORIENTED_EDGE ( 'NONE', *, *, #31149, .F. ) ;
#14001=LINE ( 'NONE', #19699, #31110 ) ;
#14007=CARTESIAN_POINT ( 'NONE',  ( 2.789999999999999147, 0.000000000000000000, 0.000000000000000000 ) ) ;
#14010=CARTESIAN_POINT ( 'NONE',  ( -10.00000000000000000, 0.000000000000000000, 0.000000000000000000 ) ) ;
#14018=CARTESIAN_POINT ( 'NONE',  ( 0.07098925588714952162, -15.78394019282763239, 27.48475859319551873 ) ) ;
#14020=VERTEX_POINT ( 'NONE', #15139 ) ;
#14039=CARTESIAN_POINT ( 'NONE',  ( 0.1859802735910837668, -8.821517218319813836, -31.05303142369434966 ) ) ;
#14053=ORIENTED_EDGE ( 'NONE', *, *, #28775, .T. ) ;
#14056=ORIENTED_EDGE ( 'NONE', *, *, #27771, .T. ) ;
#14057=B_SPLINE_CURVE_WITH_KNOTS ( 'NONE', 3,
 ( #7505, #10018, #9839, #28541 ),
 .UNSPECIFIED., .F., .F.,
 ( 4, 4 ),
 ( 2.557638148638405956E-07, 0.0006879919438241684443 ),
 .UNSPECIFIED. ) ;
#14064=CARTESIAN_POINT ( 'NONE',  ( 2.789999999999999147, 28.95078156989571383, -9.502838467757751317 ) ) ;
#14065=VERTEX_POINT ( 'NONE', #22793 ) ;
#14067=FACE_OUTER_BOUND ( 'NONE', #9102, .T. ) ;
#14072=CARTESIAN_POINT ( 'NONE',  ( 0.006871061397808507845, -17.88422427744469090, 25.16112242373430874 ) ) ;
#14083=EDGE_CURVE ( 'NONE', #22788, #30647, #12530, .T. ) ;
#14085=AXIS2_PLACEMENT_3D ( 'NONE', #32682, #2428, #2606 ) ;
#14088=SHAPE_DEFINITION_REPRESENTATION ( #17203, #1195 ) ;
#14099=CARTESIAN_POINT ( 'NONE',  ( 0.5288002393074070495, 13.51471344666089003, 30.53246971302650081 ) ) ;
#14105=AXIS2_PLACEMENT_3D ( 'NONE', #32914, #19409, #30249 ) ;
#14107=DIRECTION ( 'NONE',  ( 0.000000000000000000, 1.374038396813312784E-15, -1.000000000000000000 ) ) ;
#14108=ORIENTED_EDGE ( 'NONE', *, *, #30449, .T. ) ;
#14119=ADVANCED_FACE ( 'NONE', ( #3905 ), #22627, .T. ) ;
#14122=ADVANCED_FACE ( 'NONE', ( #28481 ), #33465, .T. ) ;
#14126=CIRCLE ( 'NONE', #26061, 30.47050528711511674 ) ;
#14132=ADVANCED_FACE ( 'NONE', ( #4256 ), #6252, .T. ) ;
#14135=EDGE_LOOP ( 'NONE', ( #9793, #9224, #32055, #16010, #4932, #29903 ) ) ;
#14141=CARTESIAN_POINT ( 'NONE',  ( 1.749999999999999778, -1.891117961019737725, -34.36292081097834483 ) ) ;
#14148=EDGE_CURVE ( 'NONE', #11540, #13159, #1286, .T. ) ;
#14153=VERTEX_POINT ( 'NONE', #28824 ) ;
#14157=DIRECTION ( 'NONE',  ( -1.000000000000000000, 0.000000000000000000, 0.000000000000000000 ) ) ;
#14161=ORIENTED_EDGE ( 'NONE', *, *, #30668, .T. ) ;
#14162=B_SPLINE_CURVE_WITH_KNOTS ( 'NONE', 3,
 ( #12515, #4302, #33872, #7498, #31370, #20354 ),
 .UNSPECIFIED., .F., .F.,
 ( 4, 2, 4 ),
 ( 4.404817046682342164E-07, 0.001874269636018126642, 0.003748098790331584954 ),
 .UNSPECIFIED. ) ;
#14164=CARTESIAN_POINT ( 'NONE',  ( 2.265105744522721398, -28.86920449294081337, -16.75648442687151629 ) ) ;
#14190=CARTESIAN_POINT ( 'NONE',  ( -5.210000000000000853, 0.000000000000000000, 0.000000000000000000 ) ) ;
#14199=DIRECTION ( 'NONE',  ( 0.000000000000000000, 0.000000000000000000, 1.000000000000000000 ) ) ;
#14205=EDGE_CURVE ( 'NONE', #20230, #22483, #24517, .T. ) ;
#14214=ORIENTED_EDGE ( 'NONE', *, *, #12944, .F. ) ;
#14219=ORIENTED_EDGE ( 'NONE', *, *, #11715, .T. ) ;
#14220=CARTESIAN_POINT ( 'NONE',  ( 0.07094832863588811100, -8.452579892119532090, -30.54611582031341754 ) ) ;
#14223=CARTESIAN_POINT ( 'NONE',  ( 2.783107606170884818, 28.06690468450167586, 12.85275635055316457 ) ) ;
#14228=ORIENTED_EDGE ( 'NONE', *, *, #22145, .F. ) ;
#14229=B_SPLINE_CURVE_WITH_KNOTS ( 'NONE', 3,
 ( #7858, #5877, #391, #2515, #13913, #27603 ),
 .UNSPECIFIED., .F., .F.,
 ( 4, 2, 4 ),
 ( 4.404817033506925723E-07, 0.001874269626248501212, 0.003748098770793652050 ),
 .UNSPECIFIED. ) ;
#14232=DIRECTION ( 'NONE',  ( 0.000000000000000000, 0.000000000000000000, 1.000000000000000000 ) ) ;
#14234=B_SPLINE_CURVE_WITH_KNOTS ( 'NONE', 3,
 ( #13050, #8213, #3399, #13742 ),
 .UNSPECIFIED., .F., .F.,
 ( 4, 4 ),
 ( 0.005298345749243301393, 0.005985214453301814473 ),
 .UNSPECIFIED. ) ;
#14236=CARTESIAN_POINT ( 'NONE',  ( 2.789999999999999147, -23.41952779159748133, -19.49300927180569687 ) ) ;
#14239=CARTESIAN_POINT ( 'NONE',  ( 1.749999999999999778, -30.28730148581173864, 16.34215476954022606 ) ) ;
#14249=DIRECTION ( 'NONE',  ( 0.000000000000000000, 0.000000000000000000, 1.000000000000000000 ) ) ;
#14250=DIRECTION ( 'NONE',  ( -1.000000000000000000, -0.000000000000000000, -0.000000000000000000 ) ) ;
#14253=CARTESIAN_POINT ( 'NONE',  ( 8.000000000000000000, 0.000000000000000000, 0.000000000000000000 ) ) ;
#14260=ORIENTED_EDGE ( 'NONE', *, *, #18902, .T. ) ;
#14269=ADVANCED_FACE ( 'NONE', ( #28267 ), #12262, .T. ) ;
#14271=EDGE_CURVE ( 'NONE', #701, #1613, #12267, .T. ) ;
#14287=B_SPLINE_CURVE_WITH_KNOTS ( 'NONE', 3,
 ( #22558, #9023, #19891, #30732, #6858, #1185 ),
 .UNSPECIFIED., .F., .F.,
 ( 4, 2, 4 ),
 ( 1.989389909935507169E-07, 0.001873397232195059573, 0.003746595525399125815 ),
 .UNSPECIFIED. ) ;
#14302=AXIS2_PLACEMENT_3D ( 'NONE', #18539, #13363, #23847 ) ;
#14311=ORIENTED_EDGE ( 'NONE', *, *, #32890, .T. ) ;
#14313=ADVANCED_FACE ( 'NONE', ( #17775 ), #19951, .T. ) ;
#14322=DIRECTION ( 'NONE',  ( 0.000000000000000000, 0.000000000000000000, -1.000000000000000000 ) ) ;
#14326=DIRECTION ( 'NONE',  ( 1.000000000000000000, 0.000000000000000000, 0.000000000000000000 ) ) ;
#14330=CARTESIAN_POINT ( 'NONE',  ( 0.000000000000000000, 14.59907093257252164, -26.74544485249453274 ) ) ;
#14343=DIRECTION ( 'NONE',  ( 1.000000000000000000, -0.000000000000000000, -0.000000000000000000 ) ) ;
#14347=CARTESIAN_POINT ( 'NONE',  ( 2.765921099433444663, 29.44518845714764765, 9.980709654879525772 ) ) ;
#14348=EDGE_CURVE ( 'NONE', #33511, #28747, #17611, .T. ) ;
#14353=CARTESIAN_POINT ( 'NONE',  ( 1.040000000000000924, 0.000000000000000000, 0.000000000000000000 ) ) ;
#14356=VECTOR ( 'NONE', #17709, 1000.000000000000000 ) ;
#14357=TOROIDAL_SURFACE ( 'NONE', #3532, 30.47050528711511674, 8.000000000000000000 ) ;
#14362=DIRECTION ( 'NONE',  ( -1.000000000000000000, -0.000000000000000000, -0.000000000000000000 ) ) ;
#14363=DIRECTION ( 'NONE',  ( -1.000000000000000000, 0.000000000000000000, 0.000000000000000000 ) ) ;
#14369=CARTESIAN_POINT ( 'NONE',  ( 2.261199760692593319, 13.51471344666133412, -30.53246971302630541 ) ) ;
#14373=DIRECTION ( 'NONE',  ( -1.000000000000000000, -0.000000000000000000, -0.000000000000000000 ) ) ;
#14374=ADVANCED_FACE ( 'NONE', ( #25764 ), #14408, .T. ) ;
#14383=CIRCLE ( 'NONE', #154, 30.47050528711511674 ) ;
#14385=CIRCLE ( 'NONE', #26857, 34.41491905851385269 ) ;
#14388=B_SPLINE_CURVE_WITH_KNOTS ( 'NONE', 3,
 ( #9433, #31477, #10118, #12458 ),
 .UNSPECIFIED., .F., .F.,
 ( 4, 4 ),
 ( 2.010610498844539582E-07, 0.0006879367828357083612 ),
 .UNSPECIFIED. ) ;
#14395=LINE ( 'NONE', #16363, #6343 ) ;
#14396=ADVANCED_FACE ( 'NONE', ( #23958 ), #18136, .T. ) ;
#14398=EDGE_CURVE ( 'NONE', #22483, #23546, #25414, .T. ) ;
#14403=DIRECTION ( 'NONE',  ( 0.000000000000000000, 1.000000000000000000, 0.000000000000000000 ) ) ;
#14408=CYLINDRICAL_SURFACE ( 'NONE', #29025, 16.19999999999999574 ) ;
#14411=ORIENTED_EDGE ( 'NONE', *, *, #10117, .F. ) ;
#14415=DIRECTION ( 'NONE',  ( 1.000000000000000000, 0.000000000000000000, 0.000000000000000000 ) ) ;
#14418=EDGE_LOOP ( 'NONE', ( #33599, #19755, #27532, #31839 ) ) ;
#14448=DIRECTION ( 'NONE',  ( 0.000000000000000000, 0.000000000000000000, 1.000000000000000000 ) ) ;
#14449=VERTEX_POINT ( 'NONE', #4911 ) ;
#14457=VECTOR ( 'NONE', #6478, 1000.000000000000000 ) ;
#14463=CARTESIAN_POINT ( 'NONE',  ( 0.5288002500384482163, -23.80541455566215348, -23.41327456068897206 ) ) ;
#14473=DIRECTION ( 'NONE',  ( -1.000000000000000000, 0.000000000000000000, 0.000000000000000000 ) ) ;
#14475=CARTESIAN_POINT ( 'NONE',  ( 2.765921099433440666, -8.112136323388726922, -30.01377904834218668 ) ) ;
#14478=EDGE_CURVE ( 'NONE', #32274, #12335, #34137, .T. ) ;
#14486=VERTEX_POINT ( 'NONE', #9744 ) ;
#14487=ORIENTED_EDGE ( 'NONE', *, *, #22748, .F. ) ;
#14495=CARTESIAN_POINT ( 'NONE',  ( 2.789999999999999147, 2.005524111408653720, -31.87689292423236154 ) ) ;
#14505=DIRECTION ( 'NONE',  ( -1.000000000000000000, -0.000000000000000000, 0.000000000000000000 ) ) ;
#14514=CARTESIAN_POINT ( 'NONE',  ( 1.394999999999999574, -24.90160365674851661, -23.75493189058366994 ) ) ;
#14528=TOROIDAL_SURFACE ( 'NONE', #24734, 30.47050528711511674, 8.000000000000000000 ) ;
#14531=B_SPLINE_CURVE_WITH_KNOTS ( 'NONE', 3,
 ( #5719, #18763, #227, #8229 ),
 .UNSPECIFIED., .F., .F.,
 ( 4, 4 ),
 ( 1.991136383990097483E-07, 0.0006879348191047804937 ),
 .UNSPECIFIED. ) ;
#14541=CARTESIAN_POINT ( 'NONE',  ( 2.789999999999999147, -17.83604598421683107, 24.70480026434158916 ) ) ;
#14543=CARTESIAN_POINT ( 'NONE',  ( 1.040000000000001146, 34.10861917999622506, -4.581348211831715034 ) ) ;
#14551=AXIS2_PLACEMENT_3D ( 'NONE', #11164, #17223, #25372 ) ;
#14552=CARTESIAN_POINT ( 'NONE',  ( 2.765921099433440666, -8.112136323388726922, -30.01377904834218668 ) ) ;
#14562=( LENGTH_UNIT ( ) NAMED_UNIT ( * ) SI_UNIT ( .MILLI., .METRE. ) );
#14565=AXIS2_PLACEMENT_3D ( 'NONE', #6496, #3994, #12042 ) ;
#14566=EDGE_LOOP ( 'NONE', ( #293, #17264, #7118, #30593, #4694, #9381 ) ) ;
#14567=CARTESIAN_POINT ( 'NONE',  ( 2.765921099433441110, 14.63235270440936731, 27.43224275967444470 ) ) ;
#14593=CARTESIAN_POINT ( 'NONE',  ( 1.040000000000000924, 0.000000000000000000, 0.000000000000000000 ) ) ;
#14617=CIRCLE ( 'NONE', #30500, 2.524999999999999911 ) ;
#14625=AXIS2_PLACEMENT_3D ( 'NONE', #4970, #32554, #21370 ) ;
#14633=DIRECTION ( 'NONE',  ( -1.000000000000000000, -0.000000000000000000, -0.000000000000000000 ) ) ;
#14644=EDGE_CURVE ( 'NONE', #23263, #5461, #22182, .T. ) ;
#14646=ORIENTED_EDGE ( 'NONE', *, *, #1082, .F. ) ;
#14650=CARTESIAN_POINT ( 'NONE',  ( 2.789999999999999147, -31.68806325674604452, -4.003133335385915537 ) ) ;
#14653=CIRCLE ( 'NONE', #20329, 2.524999999999999911 ) ;
#14654=AXIS2_PLACEMENT_3D ( 'NONE', #31726, #26739, #7334 ) ;
#14661=TOROIDAL_SURFACE ( 'NONE', #12389, 30.47050528711511674, 8.000000000000000000 ) ;
#14665=CIRCLE ( 'NONE', #16931, 2.525000000000000799 ) ;
#14666=ORIENTED_EDGE ( 'NONE', *, *, #16264, .T. ) ;
#14675=VERTEX_POINT ( 'NONE', #8475 ) ;
#14680=CARTESIAN_POINT ( 'NONE',  ( 1.040000000000000924, 0.000000000000000000, 0.000000000000000000 ) ) ;
#14681=DIRECTION ( 'NONE',  ( -1.000000000000000000, 0.000000000000000000, 0.000000000000000000 ) ) ;
#14683=CARTESIAN_POINT ( 'NONE',  ( 0.000000000000000000, 17.98401995359670025, -24.59729088254937324 ) ) ;
#14684=CARTESIAN_POINT ( 'NONE',  ( 0.000000000000000000, 27.60935207499554522, 12.89090262359660422 ) ) ;
#14685=CARTESIAN_POINT ( 'NONE',  ( 2.790000000000083080, 29.09328061627297757, 9.684256520155898329 ) ) ;
#14686=ORIENTED_EDGE ( 'NONE', *, *, #14644, .F. ) ;
#14693=FACE_OUTER_BOUND ( 'NONE', #25617, .T. ) ;
#14698=AXIS2_PLACEMENT_3D ( 'NONE', #3083, #13961, #24796 ) ;
#14701=B_SPLINE_CURVE_WITH_KNOTS ( 'NONE', 3,
 ( #32140, #24291, #12943, #32311, #26978, #19162 ),
 .UNSPECIFIED., .F., .F.,
 ( 4, 2, 4 ),
 ( 4.404817164018835850E-07, 0.001874269726455596438, 0.003748098971194791310 ),
 .UNSPECIFIED. ) ;
#14702=CARTESIAN_POINT ( 'NONE',  ( -8.304372355306091180E-14, 20.82920972943067284, -22.50217193233280000 ) ) ;
#14706=VERTEX_POINT ( 'NONE', #6315 ) ;
#14709=CARTESIAN_POINT ( 'NONE',  ( 1.040000000000000924, 0.000000000000000000, 0.000000000000000000 ) ) ;
#14715=ORIENTED_EDGE ( 'NONE', *, *, #681, .F. ) ;
#14718=CARTESIAN_POINT ( 'NONE',  ( 0.07094834062134731945, -11.11627562454433082, 29.68062877649318665 ) ) ;
#14724=CARTESIAN_POINT ( 'NONE',  ( 1.040000000000001368, 6.714005886385424837, -33.75364837705166110 ) ) ;
#14728=CARTESIAN_POINT ( 'NONE',  ( 2.789999999999999147, -30.41598411195409923, 1.821977758773558165 ) ) ;
#14739=VERTEX_POINT ( 'NONE', #25545 ) ;
#14746=CARTESIAN_POINT ( 'NONE',  ( 2.604019706987809712, 14.82665350068097254, 28.67542985682328549 ) ) ;
#14761=ORIENTED_EDGE ( 'NONE', *, *, #3010, .F. ) ;
#14763=CARTESIAN_POINT ( 'NONE',  ( 0.000000000000000000, 30.93646776788807173, -7.943134866715984899 ) ) ;
#14776=CARTESIAN_POINT ( 'NONE',  ( 2.719051671364112632, -8.452579892119949534, 30.54611582031328609 ) ) ;
#14778=EDGE_CURVE ( 'NONE', #29101, #11797, #17130, .T. ) ;
#14781=CARTESIAN_POINT ( 'NONE',  ( 2.789999999999999147, -11.13185981125856827, -28.36429779836962339 ) ) ;
#14787=CARTESIAN_POINT ( 'NONE',  ( 1.040000000000000702, 22.14447232807505728, 26.34405054495564968 ) ) ;
#14793=ORIENTED_EDGE ( 'NONE', *, *, #22851, .F. ) ;
#14795=EDGE_CURVE ( 'NONE', #26863, #11290, #15875, .T. ) ;
#14796=EDGE_CURVE ( 'NONE', #9427, #5512, #9167, .T. ) ;
#14813=EDGE_CURVE ( 'NONE', #10508, #22962, #20527, .T. ) ;
#14817=EDGE_CURVE ( 'NONE', #916, #33934, #24345, .T. ) ;
#14818=FACE_OUTER_BOUND ( 'NONE', #8947, .T. ) ;
#14830=VERTEX_POINT ( 'NONE', #20908 ) ;
#14842=EDGE_CURVE ( 'NONE', #25806, #15766, #23401, .T. ) ;
#14843=ORIENTED_EDGE ( 'NONE', *, *, #28523, .F. ) ;
#14850=FACE_OUTER_BOUND ( 'NONE', #11861, .T. ) ;
#14860=VERTEX_POINT ( 'NONE', #31243 ) ;
#14871=FACE_OUTER_BOUND ( 'NONE', #15956, .T. ) ;
#14872=CARTESIAN_POINT ( 'NONE',  ( 1.749999999999999778, 0.000000000000000000, 0.000000000000000000 ) ) ;
#14894=DIRECTION ( 'NONE',  ( 0.000000000000000000, 0.000000000000000000, 1.000000000000000000 ) ) ;
#14898=DIRECTION ( 'NONE',  ( 0.000000000000000000, 0.000000000000000000, 1.000000000000000000 ) ) ;
#14904=CARTESIAN_POINT ( 'NONE',  ( 2.789999999999999591, -11.08319859408639374, 28.58839307351509618 ) ) ;
#14912=VECTOR ( 'NONE', #7262, 1000.000000000000000 ) ;
#14917=CARTESIAN_POINT ( 'NONE',  ( 0.02407890056655695096, 20.99477179376825120, 22.93149026599753526 ) ) ;
#14919=EDGE_CURVE ( 'NONE', #34651, #19524, #26205, .T. ) ;
#14923=CARTESIAN_POINT ( 'NONE',  ( -10.00000000000000000, 0.000000000000000000, 0.000000000000000000 ) ) ;
#14930=VERTEX_POINT ( 'NONE', #2041 ) ;
#14935=CARTESIAN_POINT ( 'NONE',  ( 0.7561992069920354664, 27.74641878906462722, 19.50321439924967848 ) ) ;
#14936=DIRECTION ( 'NONE',  ( -1.000000000000000000, -0.000000000000000000, -0.000000000000000000 ) ) ;
#14941=CARTESIAN_POINT ( 'NONE',  ( 0.07094832566281392139, 19.10378521888243597, 25.28945800968172009 ) ) ;
#14944=EDGE_LOOP ( 'NONE', ( #29611, #32309, #34531, #27783 ) ) ;
#14947=CARTESIAN_POINT ( 'NONE',  ( 2.765921099433442887, -8.112136323389137260, 30.01377904834206589 ) ) ;
#14948=LINE ( 'NONE', #28460, #723 ) ;
#14953=CARTESIAN_POINT ( 'NONE',  ( 0.1835381641992968882, -0.8174345826532598558, 32.26081300283360065 ) ) ;
#14959=VERTEX_POINT ( 'NONE', #8251 ) ;
#14961=AXIS2_PLACEMENT_3D ( 'NONE', #13548, #35087, #19075 ) ;
#14966=EDGE_CURVE ( 'NONE', #9840, #13324, #7769, .T. ) ;
#14980=ORIENTED_EDGE ( 'NONE', *, *, #9768, .T. ) ;
#14981=DIRECTION ( 'NONE',  ( 1.000000000000000000, 0.000000000000000000, 0.000000000000000000 ) ) ;
#14985=CARTESIAN_POINT ( 'NONE',  ( 2.789999999999999591, -21.14855567236443434, -22.20072382163073854 ) ) ;
#14991=CYLINDRICAL_SURFACE ( 'NONE', #9860, 2.524999999999999467 ) ;
#14995=DIRECTION ( 'NONE',  ( 0.000000000000000000, 0.000000000000000000, 1.000000000000000000 ) ) ;
#14996=ORIENTED_EDGE ( 'NONE', *, *, #29727, .F. ) ;
#14997=CARTESIAN_POINT ( 'NONE',  ( 2.033800785921083154, -9.974544214302445866, -32.41523709743442083 ) ) ;
#14998=CARTESIAN_POINT ( 'NONE',  ( 0.02407890056655695096, -26.45933846664182099, -16.32596387352474565 ) ) ;
#15000=ORIENTED_EDGE ( 'NONE', *, *, #15125, .F. ) ;
#15002=ADVANCED_FACE ( 'NONE', ( #2555 ), #30139, .F. ) ;
#15004=VECTOR ( 'NONE', #14343, 1000.000000000000000 ) ;
#15005=EDGE_CURVE ( 'NONE', #8559, #3111, #11431, .T. ) ;
#15029=ORIENTED_EDGE ( 'NONE', *, *, #6086, .F. ) ;
#15031=CARTESIAN_POINT ( 'NONE',  ( 0.7561992264529545649, -32.71371797491577382, 8.947166372574571369 ) ) ;
#15046=CARTESIAN_POINT ( 'NONE',  ( 0.1859802928572567293, -3.229344000442754048, 32.11979559073828483 ) ) ;
#15056=VERTEX_POINT ( 'NONE', #10590 ) ;
#15058=CARTESIAN_POINT ( 'NONE',  ( 1.749999999999999778, 0.000000000000000000, 0.000000000000000000 ) ) ;
#15065=ORIENTED_EDGE ( 'NONE', *, *, #28202, .T. ) ;
#15067=CARTESIAN_POINT ( 'NONE',  ( 2.789999999999999147, 27.98916443103621177, -12.86217335695007868 ) ) ;
#15071=CARTESIAN_POINT ( 'NONE',  ( 1.039999999999999591, 31.89769921722987434, 12.91988538846969803 ) ) ;
#15072=ORIENTED_EDGE ( 'NONE', *, *, #12125, .F. ) ;
#15075=CARTESIAN_POINT ( 'NONE',  ( 0.5288002586553935958, 33.02096244749627374, 4.949265406682166635 ) ) ;
#15078=DIRECTION ( 'NONE',  ( 0.000000000000000000, 0.000000000000000000, 1.000000000000000000 ) ) ;
#15100=B_SPLINE_CURVE_WITH_KNOTS ( 'NONE', 3,
 ( #7918, #2572, #21793, #8270 ),
 .UNSPECIFIED., .F., .F.,
 ( 4, 4 ),
 ( 0.005298352430873754307, 0.005985221104152186646 ),
 .UNSPECIFIED. ) ;
#15101=CARTESIAN_POINT ( 'NONE',  ( 1.039999999999999813, -30.02688531850407117, 16.81585001935569323 ) ) ;
#15115=DIRECTION ( 'NONE',  ( -1.000000000000000000, -0.000000000000000000, -0.000000000000000000 ) ) ;
#15119=DIRECTION ( 'NONE',  ( -1.000000000000000000, -0.000000000000000000, -0.000000000000000000 ) ) ;
#15125=EDGE_CURVE ( 'NONE', #29665, #22708, #8574, .T. ) ;
#15129=CARTESIAN_POINT ( 'NONE',  ( 0.006892386950099134262, -26.23471115434894685, 16.26912442529598835 ) ) ;
#15134=VERTEX_POINT ( 'NONE', #19660 ) ;
#15136=ORIENTED_EDGE ( 'NONE', *, *, #19165, .T. ) ;
#15137=CIRCLE ( 'NONE', #28771, 2.525000000000001688 ) ;
#15139=CARTESIAN_POINT ( 'NONE',  ( 2.765921099433441555, 24.20451283648857554, -19.51346322004903300 ) ) ;
#15143=DIRECTION ( 'NONE',  ( -1.000000000000000000, -0.000000000000000000, -0.000000000000000000 ) ) ;
#15149=EDGE_LOOP ( 'NONE', ( #31945, #30896, #8639, #10064 ) ) ;
#15159=B_SPLINE_CURVE_WITH_KNOTS ( 'NONE', 3,
 ( #20790, #7244, #31984, #15459 ),
 .UNSPECIFIED., .F., .F.,
 ( 4, 4 ),
 ( 2.876507994514687179E-07, 0.0006880240977454715181 ),
 .UNSPECIFIED. ) ;
#15168=CARTESIAN_POINT ( 'NONE',  ( 2.789999999999999147, -25.77598557799237255, -16.24962337825830616 ) ) ;
#15180=CARTESIAN_POINT ( 'NONE',  ( 2.765921099433441999, -21.56796757982826307, 22.39322359481599278 ) ) ;
#15184=DIRECTION ( 'NONE',  ( 0.000000000000000000, 0.000000000000000000, -1.000000000000000000 ) ) ;
#15191=DIRECTION ( 'NONE',  ( 0.000000000000000000, 0.000000000000000000, 1.000000000000000000 ) ) ;
#15198=DIRECTION ( 'NONE',  ( -1.000000000000000000, -0.000000000000000000, -0.000000000000000000 ) ) ;
#15203=DIRECTION ( 'NONE',  ( -1.000000000000000000, -0.000000000000000000, -0.000000000000000000 ) ) ;
#15208=CARTESIAN_POINT ( 'NONE',  ( -1.120881116509116332E-15, 14.57887998322625300, 26.97387222978633403 ) ) ;
#15211=EDGE_CURVE ( 'NONE', #5830, #10504, #23470, .T. ) ;
#15228=DIRECTION ( 'NONE',  ( -1.000000000000000000, -0.000000000000000000, -0.000000000000000000 ) ) ;
#15233=EDGE_CURVE ( 'NONE', #33936, #17530, #3493, .T. ) ;
#15254=VECTOR ( 'NONE', #550, 1000.000000000000000 ) ;
#15256=EDGE_CURVE ( 'NONE', #28359, #29908, #14162, .T. ) ;
#15276=B_SPLINE_CURVE_WITH_KNOTS ( 'NONE', 3,
 ( #9989, #31012, #23515, #9477, #31350, #14998 ),
 .UNSPECIFIED., .F., .F.,
 ( 4, 2, 4 ),
 ( 4.404817019028824490E-07, 0.001874269618538360743, 0.003748098755374818306 ),
 .UNSPECIFIED. ) ;
#15278=CARTESIAN_POINT ( 'NONE',  ( 0.07098932382052611234, -27.07245655034587628, 16.48110659958382129 ) ) ;
#15285=ORIENTED_EDGE ( 'NONE', *, *, #33301, .T. ) ;
#15286=CARTESIAN_POINT ( 'NONE',  ( 8.000000000000000000, 0.000000000000000000, 0.000000000000000000 ) ) ;
#15287=EDGE_CURVE ( 'NONE', #22184, #4601, #10899, .T. ) ;
#15289=CARTESIAN_POINT ( 'NONE',  ( 2.765921099433444219, 31.00221527374952046, 2.344426712874309260 ) ) ;
#15292=B_SPLINE_CURVE_WITH_KNOTS ( 'NONE', 3,
 ( #8892, #30785, #17630, #14781 ),
 .UNSPECIFIED., .F., .F.,
 ( 4, 4 ),
 ( 1.979774382698227165E-07, 0.0006879336733830483793 ),
 .UNSPECIFIED. ) ;
#15299=CARTESIAN_POINT ( 'NONE',  ( 1.749999999999999778, -25.27164158951585549, 23.36088151536907631 ) ) ;
#15304=FACE_OUTER_BOUND ( 'NONE', #25134, .T. ) ;
#15308=AXIS2_PLACEMENT_3D ( 'NONE', #20621, #15115, #29149 ) ;
#15315=EDGE_CURVE ( 'NONE', #6398, #14065, #10752, .T. ) ;
#15324=CARTESIAN_POINT ( 'NONE',  ( 1.749999999999999778, -2.430610048906265419, 34.32897884578299852 ) ) ;
#15330=FACE_OUTER_BOUND ( 'NONE', #13262, .T. ) ;
#15334=B_SPLINE_CURVE_WITH_KNOTS ( 'NONE', 3,
 ( #24991, #16486, #18468, #3109 ),
 .UNSPECIFIED., .F., .F.,
 ( 4, 4 ),
 ( 0.002009632881715329999, 0.003746595525399130586 ),
 .UNSPECIFIED. ) ;
#15341=AXIS2_PLACEMENT_3D ( 'NONE', #9628, #28324, #17494 ) ;
#15344=CARTESIAN_POINT ( 'NONE',  ( 0.006915246992955798207, 27.98916443103565399, -12.86217335695007868 ) ) ;
#15347=B_SPLINE_CURVE_WITH_KNOTS ( 'NONE', 3,
 ( #24586, #27794, #21934, #32950, #8751, #16794 ),
 .UNSPECIFIED., .F., .F.,
 ( 4, 2, 4 ),
 ( 2.126639591840295689E-07, 0.001873410972133593942, 0.003746609280308003942 ),
 .UNSPECIFIED. ) ;
#15362=CARTESIAN_POINT ( 'NONE',  ( 1.749999999999999778, -30.02688531850407472, 16.81585001935568613 ) ) ;
#15378=DIRECTION ( 'NONE',  ( -1.000000000000000000, -0.000000000000000000, -0.000000000000000000 ) ) ;
#15380=AXIS2_PLACEMENT_3D ( 'NONE', #24392, #3033, #19608 ) ;
#15382=DIRECTION ( 'NONE',  ( -1.000000000000000000, -0.000000000000000000, -0.000000000000000000 ) ) ;
#15384=LINE ( 'NONE', #13065, #20139 ) ;
#15392=EDGE_LOOP ( 'NONE', ( #18687, #20356, #25768, #8900 ) ) ;
#15393=EDGE_CURVE ( 'NONE', #19998, #9840, #29846, .T. ) ;
#15398=ADVANCED_FACE ( 'NONE', ( #19224 ), #27563, .T. ) ;
#15402=DIRECTION ( 'NONE',  ( -1.000000000000000000, -0.000000000000000000, -0.000000000000000000 ) ) ;
#15407=ORIENTED_EDGE ( 'NONE', *, *, #30261, .F. ) ;
#15408=CARTESIAN_POINT ( 'NONE',  ( 2.789999999999999147, 2.005524111408194088, 31.87689292423238996 ) ) ;
#15410=FACE_OUTER_BOUND ( 'NONE', #2796, .T. ) ;
#15417=AXIS2_PLACEMENT_3D ( 'NONE', #1822, #20524, #28540 ) ;
#15418=DIRECTION ( 'NONE',  ( 0.000000000000000000, 0.000000000000000000, 1.000000000000000000 ) ) ;
#15422=CARTESIAN_POINT ( 'NONE',  ( 2.261199740906818079, -11.04911166161924285, -31.50867056184630854 ) ) ;
#15429=DIRECTION ( 'NONE',  ( 0.000000000000000000, 0.000000000000000000, 1.000000000000000000 ) ) ;
#15430=DIRECTION ( 'NONE',  ( 0.000000000000000000, 0.000000000000000000, 1.000000000000000000 ) ) ;
#15431=CARTESIAN_POINT ( 'NONE',  ( 0.000000000000000000, -29.00730259674847034, 9.328884633908835156 ) ) ;
#15439=VECTOR ( 'NONE', #29691, 1000.000000000000000 ) ;
#15440=AXIS2_PLACEMENT_3D ( 'NONE', #31401, #33904, #4989 ) ;
#15443=ORIENTED_EDGE ( 'NONE', *, *, #16299, .T. ) ;
#15449=EDGE_CURVE ( 'NONE', #31622, #34030, #7315, .T. ) ;
#15454=CARTESIAN_POINT ( 'NONE',  ( 2.790000000000080860, 23.76564585743019720, -19.37518496788493039 ) ) ;
#15459=CARTESIAN_POINT ( 'NONE',  ( 0.000000000000000000, -27.53147453683434520, 13.05640081644832939 ) ) ;
#15461=ORIENTED_EDGE ( 'NONE', *, *, #3652, .F. ) ;
#15464=CARTESIAN_POINT ( 'NONE',  ( 0.5288002398009233884, 27.45925096103277241, -18.99654502929918465 ) ) ;
#15465=EDGE_CURVE ( 'NONE', #6886, #8440, #13689, .T. ) ;
#15469=TOROIDAL_SURFACE ( 'NONE', #31921, 30.47050528711511674, 8.000000000000000000 ) ;
#15470=AXIS2_PLACEMENT_3D ( 'NONE', #8106, #16491, #32139 ) ;
#15474=VECTOR ( 'NONE', #11224, 1000.000000000000000 ) ;
#15475=FACE_OUTER_BOUND ( 'NONE', #14566, .T. ) ;
#15481=CARTESIAN_POINT ( 'NONE',  ( 0.000000000000000000, -0.09145294252657359957, -30.47036804522409525 ) ) ;
#15493=CARTESIAN_POINT ( 'NONE',  ( 0.000000000000000000, 0.000000000000000000, 0.000000000000000000 ) ) ;
#15494=CARTESIAN_POINT ( 'NONE',  ( 2.033800778447012014, 27.12277411069248245, 20.36158770325061695 ) ) ;
#15500=CYLINDRICAL_SURFACE ( 'NONE', #8438, 16.19999999999999929 ) ;
#15515=CIRCLE ( 'NONE', #22909, 30.47050528711512030 ) ;
#15518=CARTESIAN_POINT ( 'NONE',  ( 0.02407890056655738464, 28.29688452313417812, -12.88099432405573630 ) ) ;
#15519=DIRECTION ( 'NONE',  ( 1.000000000000000000, 0.000000000000000000, 0.000000000000000000 ) ) ;
#15520=ORIENTED_EDGE ( 'NONE', *, *, #14796, .F. ) ;
#15526=ORIENTED_EDGE ( 'NONE', *, *, #21739, .T. ) ;
#15534=VERTEX_POINT ( 'NONE', #22586 ) ;
#15547=CARTESIAN_POINT ( 'NONE',  ( 0.1835380628080924836, -24.33633102984340724, -21.19365992153305100 ) ) ;
#15558=EDGE_CURVE ( 'NONE', #22891, #25011, #6367, .T. ) ;
#15574=CARTESIAN_POINT ( 'NONE',  ( 1.394999999999999574, -10.89151784028265801, -32.64600270996228204 ) ) ;
#15592=CARTESIAN_POINT ( 'NONE',  ( 1.040000000000000924, -18.66807150955393624, -28.91175816027522316 ) ) ;
#15596=CARTESIAN_POINT ( 'NONE',  ( 1.394999999999999574, 14.89726405156217126, 31.02351007835983054 ) ) ;
#15597=DIRECTION ( 'NONE',  ( 0.000000000000000000, 0.000000000000000000, 1.000000000000000000 ) ) ;
#15598=EDGE_CURVE ( 'NONE', #10504, #23746, #20001, .T. ) ;
#15599=CARTESIAN_POINT ( 'NONE',  ( 2.765921099434983876, -15.32140196853734970, -27.05343472113007763 ) ) ;
#15602=ORIENTED_EDGE ( 'NONE', *, *, #18488, .F. ) ;
#15619=AXIS2_PLACEMENT_3D ( 'NONE', #933, #11433, #19457 ) ;
#15631=ORIENTED_EDGE ( 'NONE', *, *, #34381, .F. ) ;
#15634=CARTESIAN_POINT ( 'NONE',  ( 0.000000000000000000, -29.69698570178027808, 11.75786841620004175 ) ) ;
#15635=VECTOR ( 'NONE', #27114, 1000.000000000000000 ) ;
#15639=CYLINDRICAL_SURFACE ( 'NONE', #27203, 2.524999999999999467 ) ;
#15646=EDGE_LOOP ( 'NONE', ( #3778, #15136, #25428, #23992 ) ) ;
#15650=VERTEX_POINT ( 'NONE', #10274 ) ;
#15662=AXIS2_PLACEMENT_3D ( 'NONE', #5692, #32760, #21732 ) ;
#15666=ORIENTED_EDGE ( 'NONE', *, *, #10132, .F. ) ;
#15680=FACE_OUTER_BOUND ( 'NONE', #23977, .T. ) ;
#15681=CARTESIAN_POINT ( 'NONE',  ( 2.606461809142830433, -3.232363112765826330, 32.10887868570996773 ) ) ;
#15691=CIRCLE ( 'NONE', #14551, 34.41491905851385269 ) ;
#15704=CARTESIAN_POINT ( 'NONE',  ( 2.783128901175710990, 18.40312061469657579, -24.78412275958813282 ) ) ;
#15710=CARTESIAN_POINT ( 'NONE',  ( 2.789999999999999147, 25.67797970382134309, 16.40405592474765939 ) ) ;
#15715=DIRECTION ( 'NONE',  ( 0.000000000000000000, 0.000000000000000000, 1.000000000000000000 ) ) ;
#15718=B_SPLINE_CURVE_WITH_KNOTS ( 'NONE', 3,
 ( #22660, #9115, #19983, #30835 ),
 .UNSPECIFIED., .F., .F.,
 ( 4, 4 ),
 ( 3.087659402431792624E-07, 0.0006880453895802092143 ),
 .UNSPECIFIED. ) ;
#15719=EDGE_CURVE ( 'NONE', #30318, #17643, #25578, .T. ) ;
#15723=ORIENTED_EDGE ( 'NONE', *, *, #10412, .T. ) ;
#15725=CARTESIAN_POINT ( 'NONE',  ( 0.006871111354928813829, 25.89075856630370964, -16.81059844634632228 ) ) ;
#15727=EDGE_CURVE ( 'NONE', #10508, #23413, #32502, .T. ) ;
#15728=LINE ( 'NONE', #29585, #8493 ) ;
#15730=DIRECTION ( 'NONE',  ( -1.000000000000000000, 0.000000000000000000, 0.000000000000000000 ) ) ;
#15734=B_SPLINE_CURVE_WITH_KNOTS ( 'NONE', 3,
 ( #11946, #6400, #3384, #19780, #1251, #22443 ),
 .UNSPECIFIED., .F., .F.,
 ( 4, 2, 4 ),
 ( 2.570076372303527286E-07, 0.001873455364168429135, 0.003746653720699627977 ),
 .UNSPECIFIED. ) ;
#15736=FACE_OUTER_BOUND ( 'NONE', #5561, .T. ) ;
#15739=CARTESIAN_POINT ( 'NONE',  ( 0.000000000000000000, -23.41952779159775488, 19.49300927180538778 ) ) ;
#15740=CARTESIAN_POINT ( 'NONE',  ( 0.000000000000000000, 0.000000000000000000, 0.000000000000000000 ) ) ;
#15754=CARTESIAN_POINT ( 'NONE',  ( 2.765921099433443331, -29.68817180695682723, 9.232883799364120847 ) ) ;
#15764=DIRECTION ( 'NONE',  ( -1.000000000000000000, -0.000000000000000000, -0.000000000000000000 ) ) ;
#15766=VERTEX_POINT ( 'NONE', #32330 ) ;
#15770=DIRECTION ( 'NONE',  ( 0.000000000000000000, 0.000000000000000000, 1.000000000000000000 ) ) ;
#15773=ORIENTED_EDGE ( 'NONE', *, *, #18038, .T. ) ;
#15776=ORIENTED_EDGE ( 'NONE', *, *, #15256, .T. ) ;
#15783=ORIENTED_EDGE ( 'NONE', *, *, #16342, .T. ) ;
#15786=B_SPLINE_CURVE_WITH_KNOTS ( 'NONE', 3,
 ( #15961, #27496, #2928, #14164, #7927, #29996 ),
 .UNSPECIFIED., .F., .F.,
 ( 4, 2, 4 ),
 ( 2.036796643443874831E-07, 0.001873401978039412061, 0.003746600276414479517 ),
 .UNSPECIFIED. ) ;
#15791=CIRCLE ( 'NONE', #31661, 34.41491905851385269 ) ;
#15792=B_SPLINE_CURVE_WITH_KNOTS ( 'NONE', 3,
 ( #21462, #32131, #13107, #10611 ),
 .UNSPECIFIED., .F., .F.,
 ( 4, 4 ),
 ( 0.001749480761540356689, 0.003748098735642882602 ),
 .UNSPECIFIED. ) ;
#15810=CARTESIAN_POINT ( 'NONE',  ( 2.789999999999999147, 0.000000000000000000, 0.000000000000000000 ) ) ;
#15823=ORIENTED_EDGE ( 'NONE', *, *, #16935, .T. ) ;
#15826=CARTESIAN_POINT ( 'NONE',  ( 2.789999999999999147, 30.27116788629744804, -3.198253332533264714 ) ) ;
#15852=ORIENTED_EDGE ( 'NONE', *, *, #10167, .T. ) ;
#15855=EDGE_CURVE ( 'NONE', #14675, #15650, #31508, .T. ) ;
#15859=VECTOR ( 'NONE', #6975, 1000.000000000000000 ) ;
#15863=EDGE_CURVE ( 'NONE', #17221, #11449, #32425, .T. ) ;
#15865=ORIENTED_EDGE ( 'NONE', *, *, #15598, .T. ) ;
#15867=CARTESIAN_POINT ( 'NONE',  ( 0.02407890056655695096, -21.56796757982795043, -22.39322359481629476 ) ) ;
#15874=B_SPLINE_CURVE_WITH_KNOTS ( 'NONE', 3,
 ( #14683, #33349, #28539, #8970 ),
 .UNSPECIFIED., .F., .F.,
 ( 4, 4 ),
 ( 0.005298349227682462234, 0.005985217865144625352 ),
 .UNSPECIFIED. ) ;
#15875=B_SPLINE_CURVE_WITH_KNOTS ( 'NONE', 3,
 ( #6677, #822, #3651, #3995, #25725, #14543 ),
 .UNSPECIFIED., .F., .F.,
 ( 4, 2, 4 ),
 ( 1.991142096567452048E-07, 0.001873397407604851950, 0.003746595701000047206 ),
 .UNSPECIFIED. ) ;
#15879=CARTESIAN_POINT ( 'NONE',  ( 2.719051661303893752, -27.07192087577324102, 16.48097105307871502 ) ) ;
#15885=FACE_OUTER_BOUND ( 'NONE', #4374, .T. ) ;
#15887=AXIS2_PLACEMENT_3D ( 'NONE', #18614, #23920, #29625 ) ;
#15900=TOROIDAL_SURFACE ( 'NONE', #7049, 30.47050528711511674, 8.000000000000000000 ) ;
#15911=CARTESIAN_POINT ( 'NONE',  ( 2.783107617110828880, 23.98878059851154632, 19.42891868047417958 ) ) ;
#15918=DIRECTION ( 'NONE',  ( 0.000000000000000000, -0.3681245526846723126, -0.9297764858882535677 ) ) ;
#15920=DIRECTION ( 'NONE',  ( -1.000000000000000000, -0.000000000000000000, -0.000000000000000000 ) ) ;
#15928=AXIS2_PLACEMENT_3D ( 'NONE', #14923, #684, #6709 ) ;
#15937=DIRECTION ( 'NONE',  ( -1.000000000000000000, 0.000000000000000000, 0.000000000000000000 ) ) ;
#15941=FACE_OUTER_BOUND ( 'NONE', #23906, .T. ) ;
#15945=CARTESIAN_POINT ( 'NONE',  ( 1.395000000000002238, -2.430610048906255649, 34.32897884578299852 ) ) ;
#15948=ORIENTED_EDGE ( 'NONE', *, *, #2592, .T. ) ;
#15949=CIRCLE ( 'NONE', #25005, 34.41491905851385269 ) ;
#15956=EDGE_LOOP ( 'NONE', ( #23832, #26064, #32243, #2282 ) ) ;
#15961=CARTESIAN_POINT ( 'NONE',  ( 2.765921099433443775, -26.45933846664182099, -16.32596387352474565 ) ) ;
#15980=ORIENTED_EDGE ( 'NONE', *, *, #11984, .T. ) ;
#15981=VECTOR ( 'NONE', #31100, 1000.000000000000000 ) ;
#15986=CYLINDRICAL_SURFACE ( 'NONE', #23057, 16.19999999999999574 ) ;
#15988=DIRECTION ( 'NONE',  ( 1.000000000000000000, 0.000000000000000000, 0.000000000000000000 ) ) ;
#15991=CIRCLE ( 'NONE', #23908, 30.47050528711512030 ) ;
#15992=CARTESIAN_POINT ( 'NONE',  ( 0.5248941363854600084, 20.67343389904918993, -26.20724806577283061 ) ) ;
#15994=CARTESIAN_POINT ( 'NONE',  ( 2.765921099433442443, 28.29688452313417812, -12.88099432405573630 ) ) ;
#15999=EDGE_CURVE ( 'NONE', #17643, #17012, #28530, .T. ) ;
#16010=ORIENTED_EDGE ( 'NONE', *, *, #28775, .F. ) ;
#16016=LINE ( 'NONE', #30054, #26583 ) ;
#16018=LINE ( 'NONE', #2464, #6744 ) ;
#16025=CARTESIAN_POINT ( 'NONE',  ( 2.606461795830078643, -11.11596589742349295, 30.29626325691701183 ) ) ;
#16036=ORIENTED_EDGE ( 'NONE', *, *, #4672, .F. ) ;
#16045=CARTESIAN_POINT ( 'NONE',  ( 2.789999999999999147, -5.984944020946091570, 31.37417528048439763 ) ) ;
#16049=CARTESIAN_POINT ( 'NONE',  ( 1.749999999999999778, 6.183021911001840287, 33.85493898757064812 ) ) ;
#16055=ADVANCED_FACE ( 'NONE', ( #22550 ), #11696, .T. ) ;
#16072=CARTESIAN_POINT ( 'NONE',  ( 2.789999999999999147, 27.60935207499570154, -12.89090262359623118 ) ) ;
#16073=CARTESIAN_POINT ( 'NONE',  ( 0.000000000000000000, -29.00730259674833178, -9.328884633909240165 ) ) ;
#16075=LINE ( 'NONE', #24405, #25079 ) ;
#16082=AXIS2_PLACEMENT_3D ( 'NONE', #34598, #25886, #7002 ) ;
#16086=CYLINDRICAL_SURFACE ( 'NONE', #3649, 2.525000000000000799 ) ;
#16088=DIRECTION ( 'NONE',  ( 1.000000000000000000, 0.000000000000000000, 0.000000000000000000 ) ) ;
#16094=VERTEX_POINT ( 'NONE', #15071 ) ;
#16095=EDGE_CURVE ( 'NONE', #5845, #19421, #4015, .T. ) ;
#16107=CARTESIAN_POINT ( 'NONE',  ( 2.783084753007022627, 27.98916443103619045, -12.86217335695007868 ) ) ;
#16111=ORIENTED_EDGE ( 'NONE', *, *, #31700, .F. ) ;
#16115=EDGE_CURVE ( 'NONE', #34702, #31399, #12923, .T. ) ;
#16128=ORIENTED_EDGE ( 'NONE', *, *, #25841, .F. ) ;
#16137=CARTESIAN_POINT ( 'NONE',  ( 0.02407890056655738464, -11.07880054387200985, -29.04985141099774637 ) ) ;
#16141=CARTESIAN_POINT ( 'NONE',  ( 2.765921099433442887, -8.112136323389137260, 30.01377904834206589 ) ) ;
#16147=ORIENTED_EDGE ( 'NONE', *, *, #30836, .F. ) ;
#16150=AXIS2_PLACEMENT_3D ( 'NONE', #26924, #22122, #8412 ) ;
#16163=CARTESIAN_POINT ( 'NONE',  ( 2.789999999999999147, 30.27116788629744804, -3.198253332533264714 ) ) ;
#16164=CARTESIAN_POINT ( 'NONE',  ( 2.719051666187956684, 4.557485336350932670, -31.36463980626626835 ) ) ;
#16168=CARTESIAN_POINT ( 'NONE',  ( 0.07098928307139744376, 19.10423307544374438, -25.28978101402028145 ) ) ;
#16175=ORIENTED_EDGE ( 'NONE', *, *, #21401, .T. ) ;
#16176=AXIS2_PLACEMENT_3D ( 'NONE', #11601, #14633, #22451 ) ;
#16177=CARTESIAN_POINT ( 'NONE',  ( 0.000000000000000000, 17.98401995359670025, -24.59729088254937324 ) ) ;
#16190=LINE ( 'NONE', #3513, #33734 ) ;
#16195=AXIS2_PLACEMENT_3D ( 'NONE', #15058, #25900, #28221 ) ;
#16204=EDGE_CURVE ( 'NONE', #33378, #11423, #15991, .T. ) ;
#16208=CIRCLE ( 'NONE', #15619, 30.47050528711511674 ) ;
#16209=VERTEX_POINT ( 'NONE', #7198 ) ;
#16227=CARTESIAN_POINT ( 'NONE',  ( 0.02407890056441847060, -0.3931553186915530129, 31.08824725498900321 ) ) ;
#16229=CARTESIAN_POINT ( 'NONE',  ( 1.749999999999999778, 34.17636915695680244, 4.045051921974837761 ) ) ;
#16230=AXIS2_PLACEMENT_3D ( 'NONE', #14010, #14373, #25198 ) ;
#16232=DIRECTION ( 'NONE',  ( 0.000000000000000000, 0.000000000000000000, 1.000000000000000000 ) ) ;
#16237=ORIENTED_EDGE ( 'NONE', *, *, #3516, .F. ) ;
#16255=CARTESIAN_POINT ( 'NONE',  ( 0.7561992253044003132, 14.91862693714140242, 30.45773629169372398 ) ) ;
#16260=CARTESIAN_POINT ( 'NONE',  ( 2.261199765031106867, -17.23487904370277235, 28.59786932736725618 ) ) ;
#16264=EDGE_CURVE ( 'NONE', #2759, #3106, #10281, .T. ) ;
#16270=DIRECTION ( 'NONE',  ( -1.000000000000000000, -0.000000000000000000, -0.000000000000000000 ) ) ;
#16276=CIRCLE ( 'NONE', #8891, 30.47050528711512030 ) ;
#16277=ORIENTED_EDGE ( 'NONE', *, *, #22748, .T. ) ;
#16281=EDGE_LOOP ( 'NONE', ( #3302, #18260, #30886, #22233, #29627, #3509, #6583 ) ) ;
#16282=DIRECTION ( 'NONE',  ( 1.000000000000000000, 0.000000000000000000, -0.000000000000000000 ) ) ;
#16283=AXIS2_PLACEMENT_3D ( 'NONE', #32132, #31949, #20936 ) ;
#16295=DIRECTION ( 'NONE',  ( 1.000000000000000000, 0.000000000000000000, 0.000000000000000000 ) ) ;
#16298=DIRECTION ( 'NONE',  ( 0.000000000000000000, 0.000000000000000000, 1.000000000000000000 ) ) ;
#16299=EDGE_CURVE ( 'NONE', #15650, #27137, #53, .T. ) ;
#16301=DIRECTION ( 'NONE',  ( -1.000000000000000000, -0.000000000000000000, -0.000000000000000000 ) ) ;
#16305=CARTESIAN_POINT ( 'NONE',  ( 2.789999999999999591, 0.000000000000000000, 0.000000000000000000 ) ) ;
#16309=CYLINDRICAL_SURFACE ( 'NONE', #32585, 16.19999999999999929 ) ;
#16312=DIRECTION ( 'NONE',  ( 1.000000000000000000, 0.000000000000000000, 0.000000000000000000 ) ) ;
#16335=DIRECTION ( 'NONE',  ( 0.000000000000000000, 0.000000000000000000, 1.000000000000000000 ) ) ;
#16341=CYLINDRICAL_SURFACE ( 'NONE', #12626, 2.524999999999999467 ) ;
#16342=EDGE_CURVE ( 'NONE', #21040, #23180, #34157, .T. ) ;
#16343=EDGE_CURVE ( 'NONE', #31298, #26980, #5743, .T. ) ;
#16346=ORIENTED_EDGE ( 'NONE', *, *, #4669, .F. ) ;
#16354=VECTOR ( 'NONE', #30292, 1000.000000000000000 ) ;
#16361=DIRECTION ( 'NONE',  ( 0.000000000000000000, 0.000000000000000000, 1.000000000000000000 ) ) ;
#16362=FACE_OUTER_BOUND ( 'NONE', #12081, .T. ) ;
#16363=CARTESIAN_POINT ( 'NONE',  ( 1.395000000000002238, 32.09669216789253454, -12.41728656686340138 ) ) ;
#16364=ORIENTED_EDGE ( 'NONE', *, *, #33301, .F. ) ;
#16379=DIRECTION ( 'NONE',  ( -1.000000000000000000, 0.000000000000000000, 0.000000000000000000 ) ) ;
#16380=ORIENTED_EDGE ( 'NONE', *, *, #10497, .T. ) ;
#16385=CARTESIAN_POINT ( 'NONE',  ( 2.789999999999998703, 18.19930456030770927, 24.67628137665903054 ) ) ;
#16386=AXIS2_PLACEMENT_3D ( 'NONE', #34980, #4871, #15770 ) ;
#16389=ORIENTED_EDGE ( 'NONE', *, *, #3451, .F. ) ;
#16394=VERTEX_POINT ( 'NONE', #17536 ) ;
#16396=CARTESIAN_POINT ( 'NONE',  ( 0.000000000000000000, 9.539392014169456147, 3.000000000000000000 ) ) ;
#16401=DIRECTION ( 'NONE',  ( 0.000000000000000000, 0.000000000000000000, 1.000000000000000000 ) ) ;
#16406=CARTESIAN_POINT ( 'NONE',  ( 2.789999999999999147, 14.63235270440936731, 27.43224275967444470 ) ) ;
#16423=CARTESIAN_POINT ( 'NONE',  ( 2.789999999999999147, 7.350529080603541487, 30.20932655202940254 ) ) ;
#16426=ORIENTED_EDGE ( 'NONE', *, *, #8957, .T. ) ;
#16430=DIRECTION ( 'NONE',  ( -1.000000000000000000, -0.000000000000000000, -0.000000000000000000 ) ) ;
#16431=CARTESIAN_POINT ( 'NONE',  ( 2.789999999999999147, 23.53611639059710114, 19.35207786518998319 ) ) ;
#16439=CARTESIAN_POINT ( 'NONE',  ( 0.02407890056655868569, -17.95514392185398833, -25.38201125280375692 ) ) ;
#16441=FACE_OUTER_BOUND ( 'NONE', #14135, .T. ) ;
#16448=EDGE_CURVE ( 'NONE', #1305, #30793, #33146, .T. ) ;
#16455=AXIS2_PLACEMENT_3D ( 'NONE', #7552, #32292, #29285 ) ;
#16460=CARTESIAN_POINT ( 'NONE',  ( 2.783128927722727575, 20.89672672271989029, 22.72123193261248630 ) ) ;
#16464=CARTESIAN_POINT ( 'NONE',  ( 0.000000000000000000, -13.59935610937951900, -28.90010281771846223 ) ) ;
#16476=CARTESIAN_POINT ( 'NONE',  ( 0.02407890056655781832, 18.59128259035472297, 24.91982945642928016 ) ) ;
#16481=ORIENTED_EDGE ( 'NONE', *, *, #14478, .F. ) ;
#16482=B_SPLINE_CURVE_WITH_KNOTS ( 'NONE', 3,
 ( #13872, #24712, #22060, #32900, #8522, #30232 ),
 .UNSPECIFIED., .F., .F.,
 ( 4, 2, 4 ),
 ( 4.404817078215036745E-07, 0.001874269662699934880, 0.003748098843692048571 ),
 .UNSPECIFIED. ) ;
#16486=CARTESIAN_POINT ( 'NONE',  ( 2.231373069951498422, 30.82732872002351598, 13.00174666746740293 ) ) ;
#16487=CARTESIAN_POINT ( 'NONE',  ( 2.789999999999999147, 2.005524111408194088, 31.87689292423238996 ) ) ;
#16490=ORIENTED_EDGE ( 'NONE', *, *, #1313, .F. ) ;
#16491=DIRECTION ( 'NONE',  ( -1.000000000000000000, -0.000000000000000000, -0.000000000000000000 ) ) ;
#16492=CARTESIAN_POINT ( 'NONE',  ( 2.765921099433442443, -30.46391896562403190, -6.211548095912885259 ) ) ;
#16494=EDGE_CURVE ( 'NONE', #19524, #2456, #30324, .T. ) ;
#16499=DIRECTION ( 'NONE',  ( 1.000000000000000000, 0.000000000000000000, 0.000000000000000000 ) ) ;
#16509=ORIENTED_EDGE ( 'NONE', *, *, #30636, .T. ) ;
#16521=CYLINDRICAL_SURFACE ( 'NONE', #671, 16.19999999999999218 ) ;
#16524=DIRECTION ( 'NONE',  ( 0.000000000000000000, 0.000000000000000000, 1.000000000000000000 ) ) ;
#16525=VERTEX_POINT ( 'NONE', #20873 ) ;
#16526=B_SPLINE_CURVE_WITH_KNOTS ( 'NONE', 3,
 ( #33899, #23050, #14702, #25349 ),
 .UNSPECIFIED., .F., .F.,
 ( 4, 4 ),
 ( 2.180635439307156695E-07, 0.0006879539277919046554 ),
 .UNSPECIFIED. ) ;
#16533=CARTESIAN_POINT ( 'NONE',  ( 0.000000000000000000, 17.11426446101236820, -24.44276559937708271 ) ) ;
#16541=CARTESIAN_POINT ( 'NONE',  ( 0.1835381793512137760, -32.24848086092538324, 1.209851624881392862 ) ) ;
#16542=ORIENTED_EDGE ( 'NONE', *, *, #1922, .T. ) ;
#16548=VERTEX_POINT ( 'NONE', #31720 ) ;
#16561=FACE_OUTER_BOUND ( 'NONE', #19934, .T. ) ;
#16565=VERTEX_POINT ( 'NONE', #34048 ) ;
#16566=EDGE_CURVE ( 'NONE', #4415, #14959, #9665, .T. ) ;
#16572=ORIENTED_EDGE ( 'NONE', *, *, #8852, .F. ) ;
#16574=CARTESIAN_POINT ( 'NONE',  ( 2.789999999999999147, -5.984944020945660803, -28.84917528048448787 ) ) ;
#16586=ORIENTED_EDGE ( 'NONE', *, *, #29603, .T. ) ;
#16592=VERTEX_POINT ( 'NONE', #17701 ) ;
#16594=CIRCLE ( 'NONE', #1236, 2.525000000000000799 ) ;
#16599=ORIENTED_EDGE ( 'NONE', *, *, #15558, .T. ) ;
#16606=ORIENTED_EDGE ( 'NONE', *, *, #25287, .F. ) ;
#16609=CARTESIAN_POINT ( 'NONE',  ( 0.000000000000000000, 23.53611639059741378, -19.35207786518964213 ) ) ;
#16611=EDGE_CURVE ( 'NONE', #5255, #13812, #14057, .T. ) ;
#16621=DIRECTION ( 'NONE',  ( 0.000000000000000000, 0.2486898871648417775, 0.9685831611286344067 ) ) ;
#16622=ORIENTED_EDGE ( 'NONE', *, *, #22151, .T. ) ;
#16638=TOROIDAL_SURFACE ( 'NONE', #2967, 30.47050528711512030, 8.000000000000000000 ) ;
#16644=DIRECTION ( 'NONE',  ( -1.000000000000000000, -0.000000000000000000, -0.000000000000000000 ) ) ;
#16656=DIRECTION ( 'NONE',  ( -1.000000000000000000, -0.000000000000000000, -0.000000000000000000 ) ) ;
#16657=DIRECTION ( 'NONE',  ( 0.000000000000000000, 0.000000000000000000, 1.000000000000000000 ) ) ;
#16659=DIRECTION ( 'NONE',  ( -1.000000000000000000, -0.000000000000000000, -0.000000000000000000 ) ) ;
#16661=CYLINDRICAL_SURFACE ( 'NONE', #22244, 34.41491905851385269 ) ;
#16677=CYLINDRICAL_SURFACE ( 'NONE', #10471, 34.41491905851385269 ) ;
#16678=CIRCLE ( 'NONE', #6998, 34.41491905851385269 ) ;
#16682=ORIENTED_EDGE ( 'NONE', *, *, #16095, .F. ) ;
#16687=EDGE_CURVE ( 'NONE', #33582, #30318, #16075, .T. ) ;
#16698=CARTESIAN_POINT ( 'NONE',  ( 0.02407890056655651728, -15.32140196853772984, 27.05343472112986092 ) ) ;
#16700=ORIENTED_EDGE ( 'NONE', *, *, #16299, .F. ) ;
#16708=AXIS2_PLACEMENT_3D ( 'NONE', #8510, #19379, #2460 ) ;
#16709=EDGE_LOOP ( 'NONE', ( #2199, #24718, #26815, #5032, #30475, #1962 ) ) ;
#16720=CARTESIAN_POINT ( 'NONE',  ( 0.7564103395634697025, -9.974843919188980834, -32.41553303492231208 ) ) ;
#16728=CARTESIAN_POINT ( 'NONE',  ( 0.006892404480090298657, -29.45646641511004660, 9.233692607045616896 ) ) ;
#16729=CARTESIAN_POINT ( 'NONE',  ( 0.02407890056655825201, -31.05158812718220673, -1.559667679918931738 ) ) ;
#16734=CARTESIAN_POINT ( 'NONE',  ( 1.040000000000001590, -30.02688531850382958, -16.81585001935613022 ) ) ;
#16737=EDGE_CURVE ( 'NONE', #28601, #23670, #2341, .T. ) ;
#16738=DIRECTION ( 'NONE',  ( 0.000000000000000000, 0.000000000000000000, 1.000000000000000000 ) ) ;
#16739=ORIENTED_EDGE ( 'NONE', *, *, #33758, .T. ) ;
#16740=CARTESIAN_POINT ( 'NONE',  ( 0.02407890056655564992, -30.46391896562403190, -6.211548095912885259 ) ) ;
#16750=LINE ( 'NONE', #11225, #29199 ) ;
#16752=DIRECTION ( 'NONE',  ( -1.000000000000000000, 0.000000000000000000, 0.000000000000000000 ) ) ;
#16755=EDGE_CURVE ( 'NONE', #11863, #4938, #23012, .T. ) ;
#16759=ORIENTED_EDGE ( 'NONE', *, *, #1640, .T. ) ;
#16767=ADVANCED_FACE ( 'NONE', ( #7687 ), #21580, .T. ) ;
#16772=CARTESIAN_POINT ( 'NONE',  ( 2.789999999999998703, 20.82898695786926524, -22.50081875905949147 ) ) ;
#16775=EDGE_CURVE ( 'NONE', #12335, #32759, #26198, .T. ) ;
#16780=VERTEX_POINT ( 'NONE', #34939 ) ;
#16782=CARTESIAN_POINT ( 'NONE',  ( 0.07094832122174615785, 12.21437217961350719, 29.24586132675256422 ) ) ;
#16789=CARTESIAN_POINT ( 'NONE',  ( 50.00050000000000239, 0.000000000000000000, 0.000000000000000000 ) ) ;
#16792=EDGE_LOOP ( 'NONE', ( #26690, #25529, #17454, #18236 ) ) ;
#16794=CARTESIAN_POINT ( 'NONE',  ( 1.749999999999999778, 34.17636915695680244, -4.045051921974834208 ) ) ;
#16802=FACE_OUTER_BOUND ( 'NONE', #34706, .T. ) ;
#16808=B_SPLINE_CURVE_WITH_KNOTS ( 'NONE', 3,
 ( #35056, #32716, #21522, #19039, #5646, #26501 ),
 .UNSPECIFIED., .F., .F.,
 ( 4, 2, 4 ),
 ( 2.120780580244199601E-07, 0.001873410385593401008, 0.003746608693128777694 ),
 .UNSPECIFIED. ) ;
#16809=VERTEX_POINT ( 'NONE', #22108 ) ;
#16818=CARTESIAN_POINT ( 'NONE',  ( 2.789999999999999147, 20.79173593595263014, 22.27454621808771762 ) ) ;
#16825=ORIENTED_EDGE ( 'NONE', *, *, #32441, .F. ) ;
#16833=CARTESIAN_POINT ( 'NONE',  ( 1.394999999999999574, -33.39989884085085947, -8.296590337300607132 ) ) ;
#16836=DIRECTION ( 'NONE',  ( -1.000000000000000000, 0.000000000000000000, 0.000000000000000000 ) ) ;
#16840=CARTESIAN_POINT ( 'NONE',  ( 1.394999999999999574, 6.183021911002327897, -33.85493898757056996 ) ) ;
#16842=FACE_OUTER_BOUND ( 'NONE', #9831, .T. ) ;
#16846=CARTESIAN_POINT ( 'NONE',  ( 1.394999999999999574, 27.68252950111338251, 20.44661865013498669 ) ) ;
#16848=ORIENTED_EDGE ( 'NONE', *, *, #25455, .T. ) ;
#16851=AXIS2_PLACEMENT_3D ( 'NONE', #24023, #2844, #5334 ) ;
#16856=ORIENTED_EDGE ( 'NONE', *, *, #25026, .F. ) ;
#16864=CARTESIAN_POINT ( 'NONE',  ( 2.789999999999999147, 0.000000000000000000, 0.000000000000000000 ) ) ;
#16884=EDGE_LOOP ( 'NONE', ( #23938, #15823, #7669, #8725, #6710, #32406 ) ) ;
#16890=CARTESIAN_POINT ( 'NONE',  ( 2.719051660387896696, 14.74858964725069654, 28.05334937082597335 ) ) ;
#16895=ADVANCED_FACE ( 'NONE', ( #16964 ), #24621, .T. ) ;
#16898=EDGE_CURVE ( 'NONE', #9865, #21866, #31864, .T. ) ;
#16900=CARTESIAN_POINT ( 'NONE',  ( 1.040000000000000924, -10.37741591188871482, -32.81304455236878681 ) ) ;
#16917=CARTESIAN_POINT ( 'NONE',  ( 2.606462089965854378, -28.84240889917340667, 14.47562221546536776 ) ) ;
#16918=ORIENTED_EDGE ( 'NONE', *, *, #6815, .T. ) ;
#16926=ORIENTED_EDGE ( 'NONE', *, *, #8949, .F. ) ;
#16931=AXIS2_PLACEMENT_3D ( 'NONE', #24649, #16499, #30352 ) ;
#16935=EDGE_CURVE ( 'NONE', #14860, #32635, #13294, .T. ) ;
#16947=CARTESIAN_POINT ( 'NONE',  ( 0.02407890056655608360, -31.05158812718222450, 1.559667679918499417 ) ) ;
#16956=FACE_OUTER_BOUND ( 'NONE', #25948, .T. ) ;
#16964=FACE_OUTER_BOUND ( 'NONE', #5951, .T. ) ;
#16972=CARTESIAN_POINT ( 'NONE',  ( 1.749999999999999778, 0.000000000000000000, 0.000000000000000000 ) ) ;
#16984=ORIENTED_EDGE ( 'NONE', *, *, #32787, .F. ) ;
#17012=VERTEX_POINT ( 'NONE', #13676 ) ;
#17025=DIRECTION ( 'NONE',  ( -1.000000000000000000, 0.000000000000000000, 0.000000000000000000 ) ) ;
#17027=EDGE_CURVE ( 'NONE', #4415, #3245, #13846, .T. ) ;
#17031=CARTESIAN_POINT ( 'NONE',  ( 2.790000000000000480, -30.61407293071425428, -1.706449706642680697 ) ) ;
#17044=CARTESIAN_POINT ( 'NONE',  ( 0.5288002497500084997, -32.52406052302386996, 7.554116419246433622 ) ) ;
#17050=CYLINDRICAL_SURFACE ( 'NONE', #30999, 34.41491905851385269 ) ;
#17051=CYLINDRICAL_SURFACE ( 'NONE', #28358, 16.19999999999999574 ) ;
#17052=ORIENTED_EDGE ( 'NONE', *, *, #10468, .T. ) ;
#17058=EDGE_CURVE ( 'NONE', #26512, #14449, #16190, .T. ) ;
#17060=CARTESIAN_POINT ( 'NONE',  ( 0.02407890056655695096, 20.99477179376858871, -22.93149026599722617 ) ) ;
#17061=VERTEX_POINT ( 'NONE', #11726 ) ;
#17069=AXIS2_PLACEMENT_3D ( 'NONE', #27505, #4293, #1636 ) ;
#17083=FACE_OUTER_BOUND ( 'NONE', #18824, .T. ) ;
#17084=FACE_OUTER_BOUND ( 'NONE', #72, .T. ) ;
#17087=DIRECTION ( 'NONE',  ( 0.000000000000000000, 3.606850791634946256E-15, -1.000000000000000000 ) ) ;
#17089=EDGE_CURVE ( 'NONE', #3012, #4601, #3031, .T. ) ;
#17093=CIRCLE ( 'NONE', #32959, 2.524999999999999467 ) ;
#17105=CARTESIAN_POINT ( 'NONE',  ( 1.749999999999999778, 32.09669216789253454, -12.41728656686340138 ) ) ;
#17107=B_SPLINE_CURVE_WITH_KNOTS ( 'NONE', 3,
 ( #3334, #9032, #33050, #6347 ),
 .UNSPECIFIED., .F., .F.,
 ( 4, 4 ),
 ( 0.005298349496164135759, 0.005985218188604201316 ),
 .UNSPECIFIED. ) ;
#17111=VECTOR ( 'NONE', #19486, 1000.000000000000000 ) ;
#17116=B_SPLINE_CURVE_WITH_KNOTS ( 'NONE', 3,
 ( #28159, #9293, #20159, #31007, #6606, #17673 ),
 .UNSPECIFIED., .F., .F.,
 ( 4, 2, 4 ),
 ( 2.570076372265445214E-07, 0.001873455364168430219, 0.003746653720699633615 ),
 .UNSPECIFIED. ) ;
#17119=ORIENTED_EDGE ( 'NONE', *, *, #19494, .F. ) ;
#17130=B_SPLINE_CURVE_WITH_KNOTS ( 'NONE', 3,
 ( #25010, #645, #6141, #27863 ),
 .UNSPECIFIED., .F., .F.,
 ( 4, 4 ),
 ( 0.005298404680630666025, 0.005679541198217082261 ),
 .UNSPECIFIED. ) ;
#17149=CARTESIAN_POINT ( 'NONE',  ( 0.006892398596451419605, -11.06505884892015779, -28.81855237217609655 ) ) ;
#17152=DIRECTION ( 'NONE',  ( -1.000000000000000000, 0.000000000000000000, 0.000000000000000000 ) ) ;
#17167=ORIENTED_EDGE ( 'NONE', *, *, #7733, .T. ) ;
#17173=CARTESIAN_POINT ( 'NONE',  ( 2.719010680456189100, -0.5906890623665679296, -31.68904954958541609 ) ) ;
#17176=DIRECTION ( 'NONE',  ( 0.000000000000000000, 0.000000000000000000, 1.000000000000000000 ) ) ;
#17181=VECTOR ( 'NONE', #19358, 1000.000000000000000 ) ;
#17186=AXIS2_PLACEMENT_3D ( 'NONE', #10116, #20978, #31817 ) ;
#17191=CARTESIAN_POINT ( 'NONE',  ( 0.1835381243669127194, 21.48816195191864153, 24.07669289167355231 ) ) ;
#17193=EDGE_CURVE ( 'NONE', #18581, #21650, #29309, .T. ) ;
#17195=CARTESIAN_POINT ( 'NONE',  ( 8.000000000000000000, 0.000000000000000000, 0.000000000000000000 ) ) ;
#17203=PRODUCT_DEFINITION_SHAPE ( 'NONE', 'NONE',  #31842 ) ;
#17209=AXIS2_PLACEMENT_3D ( 'NONE', #34276, #1706, #26090 ) ;
#17210=AXIS2_PLACEMENT_3D ( 'NONE', #29862, #25024, #19360 ) ;
#17212=CARTESIAN_POINT ( 'NONE',  ( 2.789999999999999147, -29.91351748324099091, -5.799410679710938155 ) ) ;
#17216=EDGE_CURVE ( 'NONE', #10268, #8440, #20794, .T. ) ;
#17219=FACE_OUTER_BOUND ( 'NONE', #13357, .T. ) ;
#17221=VERTEX_POINT ( 'NONE', #9575 ) ;
#17223=DIRECTION ( 'NONE',  ( -1.000000000000000000, -0.000000000000000000, -0.000000000000000000 ) ) ;
#17229=FACE_OUTER_BOUND ( 'NONE', #13957, .T. ) ;
#17233=CARTESIAN_POINT ( 'NONE',  ( 2.789999999999999147, -7.666252171205694133, 29.49034198003803198 ) ) ;
#17235=CARTESIAN_POINT ( 'NONE',  ( 2.789999999999999147, -25.83993731729781729, -18.77381338200996552 ) ) ;
#17243=CARTESIAN_POINT ( 'NONE',  ( 0.000000000000000000, 17.98401995359632011, 24.59729088254965035 ) ) ;
#17248=ORIENTED_EDGE ( 'NONE', *, *, #1651, .T. ) ;
#17250=DIRECTION ( 'NONE',  ( -1.000000000000000000, -0.000000000000000000, -0.000000000000000000 ) ) ;
#17258=CARTESIAN_POINT ( 'NONE',  ( 0.02407890056655695096, -26.45933846664205902, 16.32596387352436551 ) ) ;
#17260=TOROIDAL_SURFACE ( 'NONE', #26318, 30.47050528711512030, 8.000000000000000000 ) ;
#17264=ORIENTED_EDGE ( 'NONE', *, *, #27258, .F. ) ;
#17285=AXIS2_PLACEMENT_3D ( 'NONE', #9154, #6652, #3806 ) ;
#17300=AXIS2_PLACEMENT_3D ( 'NONE', #33247, #9043, #27901 ) ;
#17306=B_SPLINE_CURVE_WITH_KNOTS ( 'NONE', 3,
 ( #20100, #30944, #4399, #1909, #22935, #15289 ),
 .UNSPECIFIED., .F., .F.,
 ( 4, 2, 4 ),
 ( 4.404817051633169802E-07, 0.001874269637237882926, 0.003748098792770602258 ),
 .UNSPECIFIED. ) ;
#17311=VERTEX_POINT ( 'NONE', #26283 ) ;
#17319=FACE_OUTER_BOUND ( 'NONE', #27677, .T. ) ;
#17328=CARTESIAN_POINT ( 'NONE',  ( 0.02407890056655781832, 31.00221527374952046, -2.344426712874310148 ) ) ;
#17329=ORIENTED_EDGE ( 'NONE', *, *, #8407, .T. ) ;
#17335=AXIS2_PLACEMENT_3D ( 'NONE', #4454, #23692, #26173 ) ;
#17337=EDGE_CURVE ( 'NONE', #21866, #30042, #23441, .T. ) ;
#17346=EDGE_CURVE ( 'NONE', #33253, #34878, #6538, .T. ) ;
#17352=ORIENTED_EDGE ( 'NONE', *, *, #14271, .F. ) ;
#17375=DIRECTION ( 'NONE',  ( 0.000000000000000000, 0.000000000000000000, 1.000000000000000000 ) ) ;
#17397=CARTESIAN_POINT ( 'NONE',  ( 0.1859802947979261878, -11.11575656128866463, 30.30758796111447850 ) ) ;
#17408=DIRECTION ( 'NONE',  ( -1.000000000000000000, -0.000000000000000000, 0.000000000000000000 ) ) ;
#17426=EDGE_CURVE ( 'NONE', #16592, #32672, #26812, .T. ) ;
#17431=ORIENTED_EDGE ( 'NONE', *, *, #2174, .T. ) ;
#17436=AXIS2_PLACEMENT_3D ( 'NONE', #31988, #7956, #7597 ) ;
#17437=CARTESIAN_POINT ( 'NONE',  ( 2.789999999999999147, 17.11426446101236820, -24.44276559937708271 ) ) ;
#17442=ORIENTED_EDGE ( 'NONE', *, *, #22146, .T. ) ;
#17443=EDGE_CURVE ( 'NONE', #30046, #23843, #22941, .T. ) ;
#17450=DIRECTION ( 'NONE',  ( -1.000000000000000000, -0.000000000000000000, -0.000000000000000000 ) ) ;
#17452=CARTESIAN_POINT ( 'NONE',  ( 0.1859802683305686877, 19.63342256285821463, 25.62496134208834775 ) ) ;
#17454=ORIENTED_EDGE ( 'NONE', *, *, #17216, .T. ) ;
#17457=DIRECTION ( 'NONE',  ( 0.000000000000000000, 0.000000000000000000, 1.000000000000000000 ) ) ;
#17464=CARTESIAN_POINT ( 'NONE',  ( 1.040000000000000258, -18.66807150955433769, 28.91175816027496381 ) ) ;
#17472=CARTESIAN_POINT ( 'NONE',  ( 1.749999999999999778, -1.891117961019737725, -34.36292081097834483 ) ) ;
#17493=AXIS2_PLACEMENT_3D ( 'NONE', #16864, #32676, #6140 ) ;
#17494=DIRECTION ( 'NONE',  ( 0.000000000000000000, 0.000000000000000000, 1.000000000000000000 ) ) ;
#17497=DIRECTION ( 'NONE',  ( 1.000000000000000000, 0.000000000000000000, 0.000000000000000000 ) ) ;
#17513=CARTESIAN_POINT ( 'NONE',  ( 2.789999999999999147, 7.489092610871091793, 29.53582882395389930 ) ) ;
#17514=FACE_OUTER_BOUND ( 'NONE', #22092, .T. ) ;
#17525=AXIS2_PLACEMENT_3D ( 'NONE', #18692, #32009, #10671 ) ;
#17530=VERTEX_POINT ( 'NONE', #11686 ) ;
#17536=CARTESIAN_POINT ( 'NONE',  ( 1.040000000000000036, 14.40815186467775533, 31.25366880301323746 ) ) ;
#17541=ORIENTED_EDGE ( 'NONE', *, *, #28995, .F. ) ;
#17543=DIRECTION ( 'NONE',  ( -1.000000000000000000, 0.000000000000000000, 0.000000000000000000 ) ) ;
#17574=DIRECTION ( 'NONE',  ( 1.000000000000000000, 0.000000000000000000, 0.000000000000000000 ) ) ;
#17600=DIRECTION ( 'NONE',  ( -1.000000000000000000, 0.000000000000000000, 0.000000000000000000 ) ) ;
#17611=LINE ( 'NONE', #22399, #4569 ) ;
#17626=ORIENTED_EDGE ( 'NONE', *, *, #14778, .T. ) ;
#17630=CARTESIAN_POINT ( 'NONE',  ( 2.790000000000081304, -11.08290750742965436, -28.58973358960031774 ) ) ;
#17634=CIRCLE ( 'NONE', #31251, 34.41491905851385269 ) ;
#17636=ADVANCED_FACE ( 'NONE', ( #3469 ), #16677, .T. ) ;
#17643=VERTEX_POINT ( 'NONE', #11157 ) ;
#17651=EDGE_CURVE ( 'NONE', #9440, #1712, #33520, .T. ) ;
#17658=ORIENTED_EDGE ( 'NONE', *, *, #4200, .T. ) ;
#17673=CARTESIAN_POINT ( 'NONE',  ( 1.040000000000001368, 14.40815186467820652, -31.25366880301302785 ) ) ;
#17683=CARTESIAN_POINT ( 'NONE',  ( 2.789999999999999147, 30.61125888652961891, 5.439165181699118889 ) ) ;
#17684=AXIS2_PLACEMENT_3D ( 'NONE', #7390, #28426, #31266 ) ;
#17695=ORIENTED_EDGE ( 'NONE', *, *, #12271, .F. ) ;
#17701=CARTESIAN_POINT ( 'NONE',  ( 1.749999999999999778, -34.41385771548412720, -0.2702793785573802121 ) ) ;
#17703=AXIS2_PLACEMENT_3D ( 'NONE', #31586, #28919, #4510 ) ;
#17708=CARTESIAN_POINT ( 'NONE',  ( 0.07098933019551863233, -30.32061017160053495, 9.230676164041856424 ) ) ;
#17709=DIRECTION ( 'NONE',  ( -1.000000000000000000, 0.000000000000000000, 0.000000000000000000 ) ) ;
#17712=LINE ( 'NONE', #9677, #25221 ) ;
#17723=EDGE_CURVE ( 'NONE', #797, #17061, #19041, .T. ) ;
#17733=DIRECTION ( 'NONE',  ( -1.000000000000000000, -0.000000000000000000, -0.000000000000000000 ) ) ;
#17737=CARTESIAN_POINT ( 'NONE',  ( 2.765921099433441555, 4.286445725888036407, 30.79383171238946204 ) ) ;
#17741=CARTESIAN_POINT ( 'NONE',  ( 0.02407890056655781832, 7.350529080603967813, -30.20932655202929595 ) ) ;
#17746=LINE ( 'NONE', #23249, #10168 ) ;
#17752=CARTESIAN_POINT ( 'NONE',  ( 2.765921099433443775, -11.07880054387241664, 29.04985141099759360 ) ) ;
#17754=DIRECTION ( 'NONE',  ( -1.000000000000000000, -0.000000000000000000, 0.000000000000000000 ) ) ;
#17758=CARTESIAN_POINT ( 'NONE',  ( 2.789999999999999147, 3.909681563761668421, 30.21863799912384962 ) ) ;
#17759=CARTESIAN_POINT ( 'NONE',  ( 0.000000000000000000, 23.53611639059712601, 19.35207786518996897 ) ) ;
#17764=CARTESIAN_POINT ( 'NONE',  ( 0.006892446353074978965, -30.82736387488653307, 1.618073722873083486 ) ) ;
#17770=ORIENTED_EDGE ( 'NONE', *, *, #11960, .F. ) ;
#17775=FACE_OUTER_BOUND ( 'NONE', #19292, .T. ) ;
#17783=CARTESIAN_POINT ( 'NONE',  ( 0.5248941002295058889, 27.45362965837519909, 18.98707279867261377 ) ) ;
#17789=ADVANCED_FACE ( 'NONE', ( #26235 ), #2527, .T. ) ;
#17792=AXIS2_PLACEMENT_3D ( 'NONE', #12933, #2231, #2061 ) ;
#17803=ADVANCED_BREP_SHAPE_REPRESENTATION ( '', ( #33586, #28566 ), #10954 ) ;
#17804=CARTESIAN_POINT ( 'NONE',  ( 0.006892411738745651655, 7.365885187734036776, 29.97812926094526631 ) ) ;
#17811=AXIS2_PLACEMENT_3D ( 'NONE', #27534, #8846, #5464 ) ;
#17824=LINE ( 'NONE', #20997, #3090 ) ;
#17826=ORIENTED_EDGE ( 'NONE', *, *, #33745, .F. ) ;
#17827=ORIENTED_EDGE ( 'NONE', *, *, #22191, .F. ) ;
#17831=DIRECTION ( 'NONE',  ( -1.000000000000000000, 0.000000000000000000, 0.000000000000000000 ) ) ;
#17836=CIRCLE ( 'NONE', #1336, 2.525000000000000799 ) ;
#17843=CARTESIAN_POINT ( 'NONE',  ( 2.783107600408745164, -7.987299431473431355, -29.81857704081753369 ) ) ;
#17850=EDGE_CURVE ( 'NONE', #1771, #21781, #26407, .T. ) ;
#17853=EDGE_CURVE ( 'NONE', #33874, #33898, #26267, .T. ) ;
#17859=CARTESIAN_POINT ( 'NONE',  ( -8.346024214154725512E-14, 18.20059223136345139, 24.67675383855258175 ) ) ;
#17861=VERTEX_POINT ( 'NONE', #31749 ) ;
#17880=CARTESIAN_POINT ( 'NONE',  ( -5.210000000000000853, 0.000000000000000000, 0.000000000000000000 ) ) ;
#17883=B_SPLINE_CURVE_WITH_KNOTS ( 'NONE', 3,
 ( #34056, #17708, #20201, #9144, #15031, #28717 ),
 .UNSPECIFIED., .F., .F.,
 ( 4, 2, 4 ),
 ( 1.974571759321709208E-07, 0.001873395748763636952, 0.003746594040351341418 ),
 .UNSPECIFIED. ) ;
#17890=CARTESIAN_POINT ( 'NONE',  ( 1.749999999999999778, -33.39989884085085237, -8.296590337300626672 ) ) ;
#17902=EDGE_CURVE ( 'NONE', #4330, #2635, #32447, .T. ) ;
#17911=DIRECTION ( 'NONE',  ( 1.000000000000000000, 0.000000000000000000, 0.000000000000000000 ) ) ;
#17922=CARTESIAN_POINT ( 'NONE',  ( 0.07094834059292320916, 7.308651292220183393, -30.83982692225020017 ) ) ;
#17930=CARTESIAN_POINT ( 'NONE',  ( 8.000000000000000000, 0.000000000000000000, 0.000000000000000000 ) ) ;
#17947=B_SPLINE_CURVE_WITH_KNOTS ( 'NONE', 3,
 ( #10564, #32603, #24415, #15739 ),
 .UNSPECIFIED., .F., .F.,
 ( 4, 4 ),
 ( 2.335573237707780769E-07, 0.0006879695513619300427 ),
 .UNSPECIFIED. ) ;
#17952=CARTESIAN_POINT ( 'NONE',  ( 2.783128873642846113, -15.15173253686525001, 26.89521541643887304 ) ) ;
#17968=VECTOR ( 'NONE', #32075, 1000.000000000000000 ) ;
#17980=CARTESIAN_POINT ( 'NONE',  ( 2.033800785574606085, -25.08322906883849512, 22.82697412903067757 ) ) ;
#17988=CARTESIAN_POINT ( 'NONE',  ( 0.02407890056655738464, -11.07880054387241664, 29.04985141099759360 ) ) ;
#17990=EDGE_CURVE ( 'NONE', #5282, #26863, #11287, .T. ) ;
#17991=ORIENTED_EDGE ( 'NONE', *, *, #28078, .F. ) ;
#17998=CARTESIAN_POINT ( 'NONE',  ( 2.789999999999999147, 20.79173593595263014, 22.27454621808771762 ) ) ;
#18000=CARTESIAN_POINT ( 'NONE',  ( 0.02407890056655608360, -27.96208973699893008, -13.59246946040217630 ) ) ;
#18006=DIRECTION ( 'NONE',  ( 1.000000000000000000, -0.000000000000000000, -0.000000000000000000 ) ) ;
#18008=ORIENTED_EDGE ( 'NONE', *, *, #33673, .T. ) ;
#18011=ORIENTED_EDGE ( 'NONE', *, *, #32890, .F. ) ;
#18013=CARTESIAN_POINT ( 'NONE',  ( 2.604019731669432680, 19.63342256285856990, -25.62496134208807064 ) ) ;
#18015=ORIENTED_EDGE ( 'NONE', *, *, #33722, .F. ) ;
#18018=DIRECTION ( 'NONE',  ( 0.000000000000000000, 0.000000000000000000, 1.000000000000000000 ) ) ;
#18023=CARTESIAN_POINT ( 'NONE',  ( 2.789819856565905809, -25.83993731729781373, -16.24881338200996694 ) ) ;
#18026=FACE_OUTER_BOUND ( 'NONE', #5829, .T. ) ;
#18028=EDGE_CURVE ( 'NONE', #11449, #7721, #19654, .T. ) ;
#18030=CIRCLE ( 'NONE', #5487, 2.524999999999999467 ) ;
#18033=VERTEX_POINT ( 'NONE', #11110 ) ;
#18038=EDGE_CURVE ( 'NONE', #9316, #9953, #32624, .T. ) ;
#18039=DIRECTION ( 'NONE',  ( 0.000000000000000000, 0.000000000000000000, 1.000000000000000000 ) ) ;
#18040=ORIENTED_EDGE ( 'NONE', *, *, #23622, .T. ) ;
#18046=ORIENTED_EDGE ( 'NONE', *, *, #17346, .F. ) ;
#18047=CARTESIAN_POINT ( 'NONE',  ( 1.040000000000000924, 0.000000000000000000, 0.000000000000000000 ) ) ;
#18048=DIRECTION ( 'NONE',  ( -1.000000000000000000, -0.000000000000000000, -0.000000000000000000 ) ) ;
#18062=DIRECTION ( 'NONE',  ( -1.000000000000000000, 0.000000000000000000, 0.000000000000000000 ) ) ;
#18067=AXIS2_PLACEMENT_3D ( 'NONE', #14007, #28050, #25015 ) ;
#18074=CARTESIAN_POINT ( 'NONE',  ( 0.000000000000000000, 29.94779062842788164, 5.619744560739158068 ) ) ;
#18085=ORIENTED_EDGE ( 'NONE', *, *, #17850, .T. ) ;
#18086=DIRECTION ( 'NONE',  ( -1.000000000000000000, -0.000000000000000000, -0.000000000000000000 ) ) ;
#18091=CIRCLE ( 'NONE', #26591, 2.525000000000001243 ) ;
#18095=ORIENTED_EDGE ( 'NONE', *, *, #18916, .T. ) ;
#18096=CARTESIAN_POINT ( 'NONE',  ( 0.1859802947476339452, 7.229557500019326177, -31.46177729073534124 ) ) ;
#18105=ADVANCED_FACE ( 'NONE', ( #3783 ), #1641, .T. ) ;
#18107=CARTESIAN_POINT ( 'NONE',  ( 0.006892381172647100117, -21.36453267519092591, 22.28230728413997852 ) ) ;
#18110=EDGE_CURVE ( 'NONE', #20352, #32641, #12791, .T. ) ;
#18112=CARTESIAN_POINT ( 'NONE',  ( 50.00050000000000239, 1.224646799147353256E-15, -10.00000000000000000 ) ) ;
#18122=ORIENTED_EDGE ( 'NONE', *, *, #3213, .T. ) ;
#18128=VECTOR ( 'NONE', #21396, 1000.000000000000000 ) ;
#18136=CYLINDRICAL_SURFACE ( 'NONE', #31295, 16.19999999999999574 ) ;
#18138=ORIENTED_EDGE ( 'NONE', *, *, #27179, .T. ) ;
#18139=ORIENTED_EDGE ( 'NONE', *, *, #6752, .F. ) ;
#18151=ORIENTED_EDGE ( 'NONE', *, *, #29038, .T. ) ;
#18168=EDGE_LOOP ( 'NONE', ( #35022, #33508, #400, #27642, #7784, #30570 ) ) ;
#18173=EDGE_LOOP ( 'NONE', ( #5039, #26554, #33341, #22378 ) ) ;
#18177=CARTESIAN_POINT ( 'NONE',  ( 2.719010684783665699, 24.79335165344823366, 19.74422662903628023 ) ) ;
#18192=CARTESIAN_POINT ( 'NONE',  ( 2.789999999999999147, 30.27116788629744804, 13.00174666746673147 ) ) ;
#18197=CARTESIAN_POINT ( 'NONE',  ( 0.02407890056655695096, 26.03801215795542134, -16.98986790278583570 ) ) ;
#18198=CARTESIAN_POINT ( 'NONE',  ( 0.1835380586958561544, -8.814691041839493479, 31.04399216667567529 ) ) ;
#18200=ORIENTED_EDGE ( 'NONE', *, *, #13428, .F. ) ;
#18208=VERTEX_POINT ( 'NONE', #28357 ) ;
#18210=FACE_OUTER_BOUND ( 'NONE', #29371, .T. ) ;
#18212=EDGE_LOOP ( 'NONE', ( #30673, #26263, #25820, #6818 ) ) ;
#18220=CARTESIAN_POINT ( 'NONE',  ( 2.789999999999999147, 0.000000000000000000, 0.000000000000000000 ) ) ;
#18232=ADVANCED_FACE ( 'NONE', ( #18210 ), #21568, .T. ) ;
#18235=CARTESIAN_POINT ( 'NONE',  ( 1.749999999999999778, 0.000000000000000000, 0.000000000000000000 ) ) ;
#18236=ORIENTED_EDGE ( 'NONE', *, *, #15465, .F. ) ;
#18240=ORIENTED_EDGE ( 'NONE', *, *, #22146, .F. ) ;
#18242=DIRECTION ( 'NONE',  ( 1.000000000000000000, 0.000000000000000000, 0.000000000000000000 ) ) ;
#18246=VERTEX_POINT ( 'NONE', #12867 ) ;
#18252=ORIENTED_EDGE ( 'NONE', *, *, #1127, .T. ) ;
#18254=DIRECTION ( 'NONE',  ( -1.000000000000000000, 0.000000000000000000, -0.000000000000000000 ) ) ;
#18259=DIRECTION ( 'NONE',  ( 0.000000000000000000, 0.000000000000000000, 1.000000000000000000 ) ) ;
#18260=ORIENTED_EDGE ( 'NONE', *, *, #10923, .F. ) ;
#18262=DIRECTION ( 'NONE',  ( -1.000000000000000000, 0.000000000000000000, -0.000000000000000000 ) ) ;
#18265=EDGE_CURVE ( 'NONE', #2234, #28134, #7596, .T. ) ;
#18271=CARTESIAN_POINT ( 'NONE',  ( 2.789999999999999147, -16.83127206196758152, 25.36297913013168426 ) ) ;
#18298=CARTESIAN_POINT ( 'NONE',  ( 2.789999999999999147, -14.75935258146392570, -26.65732927035534772 ) ) ;
#18308=DIRECTION ( 'NONE',  ( -1.000000000000000000, -0.000000000000000000, -0.000000000000000000 ) ) ;
#18318=CARTESIAN_POINT ( 'NONE',  ( 0.02407890056655695096, 26.03801215795542134, -16.98986790278583570 ) ) ;
#18321=ORIENTED_EDGE ( 'NONE', *, *, #30261, .T. ) ;
#18323=VECTOR ( 'NONE', #20253, 1000.000000000000000 ) ;
#18327=CARTESIAN_POINT ( 'NONE',  ( 2.033589660297129065, -25.08336923281130026, -22.82737131378450357 ) ) ;
#18330=CARTESIAN_POINT ( 'NONE',  ( 2.789999999999999147, -29.69698570178010755, -11.75786841620047163 ) ) ;
#18341=CARTESIAN_POINT ( 'NONE',  ( 2.783107595519907829, -29.45646641510990804, -9.233692607046043221 ) ) ;
#18367=AXIS2_PLACEMENT_3D ( 'NONE', #11275, #583, #3416 ) ;
#18374=ADVANCED_FACE ( 'NONE', ( #13561 ), #27075, .F. ) ;
#18378=ORIENTED_EDGE ( 'NONE', *, *, #33134, .T. ) ;
#18385=FACE_OUTER_BOUND ( 'NONE', #9488, .T. ) ;
#18395=DIRECTION ( 'NONE',  ( -1.000000000000000000, -0.000000000000000000, -0.000000000000000000 ) ) ;
#18398=VERTEX_POINT ( 'NONE', #5522 ) ;
#18404=CARTESIAN_POINT ( 'NONE',  ( 2.719010716928600857, 19.10423307544339622, 25.28978101402055145 ) ) ;
#18434=DIRECTION ( 'NONE',  ( -1.000000000000000000, 0.000000000000000000, 0.000000000000000000 ) ) ;
#18435=CARTESIAN_POINT ( 'NONE',  ( 0.000000000000000000, -29.91351748324100512, -5.799410679710955030 ) ) ;
#18440=VERTEX_POINT ( 'NONE', #30457 ) ;
#18449=DIRECTION ( 'NONE',  ( 1.000000000000000000, 0.000000000000000000, 0.000000000000000000 ) ) ;
#18452=LINE ( 'NONE', #18112, #3553 ) ;
#18459=EDGE_CURVE ( 'NONE', #32641, #21769, #25293, .T. ) ;
#18468=CARTESIAN_POINT ( 'NONE',  ( 2.013160256205026144, 31.37535259441678903, 12.97259700501048840 ) ) ;
#18473=AXIS2_PLACEMENT_3D ( 'NONE', #29773, #16270, #8414 ) ;
#18480=CARTESIAN_POINT ( 'NONE',  ( 0.000000000000000000, -5.984944020945660803, -31.37417528048448645 ) ) ;
#18488=EDGE_CURVE ( 'NONE', #31361, #16565, #24995, .T. ) ;
#18525=DIRECTION ( 'NONE',  ( -1.000000000000000000, 0.000000000000000000, 0.000000000000000000 ) ) ;
#18530=DIRECTION ( 'NONE',  ( 1.000000000000000000, -0.000000000000000000, -0.000000000000000000 ) ) ;
#18538=CARTESIAN_POINT ( 'NONE',  ( 2.789999999999999147, -20.35927063852789232, -24.61013060777193218 ) ) ;
#18539=CARTESIAN_POINT ( 'NONE',  ( 2.789999999999999147, -5.984944020945660803, -31.37417528048448645 ) ) ;
#18550=CARTESIAN_POINT ( 'NONE',  ( 2.033589656297370318, -29.46130761496106842, 16.80165608683625678 ) ) ;
#18556=CARTESIAN_POINT ( 'NONE',  ( 0.000000000000000000, 17.11426446101236820, -26.96776559937708129 ) ) ;
#18563=CARTESIAN_POINT ( 'NONE',  ( 8.000000000000000000, 0.000000000000000000, 0.000000000000000000 ) ) ;
#18567=CARTESIAN_POINT ( 'NONE',  ( 0.006892381754031734996, 20.89684813776007388, 22.72149230800640751 ) ) ;
#18573=ORIENTED_EDGE ( 'NONE', *, *, #29386, .T. ) ;
#18574=ORIENTED_EDGE ( 'NONE', *, *, #19067, .F. ) ;
#18577=AXIS2_PLACEMENT_3D ( 'NONE', #27669, #625, #11486 ) ;
#18581=VERTEX_POINT ( 'NONE', #28484 ) ;
#18582=ADVANCED_FACE ( 'NONE', ( #30984 ), #27003, .T. ) ;
#18600=VERTEX_POINT ( 'NONE', #28316 ) ;
#18601=ORIENTED_EDGE ( 'NONE', *, *, #19901, .T. ) ;
#18608=ORIENTED_EDGE ( 'NONE', *, *, #17216, .F. ) ;
#18614=CARTESIAN_POINT ( 'NONE',  ( 0.000000000000000000, 0.000000000000000000, 0.000000000000000000 ) ) ;
#18616=ORIENTED_EDGE ( 'NONE', *, *, #13711, .F. ) ;
#18635=AXIS2_PLACEMENT_3D ( 'NONE', #17880, #15198, #1656 ) ;
#18641=AXIS2_PLACEMENT_3D ( 'NONE', #5970, #11166, #8829 ) ;
#18645=VERTEX_POINT ( 'NONE', #33996 ) ;
#18648=AXIS2_PLACEMENT_3D ( 'NONE', #14495, #25856, #33342 ) ;
#18650=CARTESIAN_POINT ( 'NONE',  ( 2.789999999999999147, -30.46391896562403190, -6.211548095912885259 ) ) ;
#18666=FACE_OUTER_BOUND ( 'NONE', #5245, .T. ) ;
#18670=CARTESIAN_POINT ( 'NONE',  ( 2.033589655658247342, 31.33480229261830630, -12.97668906163614189 ) ) ;
#18686=B_SPLINE_CURVE_WITH_KNOTS ( 'NONE', 3,
 ( #2154, #15704, #13028, #34726 ),
 .UNSPECIFIED., .F., .F.,
 ( 4, 4 ),
 ( 2.436748180515292673E-07, 0.0006879797535939334791 ),
 .UNSPECIFIED. ) ;
#18687=ORIENTED_EDGE ( 'NONE', *, *, #24378, .F. ) ;
#18692=CARTESIAN_POINT ( 'NONE',  ( 2.789999999999999147, -26.36977540154997257, -15.20550475489965514 ) ) ;
#18700=FACE_OUTER_BOUND ( 'NONE', #18955, .T. ) ;
#18705=EDGE_LOOP ( 'NONE', ( #27855, #33726, #15520, #21444, #13279, #18095 ) ) ;
#18707=EDGE_CURVE ( 'NONE', #31215, #2635, #25316, .T. ) ;
#18718=CYLINDRICAL_SURFACE ( 'NONE', #31459, 16.19999999999999574 ) ;
#18735=CARTESIAN_POINT ( 'NONE',  ( 0.000000000000000000, 27.98916443103598439, 15.38717335695048227 ) ) ;
#18739=B_SPLINE_CURVE_WITH_KNOTS ( 'NONE', 3,
 ( #21983, #13979, #8617, #8092, #19496, #19151 ),
 .UNSPECIFIED., .F., .F.,
 ( 4, 2, 4 ),
 ( 1.978909662040563688E-07, 0.001873396183027086154, 0.003746594475087968324 ),
 .UNSPECIFIED. ) ;
#18747=B_SPLINE_CURVE_WITH_KNOTS ( 'NONE', 3,
 ( #10918, #24594, #27277, #7887, #2886, #32612 ),
 .UNSPECIFIED., .F., .F.,
 ( 4, 2, 4 ),
 ( 2.040444213406099367E-07, 0.001873402343194270235, 0.003746600641967199555 ),
 .UNSPECIFIED. ) ;
#18749=DIRECTION ( 'NONE',  ( 0.000000000000000000, 0.000000000000000000, 1.000000000000000000 ) ) ;
#18751=DIRECTION ( 'NONE',  ( -1.000000000000000000, 0.000000000000000000, 0.000000000000000000 ) ) ;
#18754=CARTESIAN_POINT ( 'NONE',  ( 0.02407890056441847060, -0.3931553186915530129, 31.08824725498900321 ) ) ;
#18763=CARTESIAN_POINT ( 'NONE',  ( 0.006871052634921217921, 28.06661910905163992, 12.85272128629691579 ) ) ;
#18765=CARTESIAN_POINT ( 'NONE',  ( 0.02407890056655564992, -30.46391896562411716, 6.211548095912460710 ) ) ;
#18771=ADVANCED_FACE ( 'NONE', ( #2427 ), #26646, .T. ) ;
#18773=ORIENTED_EDGE ( 'NONE', *, *, #6509, .F. ) ;
#18776=ORIENTED_EDGE ( 'NONE', *, *, #32605, .F. ) ;
#18778=LINE ( 'NONE', #20907, #30483 ) ;
#18781=ORIENTED_EDGE ( 'NONE', *, *, #18971, .T. ) ;
#18782=DIRECTION ( 'NONE',  ( 0.000000000000000000, 0.000000000000000000, 1.000000000000000000 ) ) ;
#18787=CIRCLE ( 'NONE', #24441, 2.525000000000001243 ) ;
#18792=CARTESIAN_POINT ( 'NONE',  ( 1.749999999999999778, 31.89769921723006263, -12.91988538846924151 ) ) ;
#18793=DIRECTION ( 'NONE',  ( 0.000000000000000000, 0.000000000000000000, 1.000000000000000000 ) ) ;
#18800=CARTESIAN_POINT ( 'NONE',  ( 0.000000000000000000, 25.67797970382135375, 16.40405592474768426 ) ) ;
#18801=CARTESIAN_POINT ( 'NONE',  ( 0.7564103417896115289, 22.02455111472467308, -25.79115045147355190 ) ) ;
#18824=EDGE_LOOP ( 'NONE', ( #13525, #12578, #22767, #34481 ) ) ;
#18829=DIRECTION ( 'NONE',  ( -1.000000000000000000, -0.000000000000000000, -0.000000000000000000 ) ) ;
#18830=CARTESIAN_POINT ( 'NONE',  ( 2.789999999999999147, -13.59935610937951900, -28.90010281771846223 ) ) ;
#18833=ORIENTED_EDGE ( 'NONE', *, *, #24407, .F. ) ;
#18834=CARTESIAN_POINT ( 'NONE',  ( 0.1835380226106660129, 19.62374805819769819, -25.61906966869672075 ) ) ;
#18835=CARTESIAN_POINT ( 'NONE',  ( 2.765921099433441999, 4.286445725888479608, -30.79383171238939809 ) ) ;
#18836=AXIS2_PLACEMENT_3D ( 'NONE', #13432, #18953, #5566 ) ;
#18837=CARTESIAN_POINT ( 'NONE',  ( 2.604019705859993206, 29.54981872718654046, -12.99685134853830348 ) ) ;
#18871=ORIENTED_EDGE ( 'NONE', *, *, #28415, .T. ) ;
#18873=CARTESIAN_POINT ( 'NONE',  ( 2.789999999999999147, -9.994970281559119485, -28.75192165143428724 ) ) ;
#18876=AXIS2_PLACEMENT_3D ( 'NONE', #20011, #14326, #27005 ) ;
#18887=FACE_OUTER_BOUND ( 'NONE', #13574, .T. ) ;
#18890=B_SPLINE_CURVE_WITH_KNOTS ( 'NONE', 3,
 ( #20654, #31499, #15681, #31837, #7452, #15324 ),
 .UNSPECIFIED., .F., .F.,
 ( 4, 2, 4 ),
 ( 2.011514595390488525E-07, 0.001873399447076933835, 0.003746597742694328728 ),
 .UNSPECIFIED. ) ;
#18891=DIRECTION ( 'NONE',  ( -1.000000000000000000, 0.000000000000000000, -0.000000000000000000 ) ) ;
#18892=DIRECTION ( 'NONE',  ( -1.000000000000000000, 0.000000000000000000, 0.000000000000000000 ) ) ;
#18898=EDGE_CURVE ( 'NONE', #1364, #26980, #31786, .T. ) ;
#18902=EDGE_CURVE ( 'NONE', #16548, #7253, #26684, .T. ) ;
#18911=EDGE_LOOP ( 'NONE', ( #15948, #12005, #23518, #20064 ) ) ;
#18916=EDGE_CURVE ( 'NONE', #16525, #22746, #15691, .T. ) ;
#18917=DIRECTION ( 'NONE',  ( -1.000000000000000000, -0.000000000000000000, -0.000000000000000000 ) ) ;
#18920=CARTESIAN_POINT ( 'NONE',  ( 2.261199740790834412, -32.14027485980090404, 9.048862969375786491 ) ) ;
#18925=FACE_OUTER_BOUND ( 'NONE', #32515, .T. ) ;
#18926=LINE ( 'NONE', #21588, #6434 ) ;
#18932=CARTESIAN_POINT ( 'NONE',  ( 2.789999999999999147, 30.93646776788807173, -7.943134866715984899 ) ) ;
#18937=VERTEX_POINT ( 'NONE', #3133 ) ;
#18948=ORIENTED_EDGE ( 'NONE', *, *, #33578, .T. ) ;
#18953=DIRECTION ( 'NONE',  ( -1.000000000000000000, 0.000000000000000000, 0.000000000000000000 ) ) ;
#18955=EDGE_LOOP ( 'NONE', ( #29836, #20785, #23954, #12504, #17248, #11468 ) ) ;
#18966=LINE ( 'NONE', #16840, #33713 ) ;
#18969=DIRECTION ( 'NONE',  ( 0.000000000000000000, 0.000000000000000000, -1.000000000000000000 ) ) ;
#18971=EDGE_CURVE ( 'NONE', #6373, #23746, #34995, .T. ) ;
#18981=VERTEX_POINT ( 'NONE', #25907 ) ;
#18982=CARTESIAN_POINT ( 'NONE',  ( 2.783128920429635667, -21.36428053051117715, 22.28216981039778233 ) ) ;
#18983=EDGE_CURVE ( 'NONE', #33898, #11797, #7364, .T. ) ;
#18996=CARTESIAN_POINT ( 'NONE',  ( 2.809983787309732928E-16, -17.84464379609624984, -24.93395722650028290 ) ) ;
#19000=VECTOR ( 'NONE', #27018, 1000.000000000000000 ) ;
#19004=EDGE_CURVE ( 'NONE', #26512, #25584, #20231, .T. ) ;
#19016=EDGE_CURVE ( 'NONE', #34043, #19094, #29649, .T. ) ;
#19020=VECTOR ( 'NONE', #28956, 1000.000000000000000 ) ;
#19026=EDGE_CURVE ( 'NONE', #27727, #28601, #2082, .T. ) ;
#19032=CARTESIAN_POINT ( 'NONE',  ( 2.765921099433442887, -26.45933846664205902, 16.32596387352436551 ) ) ;
#19035=ORIENTED_EDGE ( 'NONE', *, *, #31496, .T. ) ;
#19039=CARTESIAN_POINT ( 'NONE',  ( 0.5248942303300246914, 26.54141775410178283, -20.24262527922973831 ) ) ;
#19041=CIRCLE ( 'NONE', #16195, 34.41491905851385269 ) ;
#19047=DIRECTION ( 'NONE',  ( 1.000000000000000000, 0.000000000000000000, 0.000000000000000000 ) ) ;
#19049=ORIENTED_EDGE ( 'NONE', *, *, #762, .T. ) ;
#19050=DIRECTION ( 'NONE',  ( 0.000000000000000000, 0.4817536741017036106, 0.8763066800438700232 ) ) ;
#19056=DIRECTION ( 'NONE',  ( -1.000000000000000000, -0.000000000000000000, 0.000000000000000000 ) ) ;
#19062=ORIENTED_EDGE ( 'NONE', *, *, #28567, .F. ) ;
#19067=EDGE_CURVE ( 'NONE', #24998, #916, #33277, .T. ) ;
#19070=DIRECTION ( 'NONE',  ( 0.000000000000000000, 0.1253332335643122519, -0.9921147013144767657 ) ) ;
#19075=DIRECTION ( 'NONE',  ( 0.000000000000000000, 0.000000000000000000, 1.000000000000000000 ) ) ;
#19079=VERTEX_POINT ( 'NONE', #12227 ) ;
#19081=AXIS2_PLACEMENT_3D ( 'NONE', #28776, #4716, #26451 ) ;
#19083=AXIS2_PLACEMENT_3D ( 'NONE', #10046, #15937, #12729 ) ;
#19089=CARTESIAN_POINT ( 'NONE',  ( 2.765921099433442443, 20.99477179376858871, -22.93149026599722617 ) ) ;
#19094=VERTEX_POINT ( 'NONE', #32111 ) ;
#19114=EDGE_CURVE ( 'NONE', #13159, #12420, #23684, .T. ) ;
#19125=EDGE_LOOP ( 'NONE', ( #1852, #24705, #6627, #20518 ) ) ;
#19139=DIRECTION ( 'NONE',  ( -1.000000000000000000, -0.000000000000000000, 0.000000000000000000 ) ) ;
#19151=CARTESIAN_POINT ( 'NONE',  ( 1.749999999999999778, 6.714005886385429278, -33.75364837705166110 ) ) ;
#19156=ORIENTED_EDGE ( 'NONE', *, *, #21975, .F. ) ;
#19157=CARTESIAN_POINT ( 'NONE',  ( 0.02407890056655738464, 26.03801215795517621, 16.98986790278620873 ) ) ;
#19162=CARTESIAN_POINT ( 'NONE',  ( 2.765921099433443331, 26.03801215795517621, 16.98986790278620873 ) ) ;
#19165=EDGE_CURVE ( 'NONE', #693, #23520, #24435, .T. ) ;
#19166=AXIS2_PLACEMENT_3D ( 'NONE', #22411, #13877, #30421 ) ;
#19167=ORIENTED_EDGE ( 'NONE', *, *, #28406, .T. ) ;
#19173=ADVANCED_FACE ( 'NONE', ( #29797 ), #29277, .T. ) ;
#19185=CARTESIAN_POINT ( 'NONE',  ( 1.040000000000000924, 0.000000000000000000, 0.000000000000000000 ) ) ;
#19191=CARTESIAN_POINT ( 'NONE',  ( 2.789999999999999147, -21.75986515490491868, 21.28569233123086946 ) ) ;
#19217=CARTESIAN_POINT ( 'NONE',  ( 2.265105736152236204, 14.91070698422201346, -29.86438609618728890 ) ) ;
#19221=VERTEX_POINT ( 'NONE', #6271 ) ;
#19224=FACE_OUTER_BOUND ( 'NONE', #23062, .T. ) ;
#19229=CARTESIAN_POINT ( 'NONE',  ( 1.749999999999999778, 34.17636915695680244, -4.045051921974834208 ) ) ;
#19236=CIRCLE ( 'NONE', #21480, 34.41491905851385269 ) ;
#19237=CARTESIAN_POINT ( 'NONE',  ( 2.790000000000000036, 29.09243261715505469, -9.683176917503056202 ) ) ;
#19249=ORIENTED_EDGE ( 'NONE', *, *, #24948, .T. ) ;
#19267=DIRECTION ( 'NONE',  ( 0.000000000000000000, 0.000000000000000000, 1.000000000000000000 ) ) ;
#19272=CARTESIAN_POINT ( 'NONE',  ( 0.1859802604725803721, 12.64393372169665675, 29.70253967906869974 ) ) ;
#19283=DIRECTION ( 'NONE',  ( 0.000000000000000000, 0.000000000000000000, 1.000000000000000000 ) ) ;
#19285=CARTESIAN_POINT ( 'NONE',  ( 2.789999999999999147, 25.67797970382158113, -16.40405592474728635 ) ) ;
#19292=EDGE_LOOP ( 'NONE', ( #1412, #1540, #4303, #30971, #28542, #22154 ) ) ;
#19296=DIRECTION ( 'NONE',  ( 0.000000000000000000, 0.000000000000000000, 1.000000000000000000 ) ) ;
#19306=ORIENTED_EDGE ( 'NONE', *, *, #31267, .T. ) ;
#19324=ORIENTED_EDGE ( 'NONE', *, *, #15719, .T. ) ;
#19326=CARTESIAN_POINT ( 'NONE',  ( 0.07094833404649768249, 21.26181984063927999, -23.50417665061993944 ) ) ;
#19327=FACE_OUTER_BOUND ( 'NONE', #19916, .T. ) ;
#19333=ORIENTED_EDGE ( 'NONE', *, *, #33292, .F. ) ;
#19342=CYLINDRICAL_SURFACE ( 'NONE', #24954, 16.19999999999999574 ) ;
#19357=DIRECTION ( 'NONE',  ( -1.000000000000000000, 0.000000000000000000, -0.000000000000000000 ) ) ;
#19358=DIRECTION ( 'NONE',  ( -1.000000000000000000, 0.000000000000000000, -0.000000000000000000 ) ) ;
#19360=DIRECTION ( 'NONE',  ( 0.000000000000000000, 0.000000000000000000, 1.000000000000000000 ) ) ;
#19362=DIRECTION ( 'NONE',  ( -1.000000000000000000, -0.000000000000000000, -0.000000000000000000 ) ) ;
#19376=AXIS2_PLACEMENT_3D ( 'NONE', #18830, #965, #11652 ) ;
#19378=TOROIDAL_SURFACE ( 'NONE', #17684, 30.47050528711512030, 8.000000000000000000 ) ;
#19379=DIRECTION ( 'NONE',  ( -1.000000000000000000, -0.000000000000000000, -0.000000000000000000 ) ) ;
#19380=ORIENTED_EDGE ( 'NONE', *, *, #23923, .T. ) ;
#19398=DIRECTION ( 'NONE',  ( 0.000000000000000000, 0.000000000000000000, 1.000000000000000000 ) ) ;
#19405=AXIS2_PLACEMENT_3D ( 'NONE', #818, #8528, #16738 ) ;
#19409=DIRECTION ( 'NONE',  ( -1.000000000000000000, -0.000000000000000000, -0.000000000000000000 ) ) ;
#19416=CYLINDRICAL_SURFACE ( 'NONE', #24716, 16.19999999999999574 ) ;
#19421=VERTEX_POINT ( 'NONE', #31373 ) ;
#19436=CARTESIAN_POINT ( 'NONE',  ( 2.033800776873903704, -18.61835568386960915, 28.34776818504836626 ) ) ;
#19437=CARTESIAN_POINT ( 'NONE',  ( 2.789999999999999147, -8.813854705727671046, 29.13568936554939981 ) ) ;
#19442=CARTESIAN_POINT ( 'NONE',  ( 1.749999999999999778, 0.000000000000000000, 0.000000000000000000 ) ) ;
#19457=DIRECTION ( 'NONE',  ( 0.000000000000000000, 0.000000000000000000, 1.000000000000000000 ) ) ;
#19472=CARTESIAN_POINT ( 'NONE',  ( 1.394999999999999574, 21.72796464722046039, -26.68861566460872936 ) ) ;
#19477=VECTOR ( 'NONE', #10778, 1000.000000000000000 ) ;
#19486=DIRECTION ( 'NONE',  ( -1.000000000000000000, 0.000000000000000000, 0.000000000000000000 ) ) ;
#19488=DIRECTION ( 'NONE',  ( -1.000000000000000000, 0.000000000000000000, 0.000000000000000000 ) ) ;
#19494=EDGE_CURVE ( 'NONE', #34043, #32609, #1466, .T. ) ;
#19496=CARTESIAN_POINT ( 'NONE',  ( 2.033800773692430397, 6.875399836226916861, -33.21096214980137518 ) ) ;
#19512=ORIENTED_EDGE ( 'NONE', *, *, #14966, .T. ) ;
#19519=DIRECTION ( 'NONE',  ( 0.000000000000000000, 0.000000000000000000, 1.000000000000000000 ) ) ;
#19524=VERTEX_POINT ( 'NONE', #31880 ) ;
#19543=EDGE_CURVE ( 'NONE', #28747, #32609, #25799, .T. ) ;
#19550=LINE ( 'NONE', #5992, #18323 ) ;
#19574=ORIENTED_EDGE ( 'NONE', *, *, #26275, .T. ) ;
#19594=EDGE_CURVE ( 'NONE', #20222, #15134, #32169, .T. ) ;
#19596=DIRECTION ( 'NONE',  ( 0.000000000000000000, 0.000000000000000000, 1.000000000000000000 ) ) ;
#19599=ORIENTED_EDGE ( 'NONE', *, *, #11078, .F. ) ;
#19603=ORIENTED_EDGE ( 'NONE', *, *, #22151, .F. ) ;
#19606=DIRECTION ( 'NONE',  ( 0.000000000000000000, 0.000000000000000000, 1.000000000000000000 ) ) ;
#19607=CIRCLE ( 'NONE', #33234, 34.41491905851385269 ) ;
#19608=DIRECTION ( 'NONE',  ( 0.000000000000000000, 0.000000000000000000, 1.000000000000000000 ) ) ;
#19615=EDGE_CURVE ( 'NONE', #19094, #29748, #32600, .T. ) ;
#19617=LINE ( 'NONE', #30461, #256 ) ;
#19620=VERTEX_POINT ( 'NONE', #2697 ) ;
#19624=FACE_OUTER_BOUND ( 'NONE', #15392, .T. ) ;
#19636=DIRECTION ( 'NONE',  ( -1.000000000000000000, 0.000000000000000000, -0.000000000000000000 ) ) ;
#19640=CARTESIAN_POINT ( 'NONE',  ( -3.660469135640938497E-16, -11.08319859408599228, -28.58839307351527381 ) ) ;
#19644=ORIENTED_EDGE ( 'NONE', *, *, #15233, .T. ) ;
#19645=B_SPLINE_CURVE_WITH_KNOTS ( 'NONE', 3,
 ( #4268, #31843, #9974, #31509 ),
 .UNSPECIFIED., .F., .F.,
 ( 4, 4 ),
 ( 0.005298361175080963312, 0.005985229640890900142 ),
 .UNSPECIFIED. ) ;
#19646=B_SPLINE_CURVE_WITH_KNOTS ( 'NONE', 3,
 ( #27083, #29234, #2001, #16072 ),
 .UNSPECIFIED., .F., .F.,
 ( 4, 4 ),
 ( 0.0003071994222346450588, 0.0006879348191048121524 ),
 .UNSPECIFIED. ) ;
#19651=DIRECTION ( 'NONE',  ( 0.000000000000000000, 8.881784197001252323E-16, 1.000000000000000000 ) ) ;
#19654=LINE ( 'NONE', #19472, #15635 ) ;
#19660=CARTESIAN_POINT ( 'NONE',  ( 0.000000000000000000, 3.909681563761695067, 30.21863799912385673 ) ) ;
#19678=AXIS2_PLACEMENT_3D ( 'NONE', #23761, #18254, #18782 ) ;
#19681=CARTESIAN_POINT ( 'NONE',  ( 0.02407890056655651728, -3.506335382740735529, 30.89238256715863784 ) ) ;
#19688=ORIENTED_EDGE ( 'NONE', *, *, #12944, .T. ) ;
#19690=ORIENTED_EDGE ( 'NONE', *, *, #14842, .T. ) ;
#19695=EDGE_CURVE ( 'NONE', #2295, #28456, #19795, .T. ) ;
#19696=CARTESIAN_POINT ( 'NONE',  ( 2.789999999999999147, -17.84464379609659446, 24.93395722650000934 ) ) ;
#19699=CARTESIAN_POINT ( 'NONE',  ( 2.789999999999999147, 24.20451283648857554, -19.51346322004903300 ) ) ;
#19702=ORIENTED_EDGE ( 'NONE', *, *, #28761, .T. ) ;
#19716=CARTESIAN_POINT ( 'NONE',  ( 2.783128938119423079, -0.3206953221638416673, 30.86785892350564708 ) ) ;
#19717=ORIENTED_EDGE ( 'NONE', *, *, #20295, .T. ) ;
#19725=CARTESIAN_POINT ( 'NONE',  ( 2.033589655920501116, 14.91861104533755267, 30.45815716957509167 ) ) ;
#19730=CARTESIAN_POINT ( 'NONE',  ( 2.765921099433441999, -29.68817180695669578, -9.232883799364548949 ) ) ;
#19735=CARTESIAN_POINT ( 'NONE',  ( 0.000000000000000000, -29.69698570178010755, -11.75786841620047163 ) ) ;
#19754=CARTESIAN_POINT ( 'NONE',  ( 1.749999999999999778, -33.39989884085096605, 8.296590337300138174 ) ) ;
#19755=ORIENTED_EDGE ( 'NONE', *, *, #28258, .T. ) ;
#19757=ADVANCED_FACE ( 'NONE', ( #13738 ), #10893, .T. ) ;
#19761=ORIENTED_EDGE ( 'NONE', *, *, #28995, .T. ) ;
#19770=CARTESIAN_POINT ( 'NONE',  ( 2.265105867312950938, 31.31301644755038538, -11.56311898902712976 ) ) ;
#19777=ORIENTED_EDGE ( 'NONE', *, *, #32189, .T. ) ;
#19779=AXIS2_PLACEMENT_3D ( 'NONE', #6847, #23248, #9703 ) ;
#19780=CARTESIAN_POINT ( 'NONE',  ( 2.265105904191462738, 13.50646231473634451, 30.52517305359789646 ) ) ;
#19783=ORIENTED_EDGE ( 'NONE', *, *, #16755, .F. ) ;
#19795=LINE ( 'NONE', #29936, #29366 ) ;
#19796=FACE_OUTER_BOUND ( 'NONE', #2136, .T. ) ;
#19804=DIRECTION ( 'NONE',  ( -1.000000000000000000, -0.000000000000000000, -0.000000000000000000 ) ) ;
#19809=CARTESIAN_POINT ( 'NONE',  ( 2.790000000000000924, 12.80000000000000071, 3.000000000000000000 ) ) ;
#19814=ORIENTED_EDGE ( 'NONE', *, *, #6539, .F. ) ;
#19827=CARTESIAN_POINT ( 'NONE',  ( 2.789999999999999147, -3.728217946243117087, 30.24156218513554606 ) ) ;
#19844=ORIENTED_EDGE ( 'NONE', *, *, #31402, .F. ) ;
#19847=CARTESIAN_POINT ( 'NONE',  ( 0.02407890056655608360, -27.96208973699893008, -13.59246946040217630 ) ) ;
#19853=CYLINDRICAL_SURFACE ( 'NONE', #7105, 34.41491905851385269 ) ;
#19860=VECTOR ( 'NONE', #16836, 1000.000000000000000 ) ;
#19867=ORIENTED_EDGE ( 'NONE', *, *, #28085, .T. ) ;
#19881=CARTESIAN_POINT ( 'NONE',  ( 0.000000000000000000, 28.95078156989558948, 9.502838467758177643 ) ) ;
#19889=EDGE_CURVE ( 'NONE', #29292, #31361, #10029, .T. ) ;
#19891=CARTESIAN_POINT ( 'NONE',  ( 0.1835381996566693985, 29.53850320881163682, -12.99634918694980357 ) ) ;
#19893=VERTEX_POINT ( 'NONE', #28323 ) ;
#19900=EDGE_CURVE ( 'NONE', #13768, #21081, #29924, .T. ) ;
#19901=EDGE_CURVE ( 'NONE', #24976, #6398, #4087, .T. ) ;
#19914=CARTESIAN_POINT ( 'NONE',  ( 2.789999999999999591, 27.83606077057228489, 12.85640846290669970 ) ) ;
#19916=EDGE_LOOP ( 'NONE', ( #21028, #4791, #9242, #3862, #5612, #29543, #6914, #32696 ) ) ;
#19919=CARTESIAN_POINT ( 'NONE',  ( 2.790000000000080860, -23.48523522029045196, -19.71414358107291420 ) ) ;
#19927=CARTESIAN_POINT ( 'NONE',  ( 0.02407890056655608360, 29.44518845714779332, -9.980709654879110104 ) ) ;
#19934=EDGE_LOOP ( 'NONE', ( #453, #10855, #12990, #28598, #31017, #33445 ) ) ;
#19951=TOROIDAL_SURFACE ( 'NONE', #10845, 30.47050528711511674, 8.000000000000000000 ) ;
#19953=DIRECTION ( 'NONE',  ( 0.000000000000000000, 0.000000000000000000, 1.000000000000000000 ) ) ;
#19972=AXIS2_PLACEMENT_3D ( 'NONE', #8214, #29942, #13922 ) ;
#19975=AXIS2_PLACEMENT_3D ( 'NONE', #27648, #5921, #11995 ) ;
#19977=CARTESIAN_POINT ( 'NONE',  ( 2.765921099433442443, 30.61125888652961891, 5.439165181699118889 ) ) ;
#19983=CARTESIAN_POINT ( 'NONE',  ( -8.373597507930047958E-14, 11.49192876466713287, 28.42779197342015607 ) ) ;
#19991=VECTOR ( 'NONE', #10868, 1000.000000000000000 ) ;
#19998=VERTEX_POINT ( 'NONE', #4786 ) ;
#20001=CIRCLE ( 'NONE', #1219, 2.525000000000001243 ) ;
#20005=CARTESIAN_POINT ( 'NONE',  ( 0.02407890056655608360, 29.44518845714779332, -9.980709654879110104 ) ) ;
#20011=CARTESIAN_POINT ( 'NONE',  ( 2.790000000000000924, 0.000000000000000000, 0.000000000000000000 ) ) ;
#20020=VECTOR ( 'NONE', #7791, 1000.000000000000000 ) ;
#20030=DIRECTION ( 'NONE',  ( -1.000000000000000000, 0.000000000000000000, -0.000000000000000000 ) ) ;
#20031=DIRECTION ( 'NONE',  ( 0.000000000000000000, 0.000000000000000000, 1.000000000000000000 ) ) ;
#20033=ORIENTED_EDGE ( 'NONE', *, *, #10117, .T. ) ;
#20049=CARTESIAN_POINT ( 'NONE',  ( -5.210000000000000853, 0.000000000000000000, 0.000000000000000000 ) ) ;
#20060=EDGE_CURVE ( 'NONE', #29345, #1567, #34498, .T. ) ;
#20064=ORIENTED_EDGE ( 'NONE', *, *, #30636, .F. ) ;
#20066=EDGE_CURVE ( 'NONE', #7395, #20222, #21067, .T. ) ;
#20085=DIRECTION ( 'NONE',  ( 0.000000000000000000, 0.000000000000000000, 1.000000000000000000 ) ) ;
#20087=CARTESIAN_POINT ( 'NONE',  ( 1.039999999999999591, -25.27164158951584483, 23.36088151536909052 ) ) ;
#20100=CARTESIAN_POINT ( 'NONE',  ( 1.749999999999999778, 34.17636915695680244, 4.045051921974837761 ) ) ;
#20108=EDGE_LOOP ( 'NONE', ( #5047, #13080, #32842, #9648, #27128, #23177 ) ) ;
#20125=ORIENTED_EDGE ( 'NONE', *, *, #10468, .F. ) ;
#20138=DIRECTION ( 'NONE',  ( -1.000000000000000000, -0.000000000000000000, -0.000000000000000000 ) ) ;
#20139=VECTOR ( 'NONE', #11272, 1000.000000000000000 ) ;
#20141=ORIENTED_EDGE ( 'NONE', *, *, #25707, .T. ) ;
#20144=EDGE_CURVE ( 'NONE', #16565, #23973, #32528, .T. ) ;
#20147=CARTESIAN_POINT ( 'NONE',  ( 2.604019705961582165, 31.85364232850774258, -5.239790278972735749 ) ) ;
#20148=EDGE_LOOP ( 'NONE', ( #2549, #29580, #28694, #29788 ) ) ;
#20149=DIRECTION ( 'NONE',  ( 0.000000000000000000, 0.000000000000000000, 1.000000000000000000 ) ) ;
#20155=DIRECTION ( 'NONE',  ( -1.000000000000000000, -0.000000000000000000, -0.000000000000000000 ) ) ;
#20156=DIRECTION ( 'NONE',  ( -1.000000000000000000, 0.000000000000000000, 0.000000000000000000 ) ) ;
#20159=CARTESIAN_POINT ( 'NONE',  ( 0.1835379687083470712, 12.63602821951847233, -29.69442701139029950 ) ) ;
#20160=CARTESIAN_POINT ( 'NONE',  ( 2.765921099435497243, 28.29688452313399338, 12.88099432405614309 ) ) ;
#20165=CARTESIAN_POINT ( 'NONE',  ( 0.5288002592091670673, -32.14027485980077614, -9.048862969376250120 ) ) ;
#20176=EDGE_CURVE ( 'NONE', #15056, #20282, #528, .T. ) ;
#20184=CARTESIAN_POINT ( 'NONE',  ( 0.1859802519188287762, -28.85000931094353049, 14.48402167767607729 ) ) ;
#20185=ADVANCED_FACE ( 'NONE', ( #10850 ), #22235, .T. ) ;
#20189=CARTESIAN_POINT ( 'NONE',  ( 1.749999999999999778, -1.891117961020238436, 34.36292081097831641 ) ) ;
#20197=EDGE_CURVE ( 'NONE', #18398, #21299, #25736, .T. ) ;
#20201=CARTESIAN_POINT ( 'NONE',  ( 0.1835382055501959819, -30.93445778156035786, 9.191712967690730096 ) ) ;
#20202=CARTESIAN_POINT ( 'NONE',  ( 0.02407890056655738464, 24.20451283648857554, -19.51346322004903300 ) ) ;
#20207=CARTESIAN_POINT ( 'NONE',  ( 2.261199744265443901, -1.325911039507465583, 33.36347027112249464 ) ) ;
#20214=CARTESIAN_POINT ( 'NONE',  ( 2.790000000000082636, 30.58763704338517542, 2.144802104989564473 ) ) ;
#20219=ORIENTED_EDGE ( 'NONE', *, *, #30535, .T. ) ;
#20222=VERTEX_POINT ( 'NONE', #8356 ) ;
#20230=VERTEX_POINT ( 'NONE', #19229 ) ;
#20231=LINE ( 'NONE', #34262, #20236 ) ;
#20236=VECTOR ( 'NONE', #28232, 1000.000000000000000 ) ;
#20245=LINE ( 'NONE', #6158, #30852 ) ;
#20246=ORIENTED_EDGE ( 'NONE', *, *, #29687, .F. ) ;
#20250=CARTESIAN_POINT ( 'NONE',  ( 1.395000000000002238, 28.00026196654299682, -20.00929742917093179 ) ) ;
#20251=EDGE_CURVE ( 'NONE', #6306, #4415, #24454, .T. ) ;
#20252=ORIENTED_EDGE ( 'NONE', *, *, #27849, .F. ) ;
#20253=DIRECTION ( 'NONE',  ( 1.000000000000000000, -0.000000000000000000, -0.000000000000000000 ) ) ;
#20258=ADVANCED_FACE ( 'NONE', ( #27392 ), #5840, .T. ) ;
#20262=CARTESIAN_POINT ( 'NONE',  ( 2.765921099433442887, -23.70329957282599764, 20.11932597908820242 ) ) ;
#20272=ORIENTED_EDGE ( 'NONE', *, *, #14398, .F. ) ;
#20278=CARTESIAN_POINT ( 'NONE',  ( 1.040000000000000924, 0.000000000000000000, 0.000000000000000000 ) ) ;
#20282=VERTEX_POINT ( 'NONE', #16734 ) ;
#20291=CARTESIAN_POINT ( 'NONE',  ( 1.749999999999999778, 22.14447232807545163, -26.34405054495532639 ) ) ;
#20295=EDGE_CURVE ( 'NONE', #6345, #8526, #8332, .T. ) ;
#20317=CARTESIAN_POINT ( 'NONE',  ( 2.765921099433442887, 24.20451283648829133, 19.51346322004938827 ) ) ;
#20320=CARTESIAN_POINT ( 'NONE',  ( 1.040000000000001146, -25.27164158951551087, -23.36088151536945645 ) ) ;
#20324=DIRECTION ( 'NONE',  ( -1.000000000000000000, -0.000000000000000000, -0.000000000000000000 ) ) ;
#20329=AXIS2_PLACEMENT_3D ( 'NONE', #34311, #15988, #26299 ) ;
#20332=CARTESIAN_POINT ( 'NONE',  ( 2.397606348813468014, 30.27116788627787614, 13.00174666746673324 ) ) ;
#20337=AXIS2_PLACEMENT_3D ( 'NONE', #2258, #31976, #32328 ) ;
#20340=ORIENTED_EDGE ( 'NONE', *, *, #12466, .F. ) ;
#20345=ORIENTED_EDGE ( 'NONE', *, *, #12797, .F. ) ;
#20352=VERTEX_POINT ( 'NONE', #1224 ) ;
#20354=CARTESIAN_POINT ( 'NONE',  ( 0.02407890056655868569, 24.20451283648829133, 19.51346322004938827 ) ) ;
#20356=ORIENTED_EDGE ( 'NONE', *, *, #24609, .F. ) ;
#20363=ORIENTED_EDGE ( 'NONE', *, *, #34707, .F. ) ;
#20370=CARTESIAN_POINT ( 'NONE',  ( 7.056651121978252318E-16, 23.76428138080773422, -19.37504760381629865 ) ) ;
#20375=VECTOR ( 'NONE', #24967, 1000.000000000000000 ) ;
#20377=CARTESIAN_POINT ( 'NONE',  ( 1.749999999999999778, -1.891117961020238436, 34.36292081097831641 ) ) ;
#20382=EDGE_CURVE ( 'NONE', #31298, #16780, #13017, .T. ) ;
#20386=CYLINDRICAL_SURFACE ( 'NONE', #15440, 34.41491905851385269 ) ;
#20387=EDGE_CURVE ( 'NONE', #9427, #22681, #29953, .T. ) ;
#20397=EDGE_CURVE ( 'NONE', #28359, #30843, #8907, .T. ) ;
#20404=CARTESIAN_POINT ( 'NONE',  ( 0.0001801434340936737804, -25.83993731729792742, -16.24881338200996694 ) ) ;
#20407=DIRECTION ( 'NONE',  ( 0.000000000000000000, -3.435095992033281961E-15, -1.000000000000000000 ) ) ;
#20419=FACE_OUTER_BOUND ( 'NONE', #16281, .T. ) ;
#20427=ORIENTED_EDGE ( 'NONE', *, *, #32617, .F. ) ;
#20456=CARTESIAN_POINT ( 'NONE',  ( 2.765921099433442887, -30.46391896562411716, 6.211548095912460710 ) ) ;
#20464=ORIENTED_EDGE ( 'NONE', *, *, #8713, .T. ) ;
#20471=CARTESIAN_POINT ( 'NONE',  ( 1.040000000000001590, -33.39989884085085947, -8.296590337300607132 ) ) ;
#20472=CARTESIAN_POINT ( 'NONE',  ( 2.789999999999999147, -2.530647759431734922, 30.33427519320593646 ) ) ;
#20479=CARTESIAN_POINT ( 'NONE',  ( 2.606461852600250317, 25.37843598539274126, 19.93397194544903073 ) ) ;
#20487=EDGE_CURVE ( 'NONE', #21040, #28354, #2679, .T. ) ;
#20494=CARTESIAN_POINT ( 'NONE',  ( 1.749999999999999778, 28.00026196654270905, 20.00929742917132970 ) ) ;
#20498=EDGE_CURVE ( 'NONE', #33253, #29665, #14653, .T. ) ;
#20513=EDGE_CURVE ( 'NONE', #16209, #10508, #15159, .T. ) ;
#20515=ORIENTED_EDGE ( 'NONE', *, *, #6355, .T. ) ;
#20518=ORIENTED_EDGE ( 'NONE', *, *, #7901, .T. ) ;
#20521=CARTESIAN_POINT ( 'NONE',  ( 1.039999999999999591, -30.28730148581173864, 16.34215476954022606 ) ) ;
#20524=DIRECTION ( 'NONE',  ( -1.000000000000000000, -0.000000000000000000, 0.000000000000000000 ) ) ;
#20527=CIRCLE ( 'NONE', #1766, 30.47050528711511674 ) ;
#20532=DIRECTION ( 'NONE',  ( 0.000000000000000000, 0.000000000000000000, 1.000000000000000000 ) ) ;
#20541=VECTOR ( 'NONE', #16752, 1000.000000000000000 ) ;
#20549=ORIENTED_EDGE ( 'NONE', *, *, #7630, .T. ) ;
#20555=ORIENTED_EDGE ( 'NONE', *, *, #21210, .F. ) ;
#20573=CARTESIAN_POINT ( 'NONE',  ( 2.790000000000083524, -30.61525927030270822, 1.705757817505451523 ) ) ;
#20579=ORIENTED_EDGE ( 'NONE', *, *, #11507, .T. ) ;
#20582=CARTESIAN_POINT ( 'NONE',  ( 0.000000000000000000, 0.000000000000000000, 0.000000000000000000 ) ) ;
#20594=AXIS2_PLACEMENT_3D ( 'NONE', #13808, #26977, #24118 ) ;
#20604=CARTESIAN_POINT ( 'NONE',  ( 0.1835381808019326266, -27.67670874042560669, 16.59602520068856180 ) ) ;
#20614=AXIS2_PLACEMENT_3D ( 'NONE', #13246, #32795, #24423 ) ;
#20621=CARTESIAN_POINT ( 'NONE',  ( 0.000000000000000000, 0.000000000000000000, 0.000000000000000000 ) ) ;
#20625=CARTESIAN_POINT ( 'NONE',  ( 0.5288002434240788308, 31.32081674369885960, -11.57089561809639733 ) ) ;
#20629=DIRECTION ( 'NONE',  ( 0.000000000000000000, 0.000000000000000000, 1.000000000000000000 ) ) ;
#20633=DIRECTION ( 'NONE',  ( 0.000000000000000000, 0.000000000000000000, 1.000000000000000000 ) ) ;
#20639=B_SPLINE_CURVE_WITH_KNOTS ( 'NONE', 3,
 ( #27662, #2921, #447, #32644 ),
 .UNSPECIFIED., .F., .F.,
 ( 4, 4 ),
 ( 0.005298356295608612834, 0.005985224943342816982 ),
 .UNSPECIFIED. ) ;
#20646=CARTESIAN_POINT ( 'NONE',  ( 2.765921099433441999, -3.506335382740735529, 30.89238256715863784 ) ) ;
#20654=CARTESIAN_POINT ( 'NONE',  ( 2.765921099433441999, -3.506335382740735529, 30.89238256715863784 ) ) ;
#20655=ORIENTED_EDGE ( 'NONE', *, *, #8191, .T. ) ;
#20671=CARTESIAN_POINT ( 'NONE',  ( 0.02407890056655695096, 30.61125888652969707, -5.439165181698684570 ) ) ;
#20672=CARTESIAN_POINT ( 'NONE',  ( 2.789999999999999147, 17.11426446101236820, -24.44276559937708271 ) ) ;
#20678=AXIS2_PLACEMENT_3D ( 'NONE', #24872, #29879, #5819 ) ;
#20679=ORIENTED_EDGE ( 'NONE', *, *, #32440, .T. ) ;
#20703=LINE ( 'NONE', #31550, #12568 ) ;
#20716=CARTESIAN_POINT ( 'NONE',  ( 1.749999999999999778, 0.000000000000000000, 0.000000000000000000 ) ) ;
#20723=CARTESIAN_POINT ( 'NONE',  ( 1.040000000000001368, 6.714005886385424837, -33.75364837705166110 ) ) ;
#20738=CARTESIAN_POINT ( 'NONE',  ( 0.006871226506761134167, -7.987145637396054987, -29.81833655972106456 ) ) ;
#20745=CARTESIAN_POINT ( 'NONE',  ( 0.5288002590641972533, 7.012902549147048248, -32.64503617578034778 ) ) ;
#20752=CARTESIAN_POINT ( 'NONE',  ( 2.789999999999999147, 29.94779062842794559, -5.619744560738758388 ) ) ;
#20756=CARTESIAN_POINT ( 'NONE',  ( 2.765921099433442887, -8.112136323389137260, 30.01377904834206589 ) ) ;
#20762=AXIS2_PLACEMENT_3D ( 'NONE', #23925, #18262, #7730 ) ;
#20765=AXIS2_PLACEMENT_3D ( 'NONE', #13335, #5291, #13670 ) ;
#20767=CARTESIAN_POINT ( 'NONE',  ( 2.789999999999999147, 2.005524111408653720, -29.35189292423236296 ) ) ;
#20770=ORIENTED_EDGE ( 'NONE', *, *, #16755, .T. ) ;
#20785=ORIENTED_EDGE ( 'NONE', *, *, #2968, .F. ) ;
#20790=CARTESIAN_POINT ( 'NONE',  ( 0.02407890056655738464, -27.96208973699912548, 13.59246946040177129 ) ) ;
#20791=CARTESIAN_POINT ( 'NONE',  ( 2.789819856565905809, -25.83993731729781373, -16.24881338200996694 ) ) ;
#20794=B_SPLINE_CURVE_WITH_KNOTS ( 'NONE', 3,
 ( #16900, #16720, #3342, #14039, #14220, #22396 ),
 .UNSPECIFIED., .F., .F.,
 ( 4, 2, 4 ),
 ( 4.404817104921089305E-07, 0.001874269682437042228, 0.003748098883163592659 ),
 .UNSPECIFIED. ) ;
#20795=CARTESIAN_POINT ( 'NONE',  ( 0.02407890056655695096, -21.56796757982795043, -22.39322359481629476 ) ) ;
#20796=CARTESIAN_POINT ( 'NONE',  ( 0.07094832170561987672, 26.43909160613385723, -17.47815001432893922 ) ) ;
#20804=DIRECTION ( 'NONE',  ( -1.000000000000000000, -0.000000000000000000, 0.000000000000000000 ) ) ;
#20818=CARTESIAN_POINT ( 'NONE',  ( 2.783107567989380193, -3.550547054313960338, 30.66493323461383369 ) ) ;
#20823=ADVANCED_FACE ( 'NONE', ( #22855 ), #27116, .T. ) ;
#20831=AXIS2_PLACEMENT_3D ( 'NONE', #11702, #27529, #11884 ) ;
#20836=ORIENTED_EDGE ( 'NONE', *, *, #3591, .T. ) ;
#20838=DIRECTION ( 'NONE',  ( 0.000000000000000000, 0.000000000000000000, -1.000000000000000000 ) ) ;
#20868=CARTESIAN_POINT ( 'NONE',  ( 0.7561992193724378364, 5.833185478271599500, -33.40977515897095884 ) ) ;
#20870=CARTESIAN_POINT ( 'NONE',  ( 0.1835380176977702282, 30.42925477731472839, 10.74656554331707170 ) ) ;
#20873=CARTESIAN_POINT ( 'NONE',  ( 1.040000000000001812, -1.891117961019736393, -34.36292081097834483 ) ) ;
#20874=EDGE_LOOP ( 'NONE', ( #6363, #32908, #12257, #16426 ) ) ;
#20888=CARTESIAN_POINT ( 'NONE',  ( 2.789999999999999147, -20.92506858792740587, -22.14933852381698642 ) ) ;
#20899=AXIS2_PLACEMENT_3D ( 'NONE', #2669, #13889, #24376 ) ;
#20906=DIRECTION ( 'NONE',  ( 0.000000000000000000, 0.000000000000000000, 1.000000000000000000 ) ) ;
#20907=CARTESIAN_POINT ( 'NONE',  ( 2.789999999999999147, -27.96208973699893008, -13.59246946040217630 ) ) ;
#20908=CARTESIAN_POINT ( 'NONE',  ( 1.749999999999999778, 32.09669216789236401, 12.41728656686386500 ) ) ;
#20919=FACE_OUTER_BOUND ( 'NONE', #16884, .T. ) ;
#20927=EDGE_CURVE ( 'NONE', #3499, #24998, #7804, .T. ) ;
#20936=DIRECTION ( 'NONE',  ( 0.000000000000000000, -6.870191984066554061E-16, -1.000000000000000000 ) ) ;
#20945=AXIS2_PLACEMENT_3D ( 'NONE', #24532, #8169, #8527 ) ;
#20955=EDGE_LOOP ( 'NONE', ( #4735, #19049, #16542, #6006, #19324, #23383, #1840, #27599 ) ) ;
#20977=ORIENTED_EDGE ( 'NONE', *, *, #4199, .T. ) ;
#20978=DIRECTION ( 'NONE',  ( -1.000000000000000000, -0.000000000000000000, -0.000000000000000000 ) ) ;
#20987=EDGE_LOOP ( 'NONE', ( #9890, #23394, #21672, #6775 ) ) ;
#20997=CARTESIAN_POINT ( 'NONE',  ( 2.789999999999999147, 18.59128259035472297, 24.91982945642928016 ) ) ;
#20998=CARTESIAN_POINT ( 'NONE',  ( 2.789999999999999147, 24.25608676732976221, 18.39061402768369291 ) ) ;
#21005=DIRECTION ( 'NONE',  ( 0.000000000000000000, 0.000000000000000000, 1.000000000000000000 ) ) ;
#21006=DIRECTION ( 'NONE',  ( 0.000000000000000000, 0.000000000000000000, 1.000000000000000000 ) ) ;
#21007=EDGE_LOOP ( 'NONE', ( #7184, #33587, #32200, #17329 ) ) ;
#21009=CARTESIAN_POINT ( 'NONE',  ( 1.395000000000002238, -25.27164158951584838, 23.36088151536909763 ) ) ;
#21010=B_SPLINE_CURVE_WITH_KNOTS ( 'NONE', 3,
 ( #14064, #19237, #11387, #25069 ),
 .UNSPECIFIED., .F., .F.,
 ( 4, 4 ),
 ( 0.005298347429621228476, 0.005985216133920623523 ),
 .UNSPECIFIED. ) ;
#21024=CARTESIAN_POINT ( 'NONE',  ( 2.789999999999999147, 2.005524111408653720, -29.35189292423236296 ) ) ;
#21027=ORIENTED_EDGE ( 'NONE', *, *, #13064, .F. ) ;
#21028=ORIENTED_EDGE ( 'NONE', *, *, #24987, .T. ) ;
#21033=CARTESIAN_POINT ( 'NONE',  ( 2.789999999999999147, 19.87737664170488827, 23.05346671160913985 ) ) ;
#21034=CARTESIAN_POINT ( 'NONE',  ( 0.7564103444947344324, -10.98355401466475811, 32.08778326629999356 ) ) ;
#21038=DIRECTION ( 'NONE',  ( 0.000000000000000000, 0.000000000000000000, 1.000000000000000000 ) ) ;
#21040=VERTEX_POINT ( 'NONE', #30112 ) ;
#21041=CARTESIAN_POINT ( 'NONE',  ( 0.1835381215211869255, 4.854340785353490340, -31.90397497931449067 ) ) ;
#21062=CARTESIAN_POINT ( 'NONE',  ( -8.176201638302029277E-14, 30.16006060148113832, 5.529416874852006281 ) ) ;
#21064=AXIS2_PLACEMENT_3D ( 'NONE', #14593, #22936, #8874 ) ;
#21066=AXIS2_PLACEMENT_3D ( 'NONE', #33495, #28160, #14995 ) ;
#21067=B_SPLINE_CURVE_WITH_KNOTS ( 'NONE', 3,
 ( #34353, #5140, #24010, #34892, #34530, #7280 ),
 .UNSPECIFIED., .F., .F.,
 ( 4, 2, 4 ),
 ( 4.404817061063498359E-07, 0.001874269649560073936, 0.003748098817414041457 ),
 .UNSPECIFIED. ) ;
#21068=ORIENTED_EDGE ( 'NONE', *, *, #19004, .T. ) ;
#21069=EDGE_CURVE ( 'NONE', #26408, #34260, #455, .T. ) ;
#21080=CARTESIAN_POINT ( 'NONE',  ( 2.789999999999999591, 4.060282914029383683, 30.39157201494050398 ) ) ;
#21081=VERTEX_POINT ( 'NONE', #16609 ) ;
#21085=FACE_OUTER_BOUND ( 'NONE', #8171, .T. ) ;
#21105=CARTESIAN_POINT ( 'NONE',  ( 1.749999999999999778, -24.90160365674851306, -23.75493189058367349 ) ) ;
#21106=CARTESIAN_POINT ( 'NONE',  ( 2.789999999999999147, -13.59935610937951900, -26.37510281771846365 ) ) ;
#21112=ORIENTED_EDGE ( 'NONE', *, *, #11783, .F. ) ;
#21115=VECTOR ( 'NONE', #34107, 1000.000000000000000 ) ;
#21116=CIRCLE ( 'NONE', #28517, 34.41491905851385269 ) ;
#21117=ORIENTED_EDGE ( 'NONE', *, *, #2620, .F. ) ;
#21144=ORIENTED_EDGE ( 'NONE', *, *, #719, .T. ) ;
#21153=ORIENTED_EDGE ( 'NONE', *, *, #14813, .F. ) ;
#21154=CARTESIAN_POINT ( 'NONE',  ( -5.866068224042683378E-16, 7.412728658108713731, 29.75205777216491398 ) ) ;
#21156=LINE ( 'NONE', #29524, #14912 ) ;
#21157=ORIENTED_EDGE ( 'NONE', *, *, #8191, .F. ) ;
#21162=ADVANCED_FACE ( 'NONE', ( #24347 ), #5478, .T. ) ;
#21173=B_SPLINE_CURVE_WITH_KNOTS ( 'NONE', 3,
 ( #2843, #18550, #13709, #21188, #15879, #26703 ),
 .UNSPECIFIED., .F., .F.,
 ( 4, 2, 4 ),
 ( 4.404817019066348049E-07, 0.001874269618538362478, 0.003748098755374818306 ),
 .UNSPECIFIED. ) ;
#21174=LINE ( 'NONE', #34522, #3242 ) ;
#21179=CARTESIAN_POINT ( 'NONE',  ( 2.606461875633085068, 21.48816195191898970, -24.07669289167323967 ) ) ;
#21188=CARTESIAN_POINT ( 'NONE',  ( 2.604019708608551031, -27.68787216339173085, 16.59794162419580132 ) ) ;
#21192=B_SPLINE_CURVE_WITH_KNOTS ( 'NONE', 3,
 ( #18435, #34263, #9879, #2217 ),
 .UNSPECIFIED., .F., .F.,
 ( 4, 4 ),
 ( 0.005298352430873783797, 0.005985221104152193584 ),
 .UNSPECIFIED. ) ;
#21201=ORIENTED_EDGE ( 'NONE', *, *, #16898, .T. ) ;
#21210=EDGE_CURVE ( 'NONE', #21769, #32541, #16016, .T. ) ;
#21217=CARTESIAN_POINT ( 'NONE',  ( 2.604019748081172203, -28.85000931094332444, -14.48402167767649296 ) ) ;
#21230=LINE ( 'NONE', #10739, #17968 ) ;
#21246=B_SPLINE_CURVE_WITH_KNOTS ( 'NONE', 3,
 ( #18023, #26005, #23337, #10161 ),
 .UNSPECIFIED., .F., .F.,
 ( 4, 4 ),
 ( 0.005362286937562653344, 0.005985250355243621097 ),
 .UNSPECIFIED. ) ;
#21253=EDGE_CURVE ( 'NONE', #18600, #14486, #16808, .T. ) ;
#21270=CARTESIAN_POINT ( 'NONE',  ( 0.000000000000000000, -0.09145294252700143789, 30.47036804522410236 ) ) ;
#21279=FACE_OUTER_BOUND ( 'NONE', #21679, .T. ) ;
#21282=VERTEX_POINT ( 'NONE', #26677 ) ;
#21287=LINE ( 'NONE', #7214, #12297 ) ;
#21288=FACE_OUTER_BOUND ( 'NONE', #24927, .T. ) ;
#21299=VERTEX_POINT ( 'NONE', #8569 ) ;
#21302=CARTESIAN_POINT ( 'NONE',  ( 2.765921099434983876, -15.32140196853734970, -27.05343472113007763 ) ) ;
#21321=AXIS2_PLACEMENT_3D ( 'NONE', #3526, #14415, #2997 ) ;
#21322=DIRECTION ( 'NONE',  ( -1.000000000000000000, 0.000000000000000000, 0.000000000000000000 ) ) ;
#21323=CARTESIAN_POINT ( 'NONE',  ( 0.000000000000000000, -29.91351748324107973, 5.799410679710550021 ) ) ;
#21324=ADVANCED_FACE ( 'NONE', ( #29946 ), #7874, .T. ) ;
#21327=B_SPLINE_CURVE_WITH_KNOTS ( 'NONE', 3,
 ( #2711, #18404, #29219, #7698, #29249, #12892 ),
 .UNSPECIFIED., .F., .F.,
 ( 4, 2, 4 ),
 ( 2.434544809778055946E-07, 0.001873441796234163017, 0.003746640137987347977 ),
 .UNSPECIFIED. ) ;
#21337=EDGE_CURVE ( 'NONE', #22114, #19079, #9155, .T. ) ;
#21341=B_SPLINE_CURVE_WITH_KNOTS ( 'NONE', 3,
 ( #9593, #34312, #33970, #20791 ),
 .UNSPECIFIED., .F., .F.,
 ( 4, 4 ),
 ( 0.005298382169618340125, 0.005362286937562653344 ),
 .UNSPECIFIED. ) ;
#21343=ADVANCED_FACE ( 'NONE', ( #29421 ), #21584, .T. ) ;
#21346=ORIENTED_EDGE ( 'NONE', *, *, #20251, .T. ) ;
#21356=AXIS2_PLACEMENT_3D ( 'NONE', #328, #7615, #8146 ) ;
#21370=DIRECTION ( 'NONE',  ( 0.000000000000000000, 0.000000000000000000, -1.000000000000000000 ) ) ;
#21383=CARTESIAN_POINT ( 'NONE',  ( 2.606461878478813166, 4.854340785353028487, 31.90397497931456883 ) ) ;
#21385=DIRECTION ( 'NONE',  ( 0.000000000000000000, 0.000000000000000000, 1.000000000000000000 ) ) ;
#21389=VERTEX_POINT ( 'NONE', #2350 ) ;
#21396=DIRECTION ( 'NONE',  ( -1.000000000000000000, -0.000000000000000000, 0.000000000000000000 ) ) ;
#21401=EDGE_CURVE ( 'NONE', #33010, #1712, #2874, .T. ) ;
#21424=FACE_OUTER_BOUND ( 'NONE', #4367, .T. ) ;
#21436=DIRECTION ( 'NONE',  ( 0.000000000000000000, 0.000000000000000000, 1.000000000000000000 ) ) ;
#21439=ORIENTED_EDGE ( 'NONE', *, *, #8407, .F. ) ;
#21442=CARTESIAN_POINT ( 'NONE',  ( 0.006892390059616927689, 11.66157578832105557, -28.58237449055226165 ) ) ;
#21443=CARTESIAN_POINT ( 'NONE',  ( 2.790000000000081304, 7.412271713510841131, 29.75335163721786103 ) ) ;
#21444=ORIENTED_EDGE ( 'NONE', *, *, #27637, .F. ) ;
#21449=EDGE_CURVE ( 'NONE', #6749, #8018, #18030, .T. ) ;
#21452=ADVANCED_FACE ( 'NONE', ( #17319 ), #25111, .F. ) ;
#21455=CYLINDRICAL_SURFACE ( 'NONE', #27448, 2.524999999999999467 ) ;
#21462=CARTESIAN_POINT ( 'NONE',  ( 0.3923936511923831194, 30.27116788629744804, 13.00174666746672969 ) ) ;
#21475=VERTEX_POINT ( 'NONE', #33658 ) ;
#21480=AXIS2_PLACEMENT_3D ( 'NONE', #956, #28533, #25501 ) ;
#21486=CARTESIAN_POINT ( 'NONE',  ( -10.00000000000000000, 0.000000000000000000, 0.000000000000000000 ) ) ;
#21487=B_SPLINE_CURVE_WITH_KNOTS ( 'NONE', 3,
 ( #30346, #17031, #5948, #33544 ),
 .UNSPECIFIED., .F., .F.,
 ( 4, 4 ),
 ( 0.005298558704933876984, 0.005985424570307887326 ),
 .UNSPECIFIED. ) ;
#21504=ORIENTED_EDGE ( 'NONE', *, *, #24634, .T. ) ;
#21512=DIRECTION ( 'NONE',  ( -1.000000000000000000, -0.000000000000000000, -0.000000000000000000 ) ) ;
#21522=CARTESIAN_POINT ( 'NONE',  ( 0.1835381473997496904, 25.37843598539303258, -19.93397194544865769 ) ) ;
#21547=ORIENTED_EDGE ( 'NONE', *, *, #16264, .F. ) ;
#21554=FACE_OUTER_BOUND ( 'NONE', #1676, .T. ) ;
#21561=VERTEX_POINT ( 'NONE', #20320 ) ;
#21563=TOROIDAL_SURFACE ( 'NONE', #26105, 30.47050528711511674, 8.000000000000000000 ) ;
#21568=CYLINDRICAL_SURFACE ( 'NONE', #31538, 16.19999999999999218 ) ;
#21578=DIRECTION ( 'NONE',  ( 0.000000000000000000, 0.000000000000000000, 1.000000000000000000 ) ) ;
#21580=CYLINDRICAL_SURFACE ( 'NONE', #64, 34.41491905851385269 ) ;
#21584=CYLINDRICAL_SURFACE ( 'NONE', #25442, 34.41491905851385269 ) ;
#21588=CARTESIAN_POINT ( 'NONE',  ( 2.789999999999999147, -27.96208973699912548, 13.59246946040177129 ) ) ;
#21590=CARTESIAN_POINT ( 'NONE',  ( 0.000000000000000000, 17.11426446101199161, 26.96776559937732642 ) ) ;
#21592=CARTESIAN_POINT ( 'NONE',  ( 2.790000000000000480, 25.77033216996941078, -16.61395588374042376 ) ) ;
#21601=ORIENTED_EDGE ( 'NONE', *, *, #6539, .T. ) ;
#21603=CARTESIAN_POINT ( 'NONE',  ( 1.749999999999999778, -25.27164158951585549, 23.36088151536907631 ) ) ;
#21605=VERTEX_POINT ( 'NONE', #12318 ) ;
#21611=CARTESIAN_POINT ( 'NONE',  ( 2.765921099433440222, -27.96208973699893008, -13.59246946040217630 ) ) ;
#21615=DIRECTION ( 'NONE',  ( 0.000000000000000000, -0.9510565162951545304, 0.3090169943749441206 ) ) ;
#21627=CIRCLE ( 'NONE', #18876, 10.00000000000000000 ) ;
#21628=FACE_OUTER_BOUND ( 'NONE', #2893, .T. ) ;
#21632=CARTESIAN_POINT ( 'NONE',  ( 2.789999999999999147, 5.092684668492991840, -30.01061466292821933 ) ) ;
#21645=EDGE_CURVE ( 'NONE', #32274, #18981, #7366, .T. ) ;
#21650=VERTEX_POINT ( 'NONE', #34358 ) ;
#21655=CARTESIAN_POINT ( 'NONE',  ( 2.033589655516955474, 6.875279775961012696, 33.21136585175272415 ) ) ;
#21666=ORIENTED_EDGE ( 'NONE', *, *, #14817, .F. ) ;
#21671=CIRCLE ( 'NONE', #24500, 34.41491905851385269 ) ;
#21672=ORIENTED_EDGE ( 'NONE', *, *, #11503, .F. ) ;
#21673=AXIS2_PLACEMENT_3D ( 'NONE', #7260, #31998, #1929 ) ;
#21679=EDGE_LOOP ( 'NONE', ( #21346, #31714, #25147, #82 ) ) ;
#21684=EDGE_CURVE ( 'NONE', #1771, #18581, #7464, .T. ) ;
#21688=ORIENTED_EDGE ( 'NONE', *, *, #21449, .T. ) ;
#21693=AXIS2_PLACEMENT_3D ( 'NONE', #4244, #10660, #23827 ) ;
#21695=CARTESIAN_POINT ( 'NONE',  ( 1.749999999999999778, -10.89151784028311809, 32.64600270996213283 ) ) ;
#21700=EDGE_CURVE ( 'NONE', #1226, #26104, #11772, .T. ) ;
#21701=CARTESIAN_POINT ( 'NONE',  ( 2.765921099433441110, -27.96208973699912548, 13.59246946040177129 ) ) ;
#21704=AXIS2_PLACEMENT_3D ( 'NONE', #11390, #9767, #12809 ) ;
#21708=ORIENTED_EDGE ( 'NONE', *, *, #10878, .T. ) ;
#21710=FACE_OUTER_BOUND ( 'NONE', #7392, .T. ) ;
#21715=ADVANCED_FACE ( 'NONE', ( #21710 ), #10694, .T. ) ;
#21726=CIRCLE ( 'NONE', #20594, 34.41491905851385269 ) ;
#21728=ORIENTED_EDGE ( 'NONE', *, *, #8064, .F. ) ;
#21732=DIRECTION ( 'NONE',  ( 0.000000000000000000, 0.000000000000000000, -1.000000000000000000 ) ) ;
#21739=EDGE_CURVE ( 'NONE', #13146, #22962, #33421, .T. ) ;
#21740=DIRECTION ( 'NONE',  ( 0.000000000000000000, 0.000000000000000000, 1.000000000000000000 ) ) ;
#21744=DIRECTION ( 'NONE',  ( 0.000000000000000000, 0.000000000000000000, 1.000000000000000000 ) ) ;
#21748=DIRECTION ( 'NONE',  ( -1.000000000000000000, -0.000000000000000000, -0.000000000000000000 ) ) ;
#21757=B_SPLINE_CURVE_WITH_KNOTS ( 'NONE', 3,
 ( #31184, #19640, #17149, #3585 ),
 .UNSPECIFIED., .F., .F.,
 ( 4, 4 ),
 ( 0.005298419352602270690, 0.005985287046740435900 ),
 .UNSPECIFIED. ) ;
#21759=FACE_OUTER_BOUND ( 'NONE', #10537, .T. ) ;
#21767=B_SPLINE_CURVE_WITH_KNOTS ( 'NONE', 3,
 ( #4353, #9881, #20573, #14728 ),
 .UNSPECIFIED., .F., .F.,
 ( 4, 4 ),
 ( 2.042209043309361781E-07, 0.0006879399691689030505 ),
 .UNSPECIFIED. ) ;
#21769=VERTEX_POINT ( 'NONE', #16396 ) ;
#21771=AXIS2_PLACEMENT_3D ( 'NONE', #5337, #15519, #34911 ) ;
#21775=EDGE_LOOP ( 'NONE', ( #28899, #18833, #4904, #1629, #2142, #22387 ) ) ;
#21776=EDGE_LOOP ( 'NONE', ( #15666, #30811, #33973, #3898, #27926, #34002 ) ) ;
#21781=VERTEX_POINT ( 'NONE', #29722 ) ;
#21783=CARTESIAN_POINT ( 'NONE',  ( 0.07098925407227295314, -28.42160548755711247, -14.02701190433918121 ) ) ;
#21786=DIRECTION ( 'NONE',  ( -1.000000000000000000, -0.000000000000000000, -0.000000000000000000 ) ) ;
#21792=CARTESIAN_POINT ( 'NONE',  ( 0.000000000000000000, -13.59935610937951900, -26.37510281771846365 ) ) ;
#21793=CARTESIAN_POINT ( 'NONE',  ( 2.783107593501489951, -30.26126365281908548, 6.099214421699650224 ) ) ;
#21794=CARTESIAN_POINT ( 'NONE',  ( 1.749999999999999778, 0.000000000000000000, 0.000000000000000000 ) ) ;
#21797=ORIENTED_EDGE ( 'NONE', *, *, #13987, .F. ) ;
#21799=AXIS2_PLACEMENT_3D ( 'NONE', #25075, #9072, #6033 ) ;
#21802=DIRECTION ( 'NONE',  ( 0.000000000000000000, -0.4817536741017159341, 0.8763066800438632509 ) ) ;
#21806=CARTESIAN_POINT ( 'NONE',  ( 2.790000000000080860, -21.14989222980560513, 22.20103112977897197 ) ) ;
#21807=CARTESIAN_POINT ( 'NONE',  ( 2.261199750249991869, -32.52406052302377049, -7.554116419246889258 ) ) ;
#21808=ORIENTED_EDGE ( 'NONE', *, *, #27470, .T. ) ;
#21815=ORIENTED_EDGE ( 'NONE', *, *, #31611, .F. ) ;
#21819=CARTESIAN_POINT ( 'NONE',  ( 2.789999999999999147, 30.40449935640660684, -2.004522720844263084 ) ) ;
#21822=ORIENTED_EDGE ( 'NONE', *, *, #4668, .F. ) ;
#21828=CARTESIAN_POINT ( 'NONE',  ( 2.719051659407074606, 7.308651292219749074, 30.83982692225031386 ) ) ;
#21847=AXIS2_PLACEMENT_3D ( 'NONE', #32783, #19636, #22654 ) ;
#21866=VERTEX_POINT ( 'NONE', #11752 ) ;
#21867=ORIENTED_EDGE ( 'NONE', *, *, #21253, .T. ) ;
#21868=ORIENTED_EDGE ( 'NONE', *, *, #28970, .F. ) ;
#21884=EDGE_LOOP ( 'NONE', ( #1997, #26231, #18573, #24163, #23961, #34463, #12120, #23314 ) ) ;
#21889=CYLINDRICAL_SURFACE ( 'NONE', #20899, 16.19999999999999574 ) ;
#21890=DIRECTION ( 'NONE',  ( -1.000000000000000000, -0.000000000000000000, -0.000000000000000000 ) ) ;
#21901=ORIENTED_EDGE ( 'NONE', *, *, #13820, .F. ) ;
#21907=AXIS2_PLACEMENT_3D ( 'NONE', #23569, #18086, #29264 ) ;
#21910=ORIENTED_EDGE ( 'NONE', *, *, #23924, .T. ) ;
#21934=CARTESIAN_POINT ( 'NONE',  ( 2.606461854930495203, 32.14582644238495135, -2.841494734165257885 ) ) ;
#21936=DIRECTION ( 'NONE',  ( 0.000000000000000000, 0.000000000000000000, 1.000000000000000000 ) ) ;
#21950=ADVANCED_FACE ( 'NONE', ( #21279 ), #29467, .T. ) ;
#21960=AXIS2_PLACEMENT_3D ( 'NONE', #23427, #23940, #15430 ) ;
#21964=CARTESIAN_POINT ( 'NONE',  ( 2.789999999999999147, -27.53147453683415335, -13.05640081644869532 ) ) ;
#21965=ORIENTED_EDGE ( 'NONE', *, *, #2036, .F. ) ;
#21975=EDGE_CURVE ( 'NONE', #6239, #28175, #34552, .T. ) ;
#21977=ORIENTED_EDGE ( 'NONE', *, *, #9384, .T. ) ;
#21983=CARTESIAN_POINT ( 'NONE',  ( 2.765921099433442443, 7.350529080603967813, -30.20932655202929595 ) ) ;
#21985=DIRECTION ( 'NONE',  ( 0.000000000000000000, 0.000000000000000000, 1.000000000000000000 ) ) ;
#21986=EDGE_LOOP ( 'NONE', ( #28370, #21808, #28519, #31175, #5435, #15852, #14260, #10597 ) ) ;
#21987=CARTESIAN_POINT ( 'NONE',  ( 0.006892382735981021635, 25.89094059359475253, 16.81082004999792545 ) ) ;
#21990=CIRCLE ( 'NONE', #18577, 30.47050528711511674 ) ;
#21992=EDGE_CURVE ( 'NONE', #23843, #34921, #3967, .T. ) ;
#22000=CARTESIAN_POINT ( 'NONE',  ( 0.000000000000000000, -3.728217946242704972, -30.24156218513559580 ) ) ;
#22023=CARTESIAN_POINT ( 'NONE',  ( 1.040000000000000924, 0.000000000000000000, 0.000000000000000000 ) ) ;
#22031=DIRECTION ( 'NONE',  ( -1.000000000000000000, -0.000000000000000000, -0.000000000000000000 ) ) ;
#22033=ORIENTED_EDGE ( 'NONE', *, *, #11509, .F. ) ;
#22038=ORIENTED_EDGE ( 'NONE', *, *, #30033, .T. ) ;
#22045=CARTESIAN_POINT ( 'NONE',  ( 2.604019708820032530, -32.25918669212989442, 1.206152977787649405 ) ) ;
#22047=AXIS2_PLACEMENT_3D ( 'NONE', #11389, #11039, #14249 ) ;
#22048=CARTESIAN_POINT ( 'NONE',  ( 2.033800774695602165, 14.91862693714182875, -30.45773629169350727 ) ) ;
#22057=AXIS2_PLACEMENT_3D ( 'NONE', #12921, #24270, #24436 ) ;
#22060=CARTESIAN_POINT ( 'NONE',  ( 2.261199749961548378, -23.80541455566248388, 23.41327456068864876 ) ) ;
#22078=CARTESIAN_POINT ( 'NONE',  ( 2.604019707142743112, -3.229344000442307738, -32.11979559073833457 ) ) ;
#22082=ORIENTED_EDGE ( 'NONE', *, *, #33390, .F. ) ;
#22086=ORIENTED_EDGE ( 'NONE', *, *, #22543, .F. ) ;
#22092=EDGE_LOOP ( 'NONE', ( #24195, #23183, #6078, #11095, #8946, #25180, #3642, #6616 ) ) ;
#22097=VECTOR ( 'NONE', #3344, 1000.000000000000000 ) ;
#22107=CYLINDRICAL_SURFACE ( 'NONE', #4005, 34.41491905851385269 ) ;
#22108=CARTESIAN_POINT ( 'NONE',  ( 0.000000000000000000, 14.59907093257217170, 26.74544485249471393 ) ) ;
#22112=CARTESIAN_POINT ( 'NONE',  ( 2.789999999999999147, 0.000000000000000000, 0.000000000000000000 ) ) ;
#22114=VERTEX_POINT ( 'NONE', #27663 ) ;
#22118=CARTESIAN_POINT ( 'NONE',  ( 1.749999999999999778, 0.000000000000000000, 0.000000000000000000 ) ) ;
#22122=DIRECTION ( 'NONE',  ( -1.000000000000000000, -0.000000000000000000, -0.000000000000000000 ) ) ;
#22124=CARTESIAN_POINT ( 'NONE',  ( 1.749999999999999778, 0.000000000000000000, 0.000000000000000000 ) ) ;
#22128=EDGE_LOOP ( 'NONE', ( #4487, #31606, #6770, #16277 ) ) ;
#22136=B_SPLINE_CURVE_WITH_KNOTS ( 'NONE', 3,
 ( #4450, #30827, #2311, #4800, #7471, #34365 ),
 .UNSPECIFIED., .F., .F.,
 ( 4, 2, 4 ),
 ( 4.404817020008189394E-07, 0.001874269619297513683, 0.003748098756893026608 ),
 .UNSPECIFIED. ) ;
#22137=VECTOR ( 'NONE', #31884, 1000.000000000000000 ) ;
#22145=EDGE_CURVE ( 'NONE', #34660, #3220, #16678, .T. ) ;
#22146=EDGE_CURVE ( 'NONE', #32609, #17061, #18966, .T. ) ;
#22151=EDGE_CURVE ( 'NONE', #13451, #7267, #7822, .T. ) ;
#22154=ORIENTED_EDGE ( 'NONE', *, *, #19494, .T. ) ;
#22157=CARTESIAN_POINT ( 'NONE',  ( 1.749999999999999778, -33.26546734453812348, -8.820166447042147695 ) ) ;
#22162=ORIENTED_EDGE ( 'NONE', *, *, #28168, .F. ) ;
#22163=CARTESIAN_POINT ( 'NONE',  ( -10.00000000000000000, 0.000000000000000000, 0.000000000000000000 ) ) ;
#22176=ORIENTED_EDGE ( 'NONE', *, *, #33893, .T. ) ;
#22182=LINE ( 'NONE', #18650, #30147 ) ;
#22183=ORIENTED_EDGE ( 'NONE', *, *, #12361, .T. ) ;
#22184=VERTEX_POINT ( 'NONE', #33892 ) ;
#22189=CARTESIAN_POINT ( 'NONE',  ( 0.1859802930121887965, 14.82665350068137933, -28.67542985682306167 ) ) ;
#22191=EDGE_CURVE ( 'NONE', #33679, #17311, #27839, .T. ) ;
#22193=LINE ( 'NONE', #6510, #31743 ) ;
#22202=CARTESIAN_POINT ( 'NONE',  ( 0.000000000000000000, 11.30192140231230091, 28.29696565125076191 ) ) ;
#22226=ORIENTED_EDGE ( 'NONE', *, *, #33745, .T. ) ;
#22230=AXIS2_PLACEMENT_3D ( 'NONE', #1351, #12223, #25369 ) ;
#22233=ORIENTED_EDGE ( 'NONE', *, *, #559, .F. ) ;
#22235=CYLINDRICAL_SURFACE ( 'NONE', #32785, 16.19999999999999574 ) ;
#22236=ORIENTED_EDGE ( 'NONE', *, *, #20066, .T. ) ;
#22242=VECTOR ( 'NONE', #4790, 1000.000000000000000 ) ;
#22244=AXIS2_PLACEMENT_3D ( 'NONE', #22163, #6122, #20031 ) ;
#22245=CARTESIAN_POINT ( 'NONE',  ( 2.765921099433441110, 11.80989368511462523, 28.76039115933989976 ) ) ;
#22264=CIRCLE ( 'NONE', #3502, 34.41491905851385269 ) ;
#22281=ORIENTED_EDGE ( 'NONE', *, *, #29644, .F. ) ;
#22294=CIRCLE ( 'NONE', #1281, 30.47050528711511674 ) ;
#22299=AXIS2_PLACEMENT_3D ( 'NONE', #2929, #22821, #25654 ) ;
#22317=AXIS2_PLACEMENT_3D ( 'NONE', #13416, #13590, #8057 ) ;
#22320=CARTESIAN_POINT ( 'NONE',  ( 2.265105757022230382, -1.320925567293070424, -33.35364885818402314 ) ) ;
#22322=CARTESIAN_POINT ( 'NONE',  ( 2.765921099433441999, 4.286445725888479608, -30.79383171238939809 ) ) ;
#22326=CARTESIAN_POINT ( 'NONE',  ( 0.7561992252148435067, -2.658747979797246419, -33.81079988514331802 ) ) ;
#22331=CARTESIAN_POINT ( 'NONE',  ( 0.5248942129897558040, 21.86923048072691600, 25.21799932878544581 ) ) ;
#22334=CARTESIAN_POINT ( 'NONE',  ( 2.765921099433441999, 26.03801215795542134, -16.98986790278583570 ) ) ;
#22341=AXIS2_PLACEMENT_3D ( 'NONE', #11620, #20155, #27975 ) ;
#22354=ORIENTED_EDGE ( 'NONE', *, *, #25348, .T. ) ;
#22357=CARTESIAN_POINT ( 'NONE',  ( 2.789999999999999147, 27.98916443103621177, -15.38717335695007904 ) ) ;
#22363=DIRECTION ( 'NONE',  ( 1.000000000000000000, -0.000000000000000000, 0.000000000000000000 ) ) ;
#22370=CARTESIAN_POINT ( 'NONE',  ( 2.789999999999999147, 7.412728658109134727, -29.75205777216480740 ) ) ;
#22378=ORIENTED_EDGE ( 'NONE', *, *, #7733, .F. ) ;
#22379=DIRECTION ( 'NONE',  ( -1.000000000000000000, -0.000000000000000000, -0.000000000000000000 ) ) ;
#22382=ORIENTED_EDGE ( 'NONE', *, *, #6661, .F. ) ;
#22387=ORIENTED_EDGE ( 'NONE', *, *, #13064, .T. ) ;
#22396=CARTESIAN_POINT ( 'NONE',  ( 0.02407890056655868569, -8.112136323388726922, -30.01377904834218668 ) ) ;
#22397=CARTESIAN_POINT ( 'NONE',  ( 2.789999999999999591, 12.80000000000000071, 0.000000000000000000 ) ) ;
#22399=CARTESIAN_POINT ( 'NONE',  ( 2.789999999999999147, 4.286445725888479608, -30.79383171238939809 ) ) ;
#22405=CARTESIAN_POINT ( 'NONE',  ( 2.765921099433440222, -27.96208973699893008, -13.59246946040217630 ) ) ;
#22410=VERTEX_POINT ( 'NONE', #26211 ) ;
#22411=CARTESIAN_POINT ( 'NONE',  ( -10.00000000000000000, 0.000000000000000000, 0.000000000000000000 ) ) ;
#22418=ORIENTED_EDGE ( 'NONE', *, *, #11913, .F. ) ;
#22431=CARTESIAN_POINT ( 'NONE',  ( 1.039999999999999369, -1.891117961020236216, 34.36292081097831641 ) ) ;
#22437=EDGE_CURVE ( 'NONE', #32336, #2950, #27459, .T. ) ;
#22443=CARTESIAN_POINT ( 'NONE',  ( 1.749999999999999778, 14.40815186467775888, 31.25366880301323746 ) ) ;
#22444=AXIS2_PLACEMENT_3D ( 'NONE', #5023, #15920, #5191 ) ;
#22451=DIRECTION ( 'NONE',  ( 0.000000000000000000, 0.000000000000000000, 1.000000000000000000 ) ) ;
#22454=ORIENTED_EDGE ( 'NONE', *, *, #24124, .F. ) ;
#22456=DIRECTION ( 'NONE',  ( 0.000000000000000000, 0.000000000000000000, 1.000000000000000000 ) ) ;
#22457=DIRECTION ( 'NONE',  ( 0.000000000000000000, 0.000000000000000000, 1.000000000000000000 ) ) ;
#22458=CARTESIAN_POINT ( 'NONE',  ( -5.210000000000000853, 0.000000000000000000, 0.000000000000000000 ) ) ;
#22460=ADVANCED_FACE ( 'NONE', ( #6994 ), #34587, .F. ) ;
#22471=CYLINDRICAL_SURFACE ( 'NONE', #33750, 2.525000000000000799 ) ;
#22474=TOROIDAL_SURFACE ( 'NONE', #19081, 30.47050528711512030, 8.000000000000000000 ) ;
#22480=CARTESIAN_POINT ( 'NONE',  ( 0.000000000000000000, -20.92506858792774338, 22.14933852381670221 ) ) ;
#22483=VERTEX_POINT ( 'NONE', #10906 ) ;
#22489=ORIENTED_EDGE ( 'NONE', *, *, #34180, .F. ) ;
#22499=DIRECTION ( 'NONE',  ( 0.000000000000000000, -2.748076793626624385E-15, -1.000000000000000000 ) ) ;
#22501=EDGE_CURVE ( 'NONE', #6306, #16209, #18926, .T. ) ;
#22505=ORIENTED_EDGE ( 'NONE', *, *, #17193, .F. ) ;
#22507=CYLINDRICAL_SURFACE ( 'NONE', #4857, 2.524999999999999467 ) ;
#22511=B_SPLINE_CURVE_WITH_KNOTS ( 'NONE', 3,
 ( #11665, #22515, #31220, #617 ),
 .UNSPECIFIED., .F., .F.,
 ( 4, 4 ),
 ( 0.005298352064454709028, 0.005985220659832061682 ),
 .UNSPECIFIED. ) ;
#22513=DIRECTION ( 'NONE',  ( 0.000000000000000000, 0.000000000000000000, 1.000000000000000000 ) ) ;
#22515=CARTESIAN_POINT ( 'NONE',  ( -5.475207829904333729E-16, -23.48484457444932261, -19.71282888652513066 ) ) ;
#22518=CYLINDRICAL_SURFACE ( 'NONE', #17285, 16.19999999999999574 ) ;
#22525=ORIENTED_EDGE ( 'NONE', *, *, #20927, .F. ) ;
#22526=DIRECTION ( 'NONE',  ( 0.000000000000000000, 0.000000000000000000, 1.000000000000000000 ) ) ;
#22533=ORIENTED_EDGE ( 'NONE', *, *, #25455, .F. ) ;
#22543=EDGE_CURVE ( 'NONE', #26161, #18440, #30321, .T. ) ;
#22544=CARTESIAN_POINT ( 'NONE',  ( 0.07094833146048340478, -31.01658195443398824, 6.517894193012690351 ) ) ;
#22550=FACE_OUTER_BOUND ( 'NONE', #6408, .T. ) ;
#22551=DIRECTION ( 'NONE',  ( -1.000000000000000000, 0.000000000000000000, 0.000000000000000000 ) ) ;
#22558=CARTESIAN_POINT ( 'NONE',  ( 0.02407890056655738464, 28.29688452313417812, -12.88099432405573630 ) ) ;
#22568=AXIS2_PLACEMENT_3D ( 'NONE', #28282, #12276, #27920 ) ;
#22569=ORIENTED_EDGE ( 'NONE', *, *, #6299, .T. ) ;
#22578=DIRECTION ( 'NONE',  ( -1.000000000000000000, -0.000000000000000000, -0.000000000000000000 ) ) ;
#22586=CARTESIAN_POINT ( 'NONE',  ( 1.749999999999999778, 34.10861917999622506, -4.581348211831717698 ) ) ;
#22597=EDGE_CURVE ( 'NONE', #23843, #10663, #25300, .T. ) ;
#22598=CARTESIAN_POINT ( 'NONE',  ( 0.7564103381736747567, 31.72524275137206828, -11.99054900124176193 ) ) ;
#22600=CIRCLE ( 'NONE', #18067, 30.47050528711512030 ) ;
#22622=VERTEX_POINT ( 'NONE', #9469 ) ;
#22623=CIRCLE ( 'NONE', #24885, 2.525000000000000799 ) ;
#22627=CYLINDRICAL_SURFACE ( 'NONE', #9675, 16.19999999999999929 ) ;
#22643=CARTESIAN_POINT ( 'NONE',  ( 2.789999999999999147, 13.51972826729850041, -27.27250221666277596 ) ) ;
#22653=AXIS2_PLACEMENT_3D ( 'NONE', #29584, #32416, #8036 ) ;
#22654=DIRECTION ( 'NONE',  ( 0.000000000000000000, 0.000000000000000000, 1.000000000000000000 ) ) ;
#22657=CYLINDRICAL_SURFACE ( 'NONE', #21066, 2.525000000000001243 ) ;
#22660=CARTESIAN_POINT ( 'NONE',  ( 0.02407890056655695096, 11.80989368511462523, 28.76039115933989976 ) ) ;
#22666=CIRCLE ( 'NONE', #28351, 2.525000000000001243 ) ;
#22681=VERTEX_POINT ( 'NONE', #25824 ) ;
#22686=LINE ( 'NONE', #5453, #10834 ) ;
#22687=CARTESIAN_POINT ( 'NONE',  ( 2.783128806874977990, 29.25797949657086860, 9.843693408253784582 ) ) ;
#22693=CARTESIAN_POINT ( 'NONE',  ( 0.000000000000000000, 3.909681563762119172, -30.21863799912381054 ) ) ;
#22699=DIRECTION ( 'NONE',  ( -1.000000000000000000, 0.000000000000000000, 0.000000000000000000 ) ) ;
#22702=CARTESIAN_POINT ( 'NONE',  ( 2.789999999999999147, -0.09145294252654824485, -30.47036804522408460 ) ) ;
#22708=VERTEX_POINT ( 'NONE', #13021 ) ;
#22713=EDGE_LOOP ( 'NONE', ( #25291, #10921, #16848, #17658, #343, #2829 ) ) ;
#22725=CYLINDRICAL_SURFACE ( 'NONE', #2141, 34.41491905851385269 ) ;
#22731=CARTESIAN_POINT ( 'NONE',  ( 2.783107588261252374, 7.365885187734460438, -29.97812926094515973 ) ) ;
#22733=CARTESIAN_POINT ( 'NONE',  ( 0.000000000000000000, -17.83604598421647935, -24.70480026434186982 ) ) ;
#22746=VERTEX_POINT ( 'NONE', #9635 ) ;
#22748=EDGE_CURVE ( 'NONE', #17861, #34482, #31341, .T. ) ;
#22750=FACE_OUTER_BOUND ( 'NONE', #20987, .T. ) ;
#22756=DIRECTION ( 'NONE',  ( 0.000000000000000000, 0.000000000000000000, 1.000000000000000000 ) ) ;
#22762=CARTESIAN_POINT ( 'NONE',  ( -10.00000000000000000, 0.000000000000000000, 0.000000000000000000 ) ) ;
#22767=ORIENTED_EDGE ( 'NONE', *, *, #23425, .F. ) ;
#22786=AXIS2_PLACEMENT_3D ( 'NONE', #25912, #29282, #29459 ) ;
#22788=VERTEX_POINT ( 'NONE', #183 ) ;
#22789=EDGE_CURVE ( 'NONE', #9953, #11863, #16594, .T. ) ;
#22793=CARTESIAN_POINT ( 'NONE',  ( 0.000000000000000000, -30.41598411195408502, -1.821977758773957179 ) ) ;
#22799=DIRECTION ( 'NONE',  ( 0.000000000000000000, 0.000000000000000000, 1.000000000000000000 ) ) ;
#22800=CARTESIAN_POINT ( 'NONE',  ( 50.00050000000000239, 12.80000000000000071, 3.000000000000000000 ) ) ;
#22802=ORIENTED_EDGE ( 'NONE', *, *, #33228, .T. ) ;
#22803=ORIENTED_EDGE ( 'NONE', *, *, #10687, .F. ) ;
#22808=CARTESIAN_POINT ( 'NONE',  ( 2.261199741344610104, 33.02096244749633769, -4.949265406681700341 ) ) ;
#22821=DIRECTION ( 'NONE',  ( -1.000000000000000000, -0.000000000000000000, -0.000000000000000000 ) ) ;
#22827=CIRCLE ( 'NONE', #644, 30.47050528711512030 ) ;
#22848=CARTESIAN_POINT ( 'NONE',  ( 2.789999999999999147, 18.92047747027354987, 23.84508255125859222 ) ) ;
#22851=EDGE_CURVE ( 'NONE', #1613, #8699, #29911, .T. ) ;
#22855=FACE_OUTER_BOUND ( 'NONE', #28703, .T. ) ;
#22859=CIRCLE ( 'NONE', #8611, 34.41491905851385269 ) ;
#22866=CARTESIAN_POINT ( 'NONE',  ( 0.07098930928321604827, 21.26205330531119841, 23.50467731722566356 ) ) ;
#22874=DIRECTION ( 'NONE',  ( 0.000000000000000000, 0.000000000000000000, -1.000000000000000000 ) ) ;
#22875=ADVANCED_FACE ( 'NONE', ( #11040 ), #1805, .T. ) ;
#22891=VERTEX_POINT ( 'NONE', #16574 ) ;
#22902=CARTESIAN_POINT ( 'NONE',  ( 2.765921099433440666, -11.07880054387200985, -29.04985141099774637 ) ) ;
#22909=AXIS2_PLACEMENT_3D ( 'NONE', #26611, #10420, #4529 ) ;
#22935=CARTESIAN_POINT ( 'NONE',  ( 2.719051664247837508, 31.58891575048174971, 2.579090161526253144 ) ) ;
#22936=DIRECTION ( 'NONE',  ( -1.000000000000000000, -0.000000000000000000, -0.000000000000000000 ) ) ;
#22941=B_SPLINE_CURVE_WITH_KNOTS ( 'NONE', 3,
 ( #18298, #29661, #29129, #21302 ),
 .UNSPECIFIED., .F., .F.,
 ( 4, 4 ),
 ( 0.005298346101779219386, 0.005985214792934989356 ),
 .UNSPECIFIED. ) ;
#22942=EDGE_CURVE ( 'NONE', #33679, #9083, #12077, .T. ) ;
#22950=CARTESIAN_POINT ( 'NONE',  ( 1.749999999999999778, -10.37741591188871482, -32.81304455236878681 ) ) ;
#22955=CARTESIAN_POINT ( 'NONE',  ( 2.790000000000000924, 9.539392014169456147, -3.000000000000000000 ) ) ;
#22962=VERTEX_POINT ( 'NONE', #11758 ) ;
#22986=DIRECTION ( 'NONE',  ( 0.000000000000000000, 0.000000000000000000, 1.000000000000000000 ) ) ;
#23010=AXIS2_PLACEMENT_3D ( 'NONE', #19735, #33423, #24878 ) ;
#23012=B_SPLINE_CURVE_WITH_KNOTS ( 'NONE', 3,
 ( #16431, #32249, #15911, #24765 ),
 .UNSPECIFIED., .F., .F.,
 ( 4, 4 ),
 ( 0.005298366463358164004, 0.005985234859393915273 ),
 .UNSPECIFIED. ) ;
#23013=CARTESIAN_POINT ( 'NONE',  ( 2.789999999999999147, 24.20451283648829133, 19.51346322004938827 ) ) ;
#23020=ORIENTED_EDGE ( 'NONE', *, *, #25305, .T. ) ;
#23026=DIRECTION ( 'NONE',  ( 0.000000000000000000, 0.000000000000000000, 1.000000000000000000 ) ) ;
#23035=TOROIDAL_SURFACE ( 'NONE', #850, 30.47050528711511674, 8.000000000000000000 ) ;
#23036=FACE_OUTER_BOUND ( 'NONE', #32021, .T. ) ;
#23043=ADVANCED_FACE ( 'NONE', ( #14067 ), #24902, .F. ) ;
#23048=LINE ( 'NONE', #6825, #15004 ) ;
#23050=CARTESIAN_POINT ( 'NONE',  ( 0.006871072277270173605, 20.89672672272023135, -22.72123193261218432 ) ) ;
#23052=CARTESIAN_POINT ( 'NONE',  ( 1.040000000000001146, -2.430610048906252985, 34.32897884578299852 ) ) ;
#23057=AXIS2_PLACEMENT_3D ( 'NONE', #16163, #35027, #31979 ) ;
#23062=EDGE_LOOP ( 'NONE', ( #12858, #11488, #2331, #24512 ) ) ;
#23065=ORIENTED_EDGE ( 'NONE', *, *, #30169, .F. ) ;
#23074=ORIENTED_EDGE ( 'NONE', *, *, #12857, .F. ) ;
#23077=FACE_OUTER_BOUND ( 'NONE', #13129, .T. ) ;
#23085=ORIENTED_EDGE ( 'NONE', *, *, #30535, .F. ) ;
#23090=ORIENTED_EDGE ( 'NONE', *, *, #9982, .F. ) ;
#23096=CARTESIAN_POINT ( 'NONE',  ( -8.386830662123268555E-14, 23.76564585742992719, 19.37518496788528211 ) ) ;
#23106=ORIENTED_EDGE ( 'NONE', *, *, #26224, .T. ) ;
#23111=ADVANCED_FACE ( 'NONE', ( #15475 ), #30806, .T. ) ;
#23128=EDGE_CURVE ( 'NONE', #9083, #21605, #152, .T. ) ;
#23138=PLANE ( 'NONE',  #21673 ) ;
#23143=ORIENTED_EDGE ( 'NONE', *, *, #5807, .F. ) ;
#23152=AXIS2_PLACEMENT_3D ( 'NONE', #12303, #29363, #7104 ) ;
#23153=EDGE_CURVE ( 'NONE', #10340, #34596, #27737, .T. ) ;
#23160=ORIENTED_EDGE ( 'NONE', *, *, #34265, .T. ) ;
#23172=PLANE ( 'NONE',  #8850 ) ;
#23177=ORIENTED_EDGE ( 'NONE', *, *, #25868, .T. ) ;
#23180=VERTEX_POINT ( 'NONE', #16177 ) ;
#23183=ORIENTED_EDGE ( 'NONE', *, *, #6327, .T. ) ;
#23190=VERTEX_POINT ( 'NONE', #34865 ) ;
#23193=AXIS2_PLACEMENT_3D ( 'NONE', #32257, #8044, #5538 ) ;
#23194=CIRCLE ( 'NONE', #22047, 34.41491905851385269 ) ;
#23203=CARTESIAN_POINT ( 'NONE',  ( 1.749999999999999778, -30.28730148581173864, 16.34215476954022606 ) ) ;
#23211=ORIENTED_EDGE ( 'NONE', *, *, #17089, .T. ) ;
#23219=CARTESIAN_POINT ( 'NONE',  ( 2.604019711028809692, -0.8217981779194966085, 32.27126551972443025 ) ) ;
#23220=VERTEX_POINT ( 'NONE', #8670 ) ;
#23221=DIRECTION ( 'NONE',  ( 1.000000000000000000, 0.000000000000000000, 0.000000000000000000 ) ) ;
#23236=CARTESIAN_POINT ( 'NONE',  ( 0.1859802892437388833, -18.30372525367501524, 26.59104308589815702 ) ) ;
#23245=ORIENTED_EDGE ( 'NONE', *, *, #7812, .F. ) ;
#23248=DIRECTION ( 'NONE',  ( -1.000000000000000000, -0.000000000000000000, -0.000000000000000000 ) ) ;
#23249=CARTESIAN_POINT ( 'NONE',  ( 2.789999999999999147, -21.56796757982826307, 22.39322359481599278 ) ) ;
#23263=VERTEX_POINT ( 'NONE', #30918 ) ;
#23267=CIRCLE ( 'NONE', #9055, 34.41491905851385269 ) ;
#23270=LINE ( 'NONE', #31615, #21115 ) ;
#23276=VERTEX_POINT ( 'NONE', #17243 ) ;
#23284=ORIENTED_EDGE ( 'NONE', *, *, #27849, .T. ) ;
#23286=ORIENTED_EDGE ( 'NONE', *, *, #24126, .F. ) ;
#23289=DIRECTION ( 'NONE',  ( 0.000000000000000000, 1.374038396813311798E-15, -1.000000000000000000 ) ) ;
#23291=CIRCLE ( 'NONE', #5072, 30.47050528711512030 ) ;
#23293=CARTESIAN_POINT ( 'NONE',  ( 2.033800783032481796, -32.97757984916182039, 7.919492155587937177 ) ) ;
#23302=EDGE_CURVE ( 'NONE', #29908, #23325, #12879, .T. ) ;
#23314=ORIENTED_EDGE ( 'NONE', *, *, #9845, .F. ) ;
#23323=DIRECTION ( 'NONE',  ( -1.000000000000000000, 0.000000000000000000, 0.000000000000000000 ) ) ;
#23325=VERTEX_POINT ( 'NONE', #25930 ) ;
#23327=CARTESIAN_POINT ( 'NONE',  ( 2.033589661659781722, 21.20732892273832704, -26.46721543659820242 ) ) ;
#23329=ORIENTED_EDGE ( 'NONE', *, *, #27568, .T. ) ;
#23332=CARTESIAN_POINT ( 'NONE',  ( 1.749999999999999778, -25.27164158951550732, -23.36088151536945645 ) ) ;
#23335=ADVANCED_FACE ( 'NONE', ( #33764 ), #19378, .T. ) ;
#23337=CARTESIAN_POINT ( 'NONE',  ( 2.781508616055402339, -26.25561000592817607, -16.27441264773137419 ) ) ;
#23345=VERTEX_POINT ( 'NONE', #28770 ) ;
#23358=ORIENTED_EDGE ( 'NONE', *, *, #16566, .F. ) ;
#23362=CARTESIAN_POINT ( 'NONE',  ( 2.789999999999999147, 26.03801215795542134, -16.98986790278583570 ) ) ;
#23363=CARTESIAN_POINT ( 'NONE',  ( 1.040000000000001590, 32.09669216789235691, 12.41728656686385968 ) ) ;
#23371=ORIENTED_EDGE ( 'NONE', *, *, #17337, .T. ) ;
#23383=ORIENTED_EDGE ( 'NONE', *, *, #15999, .T. ) ;
#23388=ORIENTED_EDGE ( 'NONE', *, *, #14348, .F. ) ;
#23393=CARTESIAN_POINT ( 'NONE',  ( 1.040000000000000924, 0.000000000000000000, 0.000000000000000000 ) ) ;
#23394=ORIENTED_EDGE ( 'NONE', *, *, #18916, .F. ) ;
#23401=LINE ( 'NONE', #13084, #5158 ) ;
#23402=B_SPLINE_CURVE_WITH_KNOTS ( 'NONE', 3,
 ( #32426, #2013, #15547, #32258, #7876, #31892 ),
 .UNSPECIFIED., .F., .F.,
 ( 4, 2, 4 ),
 ( 2.333473478908367993E-07, 0.001873431678079542006, 0.003746630008811193454 ),
 .UNSPECIFIED. ) ;
#23409=CARTESIAN_POINT ( 'NONE',  ( 1.040000000000001368, -33.26546734453825138, 8.820166447041648539 ) ) ;
#23413=VERTEX_POINT ( 'NONE', #15431 ) ;
#23425=EDGE_CURVE ( 'NONE', #8710, #14706, #9389, .T. ) ;
#23427=CARTESIAN_POINT ( 'NONE',  ( 2.789999999999999147, 9.869977788040968036, 30.37666815053940539 ) ) ;
#23431=ORIENTED_EDGE ( 'NONE', *, *, #32339, .T. ) ;
#23438=ORIENTED_EDGE ( 'NONE', *, *, #33193, .T. ) ;
#23441=LINE ( 'NONE', #34296, #19020 ) ;
#23446=VERTEX_POINT ( 'NONE', #35002 ) ;
#23470=B_SPLINE_CURVE_WITH_KNOTS ( 'NONE', 3,
 ( #20005, #30849, #9314, #10188 ),
 .UNSPECIFIED., .F., .F.,
 ( 4, 4 ),
 ( 3.346525879906762451E-07, 0.0006880714927763405177 ),
 .UNSPECIFIED. ) ;
#23476=AXIS2_PLACEMENT_3D ( 'NONE', #27305, #30336, #18969 ) ;
#23489=CYLINDRICAL_SURFACE ( 'NONE', #23817, 16.19999999999999574 ) ;
#23494=ADVANCED_FACE ( 'NONE', ( #21288 ), #2408, .T. ) ;
#23496=CARTESIAN_POINT ( 'NONE',  ( 2.789999999999999147, 14.59907093257254296, -26.74544485249450787 ) ) ;
#23499=CARTESIAN_POINT ( 'NONE',  ( 2.783107618827354024, -21.36453267519060617, -22.28230728414027340 ) ) ;
#23504=DIRECTION ( 'NONE',  ( -1.000000000000000000, 0.000000000000000000, 0.000000000000000000 ) ) ;
#23514=CARTESIAN_POINT ( 'NONE',  ( 0.7561992140789179917, -9.974544214302882850, 32.41523709743427872 ) ) ;
#23515=CARTESIAN_POINT ( 'NONE',  ( 0.5288002571296349652, -28.88016830755685405, -16.75753762755175558 ) ) ;
#23518=ORIENTED_EDGE ( 'NONE', *, *, #7786, .T. ) ;
#23519=VERTEX_POINT ( 'NONE', #16137 ) ;
#23520=VERTEX_POINT ( 'NONE', #31950 ) ;
#23525=ORIENTED_EDGE ( 'NONE', *, *, #29386, .F. ) ;
#23532=CARTESIAN_POINT ( 'NONE',  ( 2.789999999999999147, 14.59907093257254296, -26.74544485249450787 ) ) ;
#23535=ORIENTED_EDGE ( 'NONE', *, *, #12233, .T. ) ;
#23546=VERTEX_POINT ( 'NONE', #17328 ) ;
#23556=AXIS2_PLACEMENT_3D ( 'NONE', #33856, #17152, #25833 ) ;
#23569=CARTESIAN_POINT ( 'NONE',  ( 2.789999999999999147, 0.000000000000000000, 0.000000000000000000 ) ) ;
#23577=ADVANCED_FACE ( 'NONE', ( #19327 ), #1284, .F. ) ;
#23578=TOROIDAL_SURFACE ( 'NONE', #4255, 30.47050528711511674, 8.000000000000000000 ) ;
#23579=DIRECTION ( 'NONE',  ( -1.000000000000000000, -0.000000000000000000, 0.000000000000000000 ) ) ;
#23587=CIRCLE ( 'NONE', #23010, 2.525000000000001243 ) ;
#23588=LINE ( 'NONE', #29458, #8465 ) ;
#23593=CARTESIAN_POINT ( 'NONE',  ( -5.210000000000000853, 0.000000000000000000, 0.000000000000000000 ) ) ;
#23599=ORIENTED_EDGE ( 'NONE', *, *, #25707, .F. ) ;
#23600=AXIS2_PLACEMENT_3D ( 'NONE', #31198, #4121, #15184 ) ;
#23609=CIRCLE ( 'NONE', #21356, 30.47050528711512030 ) ;
#23617=EDGE_CURVE ( 'NONE', #14065, #8194, #7432, .T. ) ;
#23618=ORIENTED_EDGE ( 'NONE', *, *, #1686, .T. ) ;
#23622=EDGE_CURVE ( 'NONE', #12785, #33069, #13752, .T. ) ;
#23631=ADVANCED_FACE ( 'NONE', ( #6430 ), #22657, .F. ) ;
#23660=B_SPLINE_CURVE_WITH_KNOTS ( 'NONE', 3,
 ( #6900, #22598, #20625, #25427, #25600, #19927 ),
 .UNSPECIFIED., .F., .F.,
 ( 4, 2, 4 ),
 ( 4.404817133663990876E-07, 0.001874269703891902252, 0.003748098926070445210 ),
 .UNSPECIFIED. ) ;
#23664=EDGE_CURVE ( 'NONE', #1613, #12821, #26476, .T. ) ;
#23670=VERTEX_POINT ( 'NONE', #12328 ) ;
#23674=CARTESIAN_POINT ( 'NONE',  ( 1.749999999999999778, 22.14447232807545163, -26.34405054495532639 ) ) ;
#23684=B_SPLINE_CURVE_WITH_KNOTS ( 'NONE', 3,
 ( #5221, #21783, #10402, #2737, #26949, #5049 ),
 .UNSPECIFIED., .F., .F.,
 ( 4, 2, 4 ),
 ( 2.717607641618553552E-07, 0.001873470133380086616, 0.003746668505996011457 ),
 .UNSPECIFIED. ) ;
#23692=DIRECTION ( 'NONE',  ( -1.000000000000000000, 0.000000000000000000, -0.000000000000000000 ) ) ;
#23711=ORIENTED_EDGE ( 'NONE', *, *, #2174, .F. ) ;
#23716=LINE ( 'NONE', #24231, #27180 ) ;
#23725=AXIS2_PLACEMENT_3D ( 'NONE', #16972, #41, #8405 ) ;
#23742=AXIS2_PLACEMENT_3D ( 'NONE', #5253, #637, #32487 ) ;
#23743=ORIENTED_EDGE ( 'NONE', *, *, #22942, .T. ) ;
#23746=VERTEX_POINT ( 'NONE', #12850 ) ;
#23761=CARTESIAN_POINT ( 'NONE',  ( 2.789999999999999147, 30.11551674275786539, -4.430359003076015156 ) ) ;
#23769=VERTEX_POINT ( 'NONE', #18197 ) ;
#23771=CARTESIAN_POINT ( 'NONE',  ( 2.765921099433444219, 31.00221527374952046, 2.344426712874309260 ) ) ;
#23781=DIRECTION ( 'NONE',  ( -1.000000000000000000, -0.000000000000000000, 0.000000000000000000 ) ) ;
#23799=CARTESIAN_POINT ( 'NONE',  ( 0.1859802861825020359, 32.15598440394879276, -2.846506069495843949 ) ) ;
#23811=DIRECTION ( 'NONE',  ( -1.000000000000000000, 0.000000000000000000, -0.000000000000000000 ) ) ;
#23817=AXIS2_PLACEMENT_3D ( 'NONE', #20998, #23323, #34169 ) ;
#23822=DIRECTION ( 'NONE',  ( -1.000000000000000000, -0.000000000000000000, -0.000000000000000000 ) ) ;
#23825=CARTESIAN_POINT ( 'NONE',  ( 1.040000000000000924, 0.000000000000000000, 0.000000000000000000 ) ) ;
#23827=DIRECTION ( 'NONE',  ( 0.000000000000000000, 6.183172785659898852E-15, -1.000000000000000000 ) ) ;
#23828=ADVANCED_FACE ( 'NONE', ( #21554 ), #8185, .T. ) ;
#23832=ORIENTED_EDGE ( 'NONE', *, *, #20144, .T. ) ;
#23843=VERTEX_POINT ( 'NONE', #24546 ) ;
#23844=CARTESIAN_POINT ( 'NONE',  ( 2.765921099433442443, 20.99477179376858871, -22.93149026599722617 ) ) ;
#23847=DIRECTION ( 'NONE',  ( 0.000000000000000000, 0.9822872507286906085, -0.1873813145857145812 ) ) ;
#23850=DIRECTION ( 'NONE',  ( 0.000000000000000000, 0.000000000000000000, 1.000000000000000000 ) ) ;
#23853=ADVANCED_FACE ( 'NONE', ( #32565 ), #29734, .T. ) ;
#23855=DIRECTION ( 'NONE',  ( 0.000000000000000000, 0.000000000000000000, 1.000000000000000000 ) ) ;
#23859=DIRECTION ( 'NONE',  ( 0.000000000000000000, 0.000000000000000000, 1.000000000000000000 ) ) ;
#23863=EDGE_CURVE ( 'NONE', #1712, #26408, #28187, .T. ) ;
#23864=EDGE_CURVE ( 'NONE', #27613, #27823, #190, .T. ) ;
#23868=EDGE_CURVE ( 'NONE', #7179, #32232, #543, .T. ) ;
#23873=CARTESIAN_POINT ( 'NONE',  ( 0.02407890056655695096, 20.99477179376825120, 22.93149026599753526 ) ) ;
#23879=CARTESIAN_POINT ( 'NONE',  ( 0.02407890056655781832, 7.350529080603967813, -30.20932655202929595 ) ) ;
#23880=CARTESIAN_POINT ( 'NONE',  ( 2.789999999999999147, 0.000000000000000000, 0.000000000000000000 ) ) ;
#23898=ORIENTED_EDGE ( 'NONE', *, *, #20387, .T. ) ;
#23906=EDGE_LOOP ( 'NONE', ( #27290, #2772, #31754, #18616, #34902, #22183 ) ) ;
#23908=AXIS2_PLACEMENT_3D ( 'NONE', #34091, #26251, #18259 ) ;
#23914=ORIENTED_EDGE ( 'NONE', *, *, #9982, .T. ) ;
#23920=DIRECTION ( 'NONE',  ( -1.000000000000000000, -0.000000000000000000, -0.000000000000000000 ) ) ;
#23923=EDGE_CURVE ( 'NONE', #3220, #7946, #13678, .T. ) ;
#23924=EDGE_CURVE ( 'NONE', #7441, #13039, #27670, .T. ) ;
#23925=CARTESIAN_POINT ( 'NONE',  ( 2.789999999999999147, 9.869977788041397915, -30.37666815053925973 ) ) ;
#23930=CARTESIAN_POINT ( 'NONE',  ( 0.02407890056655868569, -8.112136323388726922, -30.01377904834218668 ) ) ;
#23938=ORIENTED_EDGE ( 'NONE', *, *, #2101, .F. ) ;
#23940=DIRECTION ( 'NONE',  ( -1.000000000000000000, 0.000000000000000000, 0.000000000000000000 ) ) ;
#23945=CARTESIAN_POINT ( 'NONE',  ( 2.765921099433441999, -21.56796757982826307, 22.39322359481599278 ) ) ;
#23947=ORIENTED_EDGE ( 'NONE', *, *, #16775, .F. ) ;
#23954=ORIENTED_EDGE ( 'NONE', *, *, #33828, .F. ) ;
#23958=FACE_OUTER_BOUND ( 'NONE', #947, .T. ) ;
#23961=ORIENTED_EDGE ( 'NONE', *, *, #20513, .T. ) ;
#23973=VERTEX_POINT ( 'NONE', #20291 ) ;
#23975=CARTESIAN_POINT ( 'NONE',  ( 0.02407890056655564992, -30.46391896562411716, 6.211548095912460710 ) ) ;
#23977=EDGE_LOOP ( 'NONE', ( #12410, #18252, #26438, #33032, #20679, #34794, #22226, #14761 ) ) ;
#23979=CARTESIAN_POINT ( 'NONE',  ( 0.006871066869920603760, 30.78681169157792041, -2.258271426746185195 ) ) ;
#23986=CARTESIAN_POINT ( 'NONE',  ( 2.765921099433441999, -0.3931553186915530129, 31.08824725498900321 ) ) ;
#23992=ORIENTED_EDGE ( 'NONE', *, *, #16687, .F. ) ;
#23994=CIRCLE ( 'NONE', #20614, 2.525000000000000355 ) ;
#23996=AXIS2_PLACEMENT_3D ( 'NONE', #25161, #17543, #22513 ) ;
#24001=ORIENTED_EDGE ( 'NONE', *, *, #10167, .F. ) ;
#24004=EDGE_CURVE ( 'NONE', #22962, #22410, #24697, .T. ) ;
#24005=EDGE_CURVE ( 'NONE', #32629, #26161, #34936, .T. ) ;
#24007=DIRECTION ( 'NONE',  ( -1.000000000000000000, -0.000000000000000000, -0.000000000000000000 ) ) ;
#24010=CARTESIAN_POINT ( 'NONE',  ( 0.5288002521483733398, 5.497007441955001461, 32.93420861807582867 ) ) ;
#24020=CARTESIAN_POINT ( 'NONE',  ( 0.7564103431398414568, -1.600050605839945961, -33.87778227150288757 ) ) ;
#24023=CARTESIAN_POINT ( 'NONE',  ( 2.789999999999999147, 23.28319895603611300, -21.86437915510192909 ) ) ;
#24025=VECTOR ( 'NONE', #24208, 1000.000000000000000 ) ;
#24029=LINE ( 'NONE', #21024, #34198 ) ;
#24030=ORIENTED_EDGE ( 'NONE', *, *, #18898, .F. ) ;
#24042=ADVANCED_FACE ( 'NONE', ( #15304 ), #4761, .F. ) ;
#24051=ADVANCED_FACE ( 'NONE', ( #31649 ), #23138, .T. ) ;
#24052=DIRECTION ( 'NONE',  ( -1.000000000000000000, -0.000000000000000000, 0.000000000000000000 ) ) ;
#24080=ORIENTED_EDGE ( 'NONE', *, *, #21700, .T. ) ;
#24083=ORIENTED_EDGE ( 'NONE', *, *, #12540, .T. ) ;
#24086=DIRECTION ( 'NONE',  ( -1.000000000000000000, -0.000000000000000000, -0.000000000000000000 ) ) ;
#24096=ORIENTED_EDGE ( 'NONE', *, *, #32779, .F. ) ;
#24098=TOROIDAL_SURFACE ( 'NONE', #16150, 30.47050528711512030, 8.000000000000000000 ) ;
#24101=CIRCLE ( 'NONE', #6500, 2.524999999999999467 ) ;
#24102=CARTESIAN_POINT ( 'NONE',  ( 1.040000000000000924, 0.000000000000000000, 0.000000000000000000 ) ) ;
#24107=CARTESIAN_POINT ( 'NONE',  ( 2.261199753130818113, -9.581412748858477713, 31.98555481955049729 ) ) ;
#24108=ORIENTED_EDGE ( 'NONE', *, *, #31402, .T. ) ;
#24113=CARTESIAN_POINT ( 'NONE',  ( 0.02407890056655738464, 26.03801215795517621, 16.98986790278620873 ) ) ;
#24118=DIRECTION ( 'NONE',  ( 0.000000000000000000, 0.000000000000000000, 1.000000000000000000 ) ) ;
#24124=EDGE_CURVE ( 'NONE', #22483, #11290, #33021, .T. ) ;
#24125=CIRCLE ( 'NONE', #22444, 2.524999999999999467 ) ;
#24126=EDGE_CURVE ( 'NONE', #13256, #13866, #8198, .T. ) ;
#24140=FACE_OUTER_BOUND ( 'NONE', #5484, .T. ) ;
#24150=VECTOR ( 'NONE', #10638, 1000.000000000000000 ) ;
#24151=CARTESIAN_POINT ( 'NONE',  ( 0.02407890056655651728, 18.59128259035506758, -24.91982945642901726 ) ) ;
#24163=ORIENTED_EDGE ( 'NONE', *, *, #22501, .T. ) ;
#24164=DIRECTION ( 'NONE',  ( 0.000000000000000000, 1.374038396813312784E-15, -1.000000000000000000 ) ) ;
#24185=EDGE_CURVE ( 'NONE', #11691, #8132, #5814, .T. ) ;
#24194=CARTESIAN_POINT ( 'NONE',  ( 2.789999999999999147, -0.3931553186911057041, -31.08824725498900676 ) ) ;
#24195=ORIENTED_EDGE ( 'NONE', *, *, #26483, .T. ) ;
#24197=DIRECTION ( 'NONE',  ( -1.000000000000000000, -0.000000000000000000, -0.000000000000000000 ) ) ;
#24199=ORIENTED_EDGE ( 'NONE', *, *, #13471, .T. ) ;
#24206=CARTESIAN_POINT ( 'NONE',  ( -10.00000000000000000, 0.000000000000000000, 0.000000000000000000 ) ) ;
#24208=DIRECTION ( 'NONE',  ( -1.000000000000000000, 0.000000000000000000, 0.000000000000000000 ) ) ;
#24213=ORIENTED_EDGE ( 'NONE', *, *, #31545, .F. ) ;
#24214=CARTESIAN_POINT ( 'NONE',  ( 2.789999999999999147, -22.61000311763359250, 20.38038735157074655 ) ) ;
#24220=DIRECTION ( 'NONE',  ( 0.000000000000000000, 3.435095992033281961E-15, -1.000000000000000000 ) ) ;
#24230=CARTESIAN_POINT ( 'NONE',  ( 0.07098930855017421271, 4.557722287734508271, -31.36513882472102210 ) ) ;
#24231=CARTESIAN_POINT ( 'NONE',  ( 2.789999999999999147, -31.05158812718222450, 1.559667679918499417 ) ) ;
#24233=DIRECTION ( 'NONE',  ( 0.000000000000000000, 0.000000000000000000, -1.000000000000000000 ) ) ;
#24252=EDGE_CURVE ( 'NONE', #7193, #34878, #12073, .T. ) ;
#24260=EDGE_LOOP ( 'NONE', ( #3160, #3495, #31186, #19333, #3141, #24725 ) ) ;
#24266=DIRECTION ( 'NONE',  ( -1.000000000000000000, -0.000000000000000000, -0.000000000000000000 ) ) ;
#24270=DIRECTION ( 'NONE',  ( -1.000000000000000000, 0.000000000000000000, 0.000000000000000000 ) ) ;
#24291=CARTESIAN_POINT ( 'NONE',  ( 2.033589663287954430, 27.74660763222603066, 19.50359089280082614 ) ) ;
#24302=ORIENTED_EDGE ( 'NONE', *, *, #26634, .F. ) ;
#24319=LINE ( 'NONE', #5270, #29031 ) ;
#24324=DIRECTION ( 'NONE',  ( 0.000000000000000000, 0.000000000000000000, 1.000000000000000000 ) ) ;
#24333=CIRCLE ( 'NONE', #27750, 34.41491905851385269 ) ;
#24341=EDGE_CURVE ( 'NONE', #6008, #27613, #25138, .T. ) ;
#24345=B_SPLINE_CURVE_WITH_KNOTS ( 'NONE', 3,
 ( #12391, #21080, #7361, #17737 ),
 .UNSPECIFIED., .F., .F.,
 ( 4, 4 ),
 ( 0.005298356295608590283, 0.005985224943342820451 ),
 .UNSPECIFIED. ) ;
#24347=FACE_OUTER_BOUND ( 'NONE', #7286, .T. ) ;
#24353=VERTEX_POINT ( 'NONE', #6701 ) ;
#24356=EDGE_CURVE ( 'NONE', #18581, #33069, #22859, .T. ) ;
#24361=ORIENTED_EDGE ( 'NONE', *, *, #8064, .T. ) ;
#24362=CARTESIAN_POINT ( 'NONE',  ( 0.7564103383402180913, 21.20732892273795756, 26.46721543659850795 ) ) ;
#24367=VERTEX_POINT ( 'NONE', #3505 ) ;
#24376=DIRECTION ( 'NONE',  ( 0.000000000000000000, 0.000000000000000000, 1.000000000000000000 ) ) ;
#24378=EDGE_CURVE ( 'NONE', #13039, #29128, #19550, .T. ) ;
#24382=CARTESIAN_POINT ( 'NONE',  ( -8.222411227241363201E-14, -17.84469521343992326, 24.93532764985518568 ) ) ;
#24383=FACE_OUTER_BOUND ( 'NONE', #10181, .T. ) ;
#24384=CYLINDRICAL_SURFACE ( 'NONE', #14961, 16.19999999999999574 ) ;
#24392=CARTESIAN_POINT ( 'NONE',  ( 2.789999999999999147, 30.27116788629740185, 3.198253332533701698 ) ) ;
#24399=ORIENTED_EDGE ( 'NONE', *, *, #32441, .T. ) ;
#24405=CARTESIAN_POINT ( 'NONE',  ( 2.789999999999999147, -3.506335382740735529, 30.89238256715863784 ) ) ;
#24407=EDGE_CURVE ( 'NONE', #17012, #30030, #17107, .T. ) ;
#24415=CARTESIAN_POINT ( 'NONE',  ( -8.208060149029089991E-14, -23.48523522029074329, 19.71414358107259091 ) ) ;
#24422=ORIENTED_EDGE ( 'NONE', *, *, #27771, .F. ) ;
#24423=DIRECTION ( 'NONE',  ( 0.000000000000000000, 0.9510565162951500895, 0.3090169943749579984 ) ) ;
#24426=ORIENTED_EDGE ( 'NONE', *, *, #18459, .F. ) ;
#24428=ORIENTED_EDGE ( 'NONE', *, *, #4200, .F. ) ;
#24435=LINE ( 'NONE', #15945, #3746 ) ;
#24436=DIRECTION ( 'NONE',  ( 0.000000000000000000, 0.000000000000000000, 1.000000000000000000 ) ) ;
#24441=AXIS2_PLACEMENT_3D ( 'NONE', #18735, #7667, #7488 ) ;
#24454=B_SPLINE_CURVE_WITH_KNOTS ( 'NONE', 3,
 ( #21701, #32548, #16917, #8698, #8167, #14239 ),
 .UNSPECIFIED., .F., .F.,
 ( 4, 2, 4 ),
 ( 2.717607641618062802E-07, 0.001873470133380088784, 0.003746668505996015794 ),
 .UNSPECIFIED. ) ;
#24456=CARTESIAN_POINT ( 'NONE',  ( 2.789999999999999147, 27.98916443103598439, 15.38717335695048227 ) ) ;
#24458=ORIENTED_EDGE ( 'NONE', *, *, #14398, .T. ) ;
#24471=CARTESIAN_POINT ( 'NONE',  ( 2.265105808055940972, -23.79505697368644235, -23.40952781232680024 ) ) ;
#24479=CARTESIAN_POINT ( 'NONE',  ( 2.789999999999999147, 14.59907093257217170, 26.74544485249471393 ) ) ;
#24493=EDGE_CURVE ( 'NONE', #21561, #9083, #23270, .T. ) ;
#24494=CARTESIAN_POINT ( 'NONE',  ( 2.789999999999999147, -29.69698570178010755, -11.75786841620047163 ) ) ;
#24500=AXIS2_PLACEMENT_3D ( 'NONE', #29550, #12837, #21006 ) ;
#24509=B_SPLINE_CURVE_WITH_KNOTS ( 'NONE', 3,
 ( #9359, #31074, #6675, #2168, #10352, #34565 ),
 .UNSPECIFIED., .F., .F.,
 ( 4, 2, 4 ),
 ( 4.404817065346997443E-07, 0.001874269648071526803, 0.003748098814436519148 ),
 .UNSPECIFIED. ) ;
#24512=ORIENTED_EDGE ( 'NONE', *, *, #33390, .T. ) ;
#24515=DIRECTION ( 'NONE',  ( 1.000000000000000000, 0.000000000000000000, -0.000000000000000000 ) ) ;
#24516=CARTESIAN_POINT ( 'NONE',  ( 0.000000000000000000, 20.79173593595263370, 22.27454621808773538 ) ) ;
#24517=LINE ( 'NONE', #29705, #10236 ) ;
#24519=ORIENTED_EDGE ( 'NONE', *, *, #4549, .F. ) ;
#24520=VERTEX_POINT ( 'NONE', #31271 ) ;
#24522=CARTESIAN_POINT ( 'NONE',  ( -8.483176869585901368E-14, -30.61525927030269756, -1.705757817505873630 ) ) ;
#24527=DIRECTION ( 'NONE',  ( -1.000000000000000000, -0.000000000000000000, 0.000000000000000000 ) ) ;
#24532=CARTESIAN_POINT ( 'NONE',  ( 2.789999999999999147, 17.11426446101236820, -26.96776559937708129 ) ) ;
#24537=DIRECTION ( 'NONE',  ( 0.000000000000000000, 0.000000000000000000, 1.000000000000000000 ) ) ;
#24546=CARTESIAN_POINT ( 'NONE',  ( 2.765921099434983876, -15.32140196853734970, -27.05343472113007763 ) ) ;
#24574=DIRECTION ( 'NONE',  ( 0.000000000000000000, 0.000000000000000000, 1.000000000000000000 ) ) ;
#24579=DIRECTION ( 'NONE',  ( -1.000000000000000000, -0.000000000000000000, -0.000000000000000000 ) ) ;
#24580=DIRECTION ( 'NONE',  ( 0.000000000000000000, 0.000000000000000000, 1.000000000000000000 ) ) ;
#24583=CIRCLE ( 'NONE', #18367, 10.00000000000000000 ) ;
#24585=EDGE_CURVE ( 'NONE', #21475, #6239, #30803, .T. ) ;
#24586=CARTESIAN_POINT ( 'NONE',  ( 2.765921099433442443, 31.00221527374952046, -2.344426712874310148 ) ) ;
#24590=CARTESIAN_POINT ( 'NONE',  ( 2.783107617264021005, 25.89094059359499056, -16.81082004999754531 ) ) ;
#24592=CARTESIAN_POINT ( 'NONE',  ( 0.02407890056655695096, -26.45933846664182099, -16.32596387352474565 ) ) ;
#24594=CARTESIAN_POINT ( 'NONE',  ( 2.719010676553170303, -31.66360817300141406, -1.400248398912504300 ) ) ;
#24603=AXIS2_PLACEMENT_3D ( 'NONE', #10907, #7879, #5714 ) ;
#24606=ORIENTED_EDGE ( 'NONE', *, *, #26141, .F. ) ;
#24609=EDGE_CURVE ( 'NONE', #23520, #13039, #21726, .T. ) ;
#24621=TOROIDAL_SURFACE ( 'NONE', #24647, 30.47050528711512030, 8.000000000000000000 ) ;
#24629=EDGE_LOOP ( 'NONE', ( #9597, #9306, #2229, #14161, #23388, #7849 ) ) ;
#24630=TOROIDAL_SURFACE ( 'NONE', #767, 30.47050528711511674, 8.000000000000000000 ) ;
#24632=CARTESIAN_POINT ( 'NONE',  ( -5.210000000000000853, 0.000000000000000000, 0.000000000000000000 ) ) ;
#24634=EDGE_CURVE ( 'NONE', #13694, #26431, #10728, .T. ) ;
#24636=CARTESIAN_POINT ( 'NONE',  ( 0.02407890056655695096, 20.99477179376858871, -22.93149026599722617 ) ) ;
#24647=AXIS2_PLACEMENT_3D ( 'NONE', #22458, #33312, #13857 ) ;
#24649=CARTESIAN_POINT ( 'NONE',  ( 2.789999999999999147, 2.005524111408653720, -31.87689292423236154 ) ) ;
#24667=DIRECTION ( 'NONE',  ( -1.000000000000000000, -0.000000000000000000, -0.000000000000000000 ) ) ;
#24678=CARTESIAN_POINT ( 'NONE',  ( 8.000000000000000000, 0.000000000000000000, 0.000000000000000000 ) ) ;
#24695=ADVANCED_FACE ( 'NONE', ( #33000 ), #628, .T. ) ;
#24697=B_SPLINE_CURVE_WITH_KNOTS ( 'NONE', 3,
 ( #25968, #12460, #15129, #4242 ),
 .UNSPECIFIED., .F., .F.,
 ( 4, 4 ),
 ( 0.005298382169618362676, 0.005985250355243617627 ),
 .UNSPECIFIED. ) ;
#24705=ORIENTED_EDGE ( 'NONE', *, *, #17990, .T. ) ;
#24710=CARTESIAN_POINT ( 'NONE',  ( 2.765921099433441555, 18.59128259035472297, 24.91982945642928016 ) ) ;
#24712=CARTESIAN_POINT ( 'NONE',  ( 2.033589659158014040, -24.35732449877370343, 23.60053042972024784 ) ) ;
#24714=ORIENTED_EDGE ( 'NONE', *, *, #10497, .F. ) ;
#24716=AXIS2_PLACEMENT_3D ( 'NONE', #191, #18891, #13198 ) ;
#24718=ORIENTED_EDGE ( 'NONE', *, *, #17850, .F. ) ;
#24725=ORIENTED_EDGE ( 'NONE', *, *, #9450, .F. ) ;
#24728=CARTESIAN_POINT ( 'NONE',  ( 0.5288002557345565791, -1.325911039506977307, -33.36347027112250885 ) ) ;
#24734=AXIS2_PLACEMENT_3D ( 'NONE', #13832, #24667, #32859 ) ;
#24758=ORIENTED_EDGE ( 'NONE', *, *, #17990, .F. ) ;
#24765=CARTESIAN_POINT ( 'NONE',  ( 2.765921099433442887, 24.20451283648829133, 19.51346322004938827 ) ) ;
#24769=CARTESIAN_POINT ( 'NONE',  ( 2.604019747054050260, -16.26694784591052922, 27.88362116434737814 ) ) ;
#24784=AXIS2_PLACEMENT_3D ( 'NONE', #15408, #17574, #9544 ) ;
#24788=EDGE_CURVE ( 'NONE', #30647, #33874, #10661, .T. ) ;
#24790=ORIENTED_EDGE ( 'NONE', *, *, #16737, .F. ) ;
#24796=DIRECTION ( 'NONE',  ( 0.000000000000000000, 0.000000000000000000, 1.000000000000000000 ) ) ;
#24806=CARTESIAN_POINT ( 'NONE',  ( 1.040000000000001368, 14.40815186467820652, -31.25366880301302785 ) ) ;
#24811=CARTESIAN_POINT ( 'NONE',  ( 1.749999999999999778, 6.183021911001840287, 33.85493898757064812 ) ) ;
#24827=CARTESIAN_POINT ( 'NONE',  ( 1.040000000000001590, 27.68252950111337896, 20.44661865013498314 ) ) ;
#24832=ORIENTED_EDGE ( 'NONE', *, *, #34321, .F. ) ;
#24838=CARTESIAN_POINT ( 'NONE',  ( 2.765921099433441999, -17.95514392185434360, 25.38201125280350468 ) ) ;
#24850=CARTESIAN_POINT ( 'NONE',  ( 2.789999999999999147, 7.489092610871509237, -29.53582882395378562 ) ) ;
#24853=CARTESIAN_POINT ( 'NONE',  ( 2.789999999999999147, 3.909681563762101852, -30.21863799912378923 ) ) ;
#24855=CARTESIAN_POINT ( 'NONE',  ( 1.749999999999999778, 0.000000000000000000, 0.000000000000000000 ) ) ;
#24872=CARTESIAN_POINT ( 'NONE',  ( 2.789999999999999147, 9.869977788041397915, -30.37666815053925973 ) ) ;
#24878=DIRECTION ( 'NONE',  ( 0.000000000000000000, 1.374038396813311798E-15, -1.000000000000000000 ) ) ;
#24884=CARTESIAN_POINT ( 'NONE',  ( 2.789999999999999147, -8.112136323388726922, -30.01377904834218668 ) ) ;
#24885=AXIS2_PLACEMENT_3D ( 'NONE', #33519, #16644, #22499 ) ;
#24888=ORIENTED_EDGE ( 'NONE', *, *, #30244, .T. ) ;
#24889=CARTESIAN_POINT ( 'NONE',  ( 1.040000000000001146, 21.72796464722008025, 26.68861566460903134 ) ) ;
#24902=CYLINDRICAL_SURFACE ( 'NONE', #21704, 2.525000000000001243 ) ;
#24916=CARTESIAN_POINT ( 'NONE',  ( 2.765921099433440222, -27.96208973699893008, -13.59246946040217630 ) ) ;
#24917=AXIS2_PLACEMENT_3D ( 'NONE', #19437, #5695, #32938 ) ;
#24921=DIRECTION ( 'NONE',  ( -1.000000000000000000, -0.000000000000000000, 0.000000000000000000 ) ) ;
#24927=EDGE_LOOP ( 'NONE', ( #28560, #1401, #26462, #2025 ) ) ;
#24942=ADVANCED_FACE ( 'NONE', ( #13840 ), #14357, .T. ) ;
#24948=EDGE_CURVE ( 'NONE', #17643, #8335, #27980, .T. ) ;
#24954=AXIS2_PLACEMENT_3D ( 'NONE', #11868, #30181, #25184 ) ;
#24967=DIRECTION ( 'NONE',  ( -1.000000000000000000, 0.000000000000000000, 0.000000000000000000 ) ) ;
#24969=VERTEX_POINT ( 'NONE', #11524 ) ;
#24976=VERTEX_POINT ( 'NONE', #2792 ) ;
#24977=CARTESIAN_POINT ( 'NONE',  ( 0.02407890056655651728, 29.44518845714764765, 9.980709654879525772 ) ) ;
#24984=CARTESIAN_POINT ( 'NONE',  ( 0.02407890056655738464, -29.68817180695669578, -9.232883799364548949 ) ) ;
#24987=EDGE_CURVE ( 'NONE', #27741, #24998, #29750, .T. ) ;
#24991=CARTESIAN_POINT ( 'NONE',  ( 2.397606348813468014, 30.27116788627787614, 13.00174666746673324 ) ) ;
#24995=B_SPLINE_CURVE_WITH_KNOTS ( 'NONE', 3,
 ( #5352, #16772, #32581, #19089 ),
 .UNSPECIFIED., .F., .F.,
 ( 4, 4 ),
 ( 0.005298360586756124813, 0.005985229062776062023 ),
 .UNSPECIFIED. ) ;
#24998=VERTEX_POINT ( 'NONE', #33223 ) ;
#25005=AXIS2_PLACEMENT_3D ( 'NONE', #4462, #7850, #18039 ) ;
#25007=FACE_OUTER_BOUND ( 'NONE', #27, .T. ) ;
#25009=CARTESIAN_POINT ( 'NONE',  ( 2.765921099433443331, 14.63235270440974922, -27.43224275967423509 ) ) ;
#25010=CARTESIAN_POINT ( 'NONE',  ( 0.000000000000000000, 27.60935207499572996, -12.89090262359622585 ) ) ;
#25011=VERTEX_POINT ( 'NONE', #30201 ) ;
#25015=DIRECTION ( 'NONE',  ( 0.000000000000000000, 0.000000000000000000, 1.000000000000000000 ) ) ;
#25019=DIRECTION ( 'NONE',  ( -1.000000000000000000, -0.000000000000000000, -0.000000000000000000 ) ) ;
#25024=DIRECTION ( 'NONE',  ( -1.000000000000000000, -0.000000000000000000, -0.000000000000000000 ) ) ;
#25026=EDGE_CURVE ( 'NONE', #20230, #15534, #14385, .T. ) ;
#25036=CARTESIAN_POINT ( 'NONE',  ( 0.02407890056655738464, -29.68817180695669578, -9.232883799364548949 ) ) ;
#25051=ORIENTED_EDGE ( 'NONE', *, *, #559, .T. ) ;
#25059=CARTESIAN_POINT ( 'NONE',  ( 2.783128938602190683, -17.88422427744433207, -25.16112242373455032 ) ) ;
#25064=ORIENTED_EDGE ( 'NONE', *, *, #24126, .T. ) ;
#25069=CARTESIAN_POINT ( 'NONE',  ( 2.765921099433442443, 29.44518845714779332, -9.980709654879110104 ) ) ;
#25075=CARTESIAN_POINT ( 'NONE',  ( 2.789999999999999147, 18.92047747027389448, -23.84508255125831866 ) ) ;
#25079=VECTOR ( 'NONE', #18751, 1000.000000000000000 ) ;
#25082=ORIENTED_EDGE ( 'NONE', *, *, #3366, .T. ) ;
#25083=AXIS2_PLACEMENT_3D ( 'NONE', #4825, #2996, #14232 ) ;
#25086=ORIENTED_EDGE ( 'NONE', *, *, #21210, .T. ) ;
#25099=CARTESIAN_POINT ( 'NONE',  ( 0.02407890056655608360, 29.44518845714779332, -9.980709654879110104 ) ) ;
#25110=LINE ( 'NONE', #3574, #11167 ) ;
#25111=CYLINDRICAL_SURFACE ( 'NONE', #10618, 10.00000000000000000 ) ;
#25130=ADVANCED_FACE ( 'NONE', ( #9715 ), #30734, .F. ) ;
#25134=EDGE_LOOP ( 'NONE', ( #19512, #31816, #3939, #30174, #2192, #17431, #28047, #4795 ) ) ;
#25136=EDGE_CURVE ( 'NONE', #1617, #23519, #20245, .T. ) ;
#25138=B_SPLINE_CURVE_WITH_KNOTS ( 'NONE', 3,
 ( #674, #19725, #28071, #14746, #16890, #14567 ),
 .UNSPECIFIED., .F., .F.,
 ( 4, 2, 4 ),
 ( 4.404817011119805222E-07, 0.001874269612720299216, 0.003748098743739486718 ),
 .UNSPECIFIED. ) ;
#25145=EDGE_LOOP ( 'NONE', ( #3166, #517, #27673, #6896, #12431, #27043 ) ) ;
#25147=ORIENTED_EDGE ( 'NONE', *, *, #12125, .T. ) ;
#25153=FACE_OUTER_BOUND ( 'NONE', #3192, .T. ) ;
#25161=CARTESIAN_POINT ( 'NONE',  ( 2.789999999999999147, -29.69698570178027808, 11.75786841620004175 ) ) ;
#25164=CARTESIAN_POINT ( 'NONE',  ( -10.00000000000000000, 0.000000000000000000, 0.000000000000000000 ) ) ;
#25165=FACE_OUTER_BOUND ( 'NONE', #8343, .T. ) ;
#25166=ORIENTED_EDGE ( 'NONE', *, *, #30283, .F. ) ;
#25176=DIRECTION ( 'NONE',  ( -1.000000000000000000, -0.000000000000000000, -0.000000000000000000 ) ) ;
#25180=ORIENTED_EDGE ( 'NONE', *, *, #33044, .T. ) ;
#25181=ORIENTED_EDGE ( 'NONE', *, *, #14842, .F. ) ;
#25184=DIRECTION ( 'NONE',  ( 0.000000000000000000, 0.000000000000000000, 1.000000000000000000 ) ) ;
#25193=CARTESIAN_POINT ( 'NONE',  ( 2.719051678778256154, 12.21437217961392818, -29.24586132675238304 ) ) ;
#25198=DIRECTION ( 'NONE',  ( 0.000000000000000000, 0.000000000000000000, 1.000000000000000000 ) ) ;
#25201=CARTESIAN_POINT ( 'NONE',  ( 2.765921099433442443, 7.350529080603967813, -30.20932655202929595 ) ) ;
#25212=ADVANCED_FACE ( 'NONE', ( #1708 ), #29110, .T. ) ;
#25221=VECTOR ( 'NONE', #33895, 1000.000000000000000 ) ;
#25237=B_SPLINE_CURVE_WITH_KNOTS ( 'NONE', 3,
 ( #8546, #9056, #30765, #30598 ),
 .UNSPECIFIED., .F., .F.,
 ( 4, 4 ),
 ( 2.010610498844524495E-07, 0.0006879367828356808224 ),
 .UNSPECIFIED. ) ;
#25249=ORIENTED_EDGE ( 'NONE', *, *, #18902, .F. ) ;
#25277=DIRECTION ( 'NONE',  ( 0.000000000000000000, 0.000000000000000000, 1.000000000000000000 ) ) ;
#25281=CARTESIAN_POINT ( 'NONE',  ( 8.000000000000000000, 0.000000000000000000, 0.000000000000000000 ) ) ;
#25284=VERTEX_POINT ( 'NONE', #7559 ) ;
#25287=EDGE_CURVE ( 'NONE', #5322, #20352, #18452, .T. ) ;
#25291=ORIENTED_EDGE ( 'NONE', *, *, #3094, .T. ) ;
#25292=CARTESIAN_POINT ( 'NONE',  ( 2.033589661826324946, 31.72524275137189065, 11.99054900124222200 ) ) ;
#25293=CIRCLE ( 'NONE', #15662, 10.00000000000000000 ) ;
#25295=B_SPLINE_CURVE_WITH_KNOTS ( 'NONE', 3,
 ( #9938, #31640, #30381, #10529 ),
 .UNSPECIFIED., .F., .F.,
 ( 4, 4 ),
 ( 2.702373194995073782E-07, 0.0006880065385067164448 ),
 .UNSPECIFIED. ) ;
#25300=LINE ( 'NONE', #11430, #32465 ) ;
#25305=EDGE_CURVE ( 'NONE', #31468, #23190, #15515, .T. ) ;
#25316=CIRCLE ( 'NONE', #27024, 34.41491905851385269 ) ;
#25317=EDGE_LOOP ( 'NONE', ( #6466, #7848, #24458, #9031 ) ) ;
#25326=ORIENTED_EDGE ( 'NONE', *, *, #32034, .T. ) ;
#25327=ORIENTED_EDGE ( 'NONE', *, *, #33828, .T. ) ;
#25332=CYLINDRICAL_SURFACE ( 'NONE', #19376, 2.524999999999999467 ) ;
#25334=ORIENTED_EDGE ( 'NONE', *, *, #5437, .F. ) ;
#25336=LINE ( 'NONE', #12009, #19860 ) ;
#25345=EDGE_CURVE ( 'NONE', #19221, #22410, #34277, .T. ) ;
#25348=EDGE_CURVE ( 'NONE', #34651, #34913, #26782, .T. ) ;
#25349=CARTESIAN_POINT ( 'NONE',  ( 0.000000000000000000, 20.79173593595294633, -22.27454621808743340 ) ) ;
#25353=EDGE_LOOP ( 'NONE', ( #6431, #812, #6247, #24213, #7032, #3522, #12107 ) ) ;
#25359=B_SPLINE_CURVE_WITH_KNOTS ( 'NONE', 3,
 ( #15867, #2662, #9975, #31674 ),
 .UNSPECIFIED., .F., .F.,
 ( 4, 4 ),
 ( 2.250995564674948756E-07, 0.0006879610227481868607 ),
 .UNSPECIFIED. ) ;
#25363=ORIENTED_EDGE ( 'NONE', *, *, #20498, .F. ) ;
#25368=CARTESIAN_POINT ( 'NONE',  ( 1.749999999999999778, 21.72796464722008380, 26.68861566460903489 ) ) ;
#25369=DIRECTION ( 'NONE',  ( 0.000000000000000000, 0.000000000000000000, 1.000000000000000000 ) ) ;
#25371=ORIENTED_EDGE ( 'NONE', *, *, #1250, .F. ) ;
#25372=DIRECTION ( 'NONE',  ( 0.000000000000000000, 0.000000000000000000, 1.000000000000000000 ) ) ;
#25391=ADVANCED_FACE ( 'NONE', ( #89 ), #21455, .F. ) ;
#25400=ORIENTED_EDGE ( 'NONE', *, *, #20487, .F. ) ;
#25402=CIRCLE ( 'NONE', #17493, 30.47050528711512030 ) ;
#25403=LINE ( 'NONE', #4027, #31795 ) ;
#25414=B_SPLINE_CURVE_WITH_KNOTS ( 'NONE', 3,
 ( #34480, #28962, #31627, #23799, #34300, #34658 ),
 .UNSPECIFIED., .F., .F.,
 ( 4, 2, 4 ),
 ( 4.404817051637942833E-07, 0.001874269637237883143, 0.003748098792770602258 ),
 .UNSPECIFIED. ) ;
#25427=CARTESIAN_POINT ( 'NONE',  ( 0.1859802676143585964, 30.43784769162285997, -10.75394592869476895 ) ) ;
#25428=ORIENTED_EDGE ( 'NONE', *, *, #1294, .T. ) ;
#25435=DIRECTION ( 'NONE',  ( -1.000000000000000000, 0.000000000000000000, 0.000000000000000000 ) ) ;
#25441=ORIENTED_EDGE ( 'NONE', *, *, #4199, .F. ) ;
#25442=AXIS2_PLACEMENT_3D ( 'NONE', #32598, #21748, #403 ) ;
#25444=ORIENTED_EDGE ( 'NONE', *, *, #16448, .F. ) ;
#25446=ORIENTED_EDGE ( 'NONE', *, *, #28202, .F. ) ;
#25447=ORIENTED_EDGE ( 'NONE', *, *, #5715, .F. ) ;
#25450=DIRECTION ( 'NONE',  ( -1.000000000000000000, -0.000000000000000000, -0.000000000000000000 ) ) ;
#25454=EDGE_CURVE ( 'NONE', #32497, #797, #18739, .T. ) ;
#25455=EDGE_CURVE ( 'NONE', #30400, #14739, #34281, .T. ) ;
#25457=CARTESIAN_POINT ( 'NONE',  ( 2.765921099433441999, -17.95514392185434360, 25.38201125280350468 ) ) ;
#25458=CYLINDRICAL_SURFACE ( 'NONE', #6139, 16.19999999999999218 ) ;
#25459=AXIS2_PLACEMENT_3D ( 'NONE', #2379, #24086, #21436 ) ;
#25471=CIRCLE ( 'NONE', #8421, 30.47050528711512030 ) ;
#25483=B_SPLINE_CURVE_WITH_KNOTS ( 'NONE', 3,
 ( #28262, #3689, #33057, #1206 ),
 .UNSPECIFIED., .F., .F.,
 ( 4, 4 ),
 ( 4.077050493238060077E-07, 0.0006881451559005274379 ),
 .UNSPECIFIED. ) ;
#25485=CARTESIAN_POINT ( 'NONE',  ( 0.000000000000000000, -29.91351748324100512, -5.799410679710955030 ) ) ;
#25487=VECTOR ( 'NONE', #33304, 1000.000000000000000 ) ;
#25493=ORIENTED_EDGE ( 'NONE', *, *, #15005, .F. ) ;
#25497=EDGE_CURVE ( 'NONE', #28134, #34702, #31387, .T. ) ;
#25501=DIRECTION ( 'NONE',  ( 0.000000000000000000, 0.000000000000000000, 1.000000000000000000 ) ) ;
#25510=EDGE_LOOP ( 'NONE', ( #5705, #4680, #24096, #12139 ) ) ;
#25515=ORIENTED_EDGE ( 'NONE', *, *, #25550, .T. ) ;
#25520=DIRECTION ( 'NONE',  ( 0.000000000000000000, 0.000000000000000000, 1.000000000000000000 ) ) ;
#25529=ORIENTED_EDGE ( 'NONE', *, *, #4581, .T. ) ;
#25538=CARTESIAN_POINT ( 'NONE',  ( 1.040000000000000258, -18.66807150955433769, 28.91175816027496381 ) ) ;
#25545=CARTESIAN_POINT ( 'NONE',  ( 0.000000000000000000, 11.30192140231274500, -28.29696565125059493 ) ) ;
#25550=EDGE_CURVE ( 'NONE', #4601, #14930, #22511, .T. ) ;
#25564=ORIENTED_EDGE ( 'NONE', *, *, #2127, .T. ) ;
#25569=FACE_OUTER_BOUND ( 'NONE', #8357, .T. ) ;
#25578=B_SPLINE_CURVE_WITH_KNOTS ( 'NONE', 3,
 ( #13315, #28794, #34486, #4741 ),
 .UNSPECIFIED., .F., .F.,
 ( 4, 4 ),
 ( 2.013258991796062060E-07, 0.0006879370499043869483 ),
 .UNSPECIFIED. ) ;
#25582=CARTESIAN_POINT ( 'NONE',  ( 2.765921099435497243, 28.29688452313399338, 12.88099432405614309 ) ) ;
#25584=VERTEX_POINT ( 'NONE', #30523 ) ;
#25594=ADVANCED_FACE ( 'NONE', ( #26394 ), #29175, .T. ) ;
#25600=CARTESIAN_POINT ( 'NONE',  ( 0.07094832525803791701, 29.95509811880046058, -10.35390711157451449 ) ) ;
#25617=EDGE_LOOP ( 'NONE', ( #22162, #22082, #19603, #10401, #27279, #18200 ) ) ;
#25623=CARTESIAN_POINT ( 'NONE',  ( -10.00000000000000000, 0.000000000000000000, 0.000000000000000000 ) ) ;
#25630=DIRECTION ( 'NONE',  ( 0.000000000000000000, 0.000000000000000000, 1.000000000000000000 ) ) ;
#25636=CARTESIAN_POINT ( 'NONE',  ( 0.000000000000000000, 0.000000000000000000, 0.000000000000000000 ) ) ;
#25650=DIRECTION ( 'NONE',  ( -1.000000000000000000, -0.000000000000000000, 0.000000000000000000 ) ) ;
#25653=CARTESIAN_POINT ( 'NONE',  ( 1.040000000000001146, 6.183021911002323456, -33.85493898757056286 ) ) ;
#25654=DIRECTION ( 'NONE',  ( 0.000000000000000000, 0.000000000000000000, 1.000000000000000000 ) ) ;
#25656=DIRECTION ( 'NONE',  ( -1.000000000000000000, -0.000000000000000000, -0.000000000000000000 ) ) ;
#25669=LINE ( 'NONE', #17683, #1700 ) ;
#25696=CARTESIAN_POINT ( 'NONE',  ( 1.395000000000002238, 31.89769921722987434, 12.91988538846969803 ) ) ;
#25705=CARTESIAN_POINT ( 'NONE',  ( 2.765921099433441555, 11.80989368511502846, -28.76039115933972923 ) ) ;
#25706=EDGE_CURVE ( 'NONE', #30641, #14675, #12144, .T. ) ;
#25707=EDGE_CURVE ( 'NONE', #18645, #30046, #28596, .T. ) ;
#25710=CARTESIAN_POINT ( 'NONE',  ( 0.02407890056655651728, 11.80989368511502846, -28.76039115933972923 ) ) ;
#25712=VERTEX_POINT ( 'NONE', #16439 ) ;
#25713=VECTOR ( 'NONE', #17600, 1000.000000000000000 ) ;
#25725=CARTESIAN_POINT ( 'NONE',  ( 0.7561992258976059089, 33.57713782924224688, -4.776499238012502424 ) ) ;
#25735=VERTEX_POINT ( 'NONE', #2879 ) ;
#25736=B_SPLINE_CURVE_WITH_KNOTS ( 'NONE', 3,
 ( #27743, #25059, #32730, #11563 ),
 .UNSPECIFIED., .F., .F.,
 ( 4, 4 ),
 ( 2.075676022607250875E-07, 0.0006879433439099810017 ),
 .UNSPECIFIED. ) ;
#25762=CIRCLE ( 'NONE', #1877, 30.47050528711511674 ) ;
#25764=FACE_OUTER_BOUND ( 'NONE', #4159, .T. ) ;
#25768=ORIENTED_EDGE ( 'NONE', *, *, #19165, .F. ) ;
#25769=CARTESIAN_POINT ( 'NONE',  ( 0.07098927069927472855, 26.43944202223353201, 17.47857661787128691 ) ) ;
#25774=DIRECTION ( 'NONE',  ( 0.000000000000000000, 0.000000000000000000, 1.000000000000000000 ) ) ;
#25780=EDGE_CURVE ( 'NONE', #34395, #24520, #4708, .T. ) ;
#25799=B_SPLINE_CURVE_WITH_KNOTS ( 'NONE', 3,
 ( #4645, #24230, #21041, #29233, #20868, #2340 ),
 .UNSPECIFIED., .F., .F.,
 ( 4, 2, 4 ),
 ( 2.185847997383155607E-07, 0.001873416899431755130, 0.003746615214063771931 ),
 .UNSPECIFIED. ) ;
#25806=VERTEX_POINT ( 'NONE', #19809 ) ;
#25807=DIRECTION ( 'NONE',  ( -1.000000000000000000, -0.000000000000000000, -0.000000000000000000 ) ) ;
#25813=ORIENTED_EDGE ( 'NONE', *, *, #1696, .F. ) ;
#25816=DIRECTION ( 'NONE',  ( 0.000000000000000000, 0.000000000000000000, 1.000000000000000000 ) ) ;
#25820=ORIENTED_EDGE ( 'NONE', *, *, #8623, .T. ) ;
#25821=CARTESIAN_POINT ( 'NONE',  ( 2.765921099433442887, -21.56796757982795043, -22.39322359481629476 ) ) ;
#25822=ORIENTED_EDGE ( 'NONE', *, *, #17443, .F. ) ;
#25824=CARTESIAN_POINT ( 'NONE',  ( 0.000000000000000000, 2.005524111408653720, -29.35189292423236296 ) ) ;
#25826=CARTESIAN_POINT ( 'NONE',  ( 2.789999999999999147, -13.59935610937951900, -28.90010281771846223 ) ) ;
#25833=DIRECTION ( 'NONE',  ( 0.000000000000000000, 0.000000000000000000, 1.000000000000000000 ) ) ;
#25841=EDGE_CURVE ( 'NONE', #9222, #17861, #12741, .T. ) ;
#25844=( LENGTH_UNIT ( ) NAMED_UNIT ( * ) SI_UNIT ( .MILLI., .METRE. ) );
#25845=ORIENTED_EDGE ( 'NONE', *, *, #28168, .T. ) ;
#25856=DIRECTION ( 'NONE',  ( -1.000000000000000000, 0.000000000000000000, -0.000000000000000000 ) ) ;
#25858=B_SPLINE_CURVE_WITH_KNOTS ( 'NONE', 3,
 ( #11728, #30405, #27552, #22045, #9045, #33061 ),
 .UNSPECIFIED., .F., .F.,
 ( 4, 2, 4 ),
 ( 4.404817020086782935E-07, 0.001874269619297521056, 0.003748098756893033113 ),
 .UNSPECIFIED. ) ;
#25868=EDGE_CURVE ( 'NONE', #17311, #21561, #8690, .T. ) ;
#25885=CARTESIAN_POINT ( 'NONE',  ( 2.789999999999999147, -20.35927063852789232, -24.61013060777193218 ) ) ;
#25886=DIRECTION ( 'NONE',  ( -1.000000000000000000, 0.000000000000000000, 0.000000000000000000 ) ) ;
#25887=CARTESIAN_POINT ( 'NONE',  ( 8.000000000000000000, 0.000000000000000000, 0.000000000000000000 ) ) ;
#25900=DIRECTION ( 'NONE',  ( -1.000000000000000000, -0.000000000000000000, -0.000000000000000000 ) ) ;
#25907=CARTESIAN_POINT ( 'NONE',  ( 2.765921099433442887, -21.56796757982795043, -22.39322359481629476 ) ) ;
#25908=DIRECTION ( 'NONE',  ( -1.000000000000000000, 0.000000000000000000, -0.000000000000000000 ) ) ;
#25912=CARTESIAN_POINT ( 'NONE',  ( 2.789999999999999147, -31.68806325674609781, 4.003133335385473224 ) ) ;
#25914=ADVANCED_FACE ( 'NONE', ( #14818 ), #22471, .F. ) ;
#25921=CARTESIAN_POINT ( 'NONE',  ( 1.749999999999999778, -10.89151784028265624, -32.64600270996228204 ) ) ;
#25930=CARTESIAN_POINT ( 'NONE',  ( 0.000000000000000000, 23.53611639059712601, 19.35207786518996897 ) ) ;
#25932=ORIENTED_EDGE ( 'NONE', *, *, #32657, .F. ) ;
#25935=B_SPLINE_CURVE_WITH_KNOTS ( 'NONE', 3,
 ( #24850, #22370, #22731, #25201 ),
 .UNSPECIFIED., .F., .F.,
 ( 4, 4 ),
 ( 0.005298458409503515980, 0.005985325590332025991 ),
 .UNSPECIFIED. ) ;
#25940=EDGE_LOOP ( 'NONE', ( #33557, #29972, #27766, #1384 ) ) ;
#25948=EDGE_LOOP ( 'NONE', ( #3744, #31669, #18138, #20345 ) ) ;
#25949=FACE_OUTER_BOUND ( 'NONE', #9386, .T. ) ;
#25953=EDGE_CURVE ( 'NONE', #23746, #26863, #11028, .T. ) ;
#25963=VECTOR ( 'NONE', #24527, 1000.000000000000000 ) ;
#25964=DIRECTION ( 'NONE',  ( -1.000000000000000000, 0.000000000000000000, 0.000000000000000000 ) ) ;
#25967=CARTESIAN_POINT ( 'NONE',  ( 0.7564103347627352258, -17.72288109958190816, -28.91649664306142142 ) ) ;
#25968=CARTESIAN_POINT ( 'NONE',  ( 0.000000000000000000, -25.77598557799263901, 16.24962337825793313 ) ) ;
#25985=EDGE_CURVE ( 'NONE', #12821, #24969, #28847, .T. ) ;
#25989=VERTEX_POINT ( 'NONE', #4097 ) ;
#26005=CARTESIAN_POINT ( 'NONE',  ( 2.788639899212288054, -26.04763539363528579, -16.24881338200996694 ) ) ;
#26031=ORIENTED_EDGE ( 'NONE', *, *, #5916, .F. ) ;
#26033=CARTESIAN_POINT ( 'NONE',  ( -5.210000000000000853, 0.000000000000000000, 0.000000000000000000 ) ) ;
#26040=TOROIDAL_SURFACE ( 'NONE', #6109, 30.47050528711512030, 8.000000000000000000 ) ;
#26057=DIRECTION ( 'NONE',  ( 0.000000000000000000, 0.000000000000000000, 1.000000000000000000 ) ) ;
#26059=AXIS2_PLACEMENT_3D ( 'NONE', #29359, #13511, #8338 ) ;
#26061=AXIS2_PLACEMENT_3D ( 'NONE', #15493, #15143, #7632 ) ;
#26063=B_SPLINE_CURVE_WITH_KNOTS ( 'NONE', 3,
 ( #34889, #10502, #16025, #11695, #5137, #21695 ),
 .UNSPECIFIED., .F., .F.,
 ( 4, 2, 4 ),
 ( 1.978042196652697246E-07, 0.001873396096185926674, 0.003746594388152188135 ),
 .UNSPECIFIED. ) ;
#26064=ORIENTED_EDGE ( 'NONE', *, *, #29248, .T. ) ;
#26067=DIRECTION ( 'NONE',  ( 0.000000000000000000, 0.000000000000000000, 1.000000000000000000 ) ) ;
#26069=ORIENTED_EDGE ( 'NONE', *, *, #1253, .T. ) ;
#26075=ORIENTED_EDGE ( 'NONE', *, *, #34321, .T. ) ;
#26077=CARTESIAN_POINT ( 'NONE',  ( 2.789999999999999147, 20.99477179376858871, -22.93149026599722617 ) ) ;
#26089=CARTESIAN_POINT ( 'NONE',  ( 1.040000000000001590, 34.10861917999616111, 4.581348211832199091 ) ) ;
#26090=DIRECTION ( 'NONE',  ( 0.000000000000000000, 0.000000000000000000, 1.000000000000000000 ) ) ;
#26096=CARTESIAN_POINT ( 'NONE',  ( 1.039999999999999369, -18.21166265554768060, -29.20140402659759360 ) ) ;
#26097=CARTESIAN_POINT ( 'NONE',  ( 0.02407890056655868569, 24.20451283648829133, 19.51346322004938827 ) ) ;
#26104=VERTEX_POINT ( 'NONE', #20494 ) ;
#26105=AXIS2_PLACEMENT_3D ( 'NONE', #29226, #17733, #15715 ) ;
#26106=ADVANCED_FACE ( 'NONE', ( #29205 ), #14991, .F. ) ;
#26122=CARTESIAN_POINT ( 'NONE',  ( 0.000000000000000000, 30.40449935640659973, -2.004522720844279959 ) ) ;
#26125=ADVANCED_FACE ( 'NONE', ( #32037 ), #13370, .T. ) ;
#26126=CARTESIAN_POINT ( 'NONE',  ( 0.000000000000000000, 23.28319895603611300, -21.86437915510192909 ) ) ;
#26129=CARTESIAN_POINT ( 'NONE',  ( 2.765921099433444663, 29.44518845714764765, 9.980709654879525772 ) ) ;
#26135=CARTESIAN_POINT ( 'NONE',  ( 2.789999999999999147, 3.909681563762101852, -30.21863799912378923 ) ) ;
#26141=EDGE_CURVE ( 'NONE', #21605, #14930, #10701, .T. ) ;
#26145=ORIENTED_EDGE ( 'NONE', *, *, #1127, .F. ) ;
#26161=VERTEX_POINT ( 'NONE', #3015 ) ;
#26165=ADVANCED_FACE ( 'NONE', ( #18887 ), #18718, .T. ) ;
#26173=DIRECTION ( 'NONE',  ( 0.000000000000000000, 0.000000000000000000, 1.000000000000000000 ) ) ;
#26180=EDGE_LOOP ( 'NONE', ( #24001, #34305, #17770, #18781, #8055, #1173, #2221, #78, #31528, #25400, #15783, #4686, #13550, #20579, #22533, #8299, #33078, #8845, #33752, #207, #4019, #34568, #8324, #25493, #20363, #8610, #4644, #33159, #7321, #7971, #23535, #23711, #20219, #27768, #5642, #22418, #15, #11319, #4862, #3265, #18378, #597, #25564, #24790, #28695, #31384, #19249, #17695, #21977, #8138, #18948, #1854, #31801, #6234, #20977, #8770, #26581 ) ) ;
#26183=DIRECTION ( 'NONE',  ( 0.000000000000000000, 0.000000000000000000, 1.000000000000000000 ) ) ;
#26198=CIRCLE ( 'NONE', #19972, 2.525000000000000799 ) ;
#26200=B_SPLINE_CURVE_WITH_KNOTS ( 'NONE', 3,
 ( #15344, #32041, #1626, #15518 ),
 .UNSPECIFIED., .F., .F.,
 ( 4, 4 ),
 ( 0.005679541198217082261, 0.005985272568144436693 ),
 .UNSPECIFIED. ) ;
#26201=LINE ( 'NONE', #1821, #22137 ) ;
#26205=CIRCLE ( 'NONE', #17703, 34.41491905851385269 ) ;
#26211=CARTESIAN_POINT ( 'NONE',  ( 0.02407890056655695096, -26.45933846664205902, 16.32596387352436551 ) ) ;
#26220=EDGE_LOOP ( 'NONE', ( #12338, #14666, #34572, #17167, #7531, #15526, #30679, #2862 ) ) ;
#26224=EDGE_CURVE ( 'NONE', #16525, #19620, #5085, .T. ) ;
#26231=ORIENTED_EDGE ( 'NONE', *, *, #22437, .T. ) ;
#26235=FACE_OUTER_BOUND ( 'NONE', #12170, .T. ) ;
#26237=EDGE_CURVE ( 'NONE', #3245, #19221, #21173, .T. ) ;
#26239=DIRECTION ( 'NONE',  ( 0.000000000000000000, 0.000000000000000000, 1.000000000000000000 ) ) ;
#26247=AXIS2_PLACEMENT_3D ( 'NONE', #24214, #32396, #16232 ) ;
#26251=DIRECTION ( 'NONE',  ( -1.000000000000000000, -0.000000000000000000, -0.000000000000000000 ) ) ;
#26256=ORIENTED_EDGE ( 'NONE', *, *, #8248, .T. ) ;
#26258=DIRECTION ( 'NONE',  ( -1.000000000000000000, -0.000000000000000000, 0.000000000000000000 ) ) ;
#26263=ORIENTED_EDGE ( 'NONE', *, *, #9845, .T. ) ;
#26267=B_SPLINE_CURVE_WITH_KNOTS ( 'NONE', 3,
 ( #4682, #29081, #10759, #16107 ),
 .UNSPECIFIED., .F., .F.,
 ( 4, 4 ),
 ( 1.991136383990134541E-07, 0.0003071994222346450588 ),
 .UNSPECIFIED. ) ;
#26273=CARTESIAN_POINT ( 'NONE',  ( -6.195103562623470712E-16, -30.61407293071429336, 1.706449706642247932 ) ) ;
#26275=EDGE_CURVE ( 'NONE', #27741, #7441, #27583, .T. ) ;
#26283=CARTESIAN_POINT ( 'NONE',  ( 1.039999999999999813, -24.90160365674851661, -23.75493189058366994 ) ) ;
#26285=CARTESIAN_POINT ( 'NONE',  ( 1.749999999999999778, -33.39989884085085237, -8.296590337300626672 ) ) ;
#26289=ORIENTED_EDGE ( 'NONE', *, *, #31304, .F. ) ;
#26291=CARTESIAN_POINT ( 'NONE',  ( 2.789999999999999147, 23.53611639059738536, -19.35207786518964213 ) ) ;
#26299=DIRECTION ( 'NONE',  ( 0.000000000000000000, 0.8443279255020087470, 0.5358267949790064266 ) ) ;
#26307=ADVANCED_FACE ( 'NONE', ( #713 ), #28115, .T. ) ;
#26318=AXIS2_PLACEMENT_3D ( 'NONE', #29736, #10165, #32567 ) ;
#26330=CARTESIAN_POINT ( 'NONE',  ( 1.749999999999999778, 0.000000000000000000, 0.000000000000000000 ) ) ;
#26348=CARTESIAN_POINT ( 'NONE',  ( 50.00050000000000239, 0.000000000000000000, 0.000000000000000000 ) ) ;
#26351=DIRECTION ( 'NONE',  ( -1.000000000000000000, -0.000000000000000000, 0.000000000000000000 ) ) ;
#26356=EDGE_CURVE ( 'NONE', #32541, #8838, #16750, .T. ) ;
#26365=TOROIDAL_SURFACE ( 'NONE', #9887, 30.47050528711511674, 8.000000000000000000 ) ;
#26379=CARTESIAN_POINT ( 'NONE',  ( -8.203566206536489625E-14, 4.061185680397187525, 30.39260865248091292 ) ) ;
#26392=DIRECTION ( 'NONE',  ( 1.000000000000000000, 0.000000000000000000, 0.000000000000000000 ) ) ;
#26394=FACE_OUTER_BOUND ( 'NONE', #21776, .T. ) ;
#26400=VERTEX_POINT ( 'NONE', #26135 ) ;
#26403=CARTESIAN_POINT ( 'NONE',  ( 0.006871052814942861346, 30.38119646769583682, 5.469045072945091235 ) ) ;
#26406=ORIENTED_EDGE ( 'NONE', *, *, #16343, .F. ) ;
#26407=CIRCLE ( 'NONE', #839, 34.41491905851385269 ) ;
#26408=VERTEX_POINT ( 'NONE', #7429 ) ;
#26414=VERTEX_POINT ( 'NONE', #29072 ) ;
#26420=CIRCLE ( 'NONE', #13379, 2.525000000000000799 ) ;
#26430=DIRECTION ( 'NONE',  ( -1.000000000000000000, -0.000000000000000000, -0.000000000000000000 ) ) ;
#26431=VERTEX_POINT ( 'NONE', #28634 ) ;
#26435=CARTESIAN_POINT ( 'NONE',  ( 2.033800797852382658, -17.72251720152513244, -28.91628452940461713 ) ) ;
#26438=ORIENTED_EDGE ( 'NONE', *, *, #14271, .T. ) ;
#26442=ORIENTED_EDGE ( 'NONE', *, *, #17027, .F. ) ;
#26443=DIRECTION ( 'NONE',  ( -1.000000000000000000, -0.000000000000000000, 0.000000000000000000 ) ) ;
#26446=CARTESIAN_POINT ( 'NONE',  ( 0.006871051457199655287, -11.06504178053304699, 28.81826507853126174 ) ) ;
#26451=DIRECTION ( 'NONE',  ( 0.000000000000000000, 0.000000000000000000, 1.000000000000000000 ) ) ;
#26452=CLOSED_SHELL ( 'NONE', ( #30065, #18374, #28994, #26106, #12989, #3178, #12503, #5164, #29546, #3725, #21452, #15002, #30685, #9146, #9148, #26543, #16895, #5378, #34389, #278, #28056, #4768, #17789, #20823, #32409, #12027, #28730, #25594, #30894, #33637, #34429, #8789, #27069, #31951, #27832, #6673, #12947, #3892, #23335, #3559, #24695, #14269, #12, #29406, #26125, #26886, #33887, #20258, #21343, #5552, #23828, #14122, #6707, #13473, #23853, #15398, #18771, #34969, #9789, #16767, #6722, #18105, #6281, #28418, #17636, #18582, #11679, #27445, #2913, #14132, #8744, #23111, #33476, #6807, #2368, #10679, #24942, #32143, #7360, #34082, #13876, #30026, #3074, #112, #14313, #12860, #32482, #11250, #1207, #22875, #34379, #19757, #32931, #7842, #9357, #10462, #10461, #13946, #7749, #33100, #19173, #26732, #25391, #27354, #27162, #7010, #4926, #8033, #11442, #26307, #4805, #22460, #13633, #32083, #29029, #23494, #21162, #5018, #8986, #29163, #25130, #16055, #20185, #24042, #11452, #30474, #25914, #21715, #26165, #23043, #28606, #14396, #30772, #3596, #21950, #7175, #3668, #13347, #26991, #14119, #13260, #27751, #5068, #32044, #34023, #30251, #25212, #23577, #12112, #28006, #1057, #3496, #3808, #34360, #1633, #12750, #11827, #14374, #13731, #6132, #2807, #6613, #18232, #8061, #23631, #21324, #602, #24051 ) ) ;
#26461=DIRECTION ( 'NONE',  ( -1.000000000000000000, 0.000000000000000000, 0.000000000000000000 ) ) ;
#26462=ORIENTED_EDGE ( 'NONE', *, *, #8949, .T. ) ;
#26465=CARTESIAN_POINT ( 'NONE',  ( 0.1835379745812393826, 26.80070150627937053, 17.97639020990316183 ) ) ;
#26467=EDGE_CURVE ( 'NONE', #949, #10663, #31748, .T. ) ;
#26469=DIRECTION ( 'NONE',  ( -1.000000000000000000, -0.000000000000000000, -0.000000000000000000 ) ) ;
#26473=CARTESIAN_POINT ( 'NONE',  ( 2.789999999999999147, 9.869977788041397915, -30.37666815053925973 ) ) ;
#26474=ORIENTED_EDGE ( 'NONE', *, *, #20066, .F. ) ;
#26476=B_SPLINE_CURVE_WITH_KNOTS ( 'NONE', 3,
 ( #20160, #6607, #9474, #20332 ),
 .UNSPECIFIED., .F., .F.,
 ( 4, 4 ),
 ( 1.989389905266797354E-07, 0.002009632881715329999 ),
 .UNSPECIFIED. ) ;
#26483=EDGE_CURVE ( 'NONE', #27613, #11423, #14388, .T. ) ;
#26499=ORIENTED_EDGE ( 'NONE', *, *, #968, .F. ) ;
#26501=CARTESIAN_POINT ( 'NONE',  ( 1.040000000000002256, 27.68252950111368094, -20.44661865013457813 ) ) ;
#26512=VERTEX_POINT ( 'NONE', #22955 ) ;
#26513=CARTESIAN_POINT ( 'NONE',  ( 2.789999999999999147, 0.000000000000000000, 0.000000000000000000 ) ) ;
#26516=FACE_OUTER_BOUND ( 'NONE', #20, .T. ) ;
#26517=CARTESIAN_POINT ( 'NONE',  ( 2.719051659807903754, 31.23788557484581574, -5.357780584450596351 ) ) ;
#26518=ORIENTED_EDGE ( 'NONE', *, *, #12190, .F. ) ;
#26524=FACE_OUTER_BOUND ( 'NONE', #26180, .T. ) ;
#26531=CYLINDRICAL_SURFACE ( 'NONE', #17335, 16.19999999999999574 ) ;
#26532=CARTESIAN_POINT ( 'NONE',  ( 2.789999999999999147, 17.11426446101199161, 26.96776559937732642 ) ) ;
#26543=ADVANCED_FACE ( 'NONE', ( #26663 ), #28081, .T. ) ;
#26547=ORIENTED_EDGE ( 'NONE', *, *, #28078, .T. ) ;
#26548=CARTESIAN_POINT ( 'NONE',  ( -5.588430218784975857E-16, 20.82898695786893484, 22.50081875905981121 ) ) ;
#26554=ORIENTED_EDGE ( 'NONE', *, *, #21684, .T. ) ;
#26557=CARTESIAN_POINT ( 'NONE',  ( 0.5248941326870452118, 31.31301644755022551, 11.56311898902757385 ) ) ;
#26572=CARTESIAN_POINT ( 'NONE',  ( 2.033589657429622388, 27.12319051591943619, -20.36165095825642979 ) ) ;
#26576=DIRECTION ( 'NONE',  ( 0.000000000000000000, 0.000000000000000000, -1.000000000000000000 ) ) ;
#26579=CARTESIAN_POINT ( 'NONE',  ( 0.000000000000000000, 0.000000000000000000, 0.000000000000000000 ) ) ;
#26581=ORIENTED_EDGE ( 'NONE', *, *, #163, .T. ) ;
#26583=VECTOR ( 'NONE', #2285, 1000.000000000000000 ) ;
#26587=CYLINDRICAL_SURFACE ( 'NONE', #19083, 16.19999999999999574 ) ;
#26591=AXIS2_PLACEMENT_3D ( 'NONE', #8257, #26598, #21615 ) ;
#26597=DIRECTION ( 'NONE',  ( -1.000000000000000000, 0.000000000000000000, 0.000000000000000000 ) ) ;
#26598=DIRECTION ( 'NONE',  ( 1.000000000000000000, 0.000000000000000000, 0.000000000000000000 ) ) ;
#26602=VERTEX_POINT ( 'NONE', #32517 ) ;
#26605=DIRECTION ( 'NONE',  ( 0.000000000000000000, 0.000000000000000000, 1.000000000000000000 ) ) ;
#26609=CARTESIAN_POINT ( 'NONE',  ( 2.606462082920441681, -16.25808774470336715, -27.87656317279346041 ) ) ;
#26611=CARTESIAN_POINT ( 'NONE',  ( 2.789999999999999147, 0.000000000000000000, 0.000000000000000000 ) ) ;
#26630=VECTOR ( 'NONE', #5005, 1000.000000000000000 ) ;
#26634=EDGE_CURVE ( 'NONE', #13451, #34913, #6121, .T. ) ;
#26646=CYLINDRICAL_SURFACE ( 'NONE', #32127, 34.41491905851385269 ) ;
#26647=CARTESIAN_POINT ( 'NONE',  ( 1.039999999999999813, 21.72796464722045684, -26.68861566460872226 ) ) ;
#26663=FACE_OUTER_BOUND ( 'NONE', #31581, .T. ) ;
#26670=EDGE_CURVE ( 'NONE', #6869, #32274, #8176, .T. ) ;
#26677=CARTESIAN_POINT ( 'NONE',  ( 1.040000000000001590, 34.10861917999616111, 4.581348211832199091 ) ) ;
#26682=EDGE_CURVE ( 'NONE', #31475, #21040, #16526, .T. ) ;
#26684=B_SPLINE_CURVE_WITH_KNOTS ( 'NONE', 3,
 ( #19881, #11511, #30723, #33022 ),
 .UNSPECIFIED., .F., .F.,
 ( 4, 4 ),
 ( 0.005298347429621244956, 0.005985216133920617451 ),
 .UNSPECIFIED. ) ;
#26687=EDGE_CURVE ( 'NONE', #31871, #5830, #31056, .T. ) ;
#26690=ORIENTED_EDGE ( 'NONE', *, *, #26993, .T. ) ;
#26691=ORIENTED_EDGE ( 'NONE', *, *, #22789, .F. ) ;
#26695=CARTESIAN_POINT ( 'NONE',  ( 2.765921099433442443, 30.61125888652969707, -5.439165181698684570 ) ) ;
#26703=CARTESIAN_POINT ( 'NONE',  ( 2.765921099433442887, -26.45933846664205902, 16.32596387352436551 ) ) ;
#26707=CARTESIAN_POINT ( 'NONE',  ( 0.006892465017757970838, -0.3207854480229822558, 30.86813304286355475 ) ) ;
#26716=CIRCLE ( 'NONE', #11384, 34.41491905851385269 ) ;
#26728=CARTESIAN_POINT ( 'NONE',  ( 0.02407890056655608360, 4.286445725888036407, 30.79383171238946204 ) ) ;
#26732=ADVANCED_FACE ( 'NONE', ( #14871 ), #6294, .T. ) ;
#26739=DIRECTION ( 'NONE',  ( -1.000000000000000000, -0.000000000000000000, -0.000000000000000000 ) ) ;
#26744=CARTESIAN_POINT ( 'NONE',  ( 2.789999999999999147, 23.28319895603611300, -19.33937915510192695 ) ) ;
#26748=CARTESIAN_POINT ( 'NONE',  ( 1.749999999999999778, 14.40815186467820475, -31.25366880301303496 ) ) ;
#26764=ORIENTED_EDGE ( 'NONE', *, *, #31700, .T. ) ;
#26782=B_SPLINE_CURVE_WITH_KNOTS ( 'NONE', 3,
 ( #3281, #26966, #20165, #8450, #3103, #24984 ),
 .UNSPECIFIED., .F., .F.,
 ( 4, 2, 4 ),
 ( 4.404817001606571728E-07, 0.001874269605587681586, 0.003748098729475202520 ),
 .UNSPECIFIED. ) ;
#26799=ORIENTED_EDGE ( 'NONE', *, *, #11715, .F. ) ;
#26812=LINE ( 'NONE', #7937, #8189 ) ;
#26815=ORIENTED_EDGE ( 'NONE', *, *, #31322, .F. ) ;
#26823=CARTESIAN_POINT ( 'NONE',  ( 2.789999999999999147, 0.000000000000000000, 0.000000000000000000 ) ) ;
#26829=CARTESIAN_POINT ( 'NONE',  ( 0.7561992110385835630, 21.20694131899082535, -26.46705060818936062 ) ) ;
#26837=CARTESIAN_POINT ( 'NONE',  ( 1.749999999999999778, 22.14447232807506438, 26.34405054495565679 ) ) ;
#26849=VERTEX_POINT ( 'NONE', #24592 ) ;
#26857=AXIS2_PLACEMENT_3D ( 'NONE', #24855, #492, #11350 ) ;
#26860=DIRECTION ( 'NONE',  ( -1.000000000000000000, 0.000000000000000000, 0.000000000000000000 ) ) ;
#26863=VERTEX_POINT ( 'NONE', #32957 ) ;
#26867=EDGE_CURVE ( 'NONE', #2667, #31399, #34352, .T. ) ;
#26886=ADVANCED_FACE ( 'NONE', ( #21759 ), #5383, .T. ) ;
#26892=VECTOR ( 'NONE', #28379, 1000.000000000000000 ) ;
#26899=FACE_OUTER_BOUND ( 'NONE', #1581, .T. ) ;
#26900=AXIS2_PLACEMENT_3D ( 'NONE', #2753, #29817, #8802 ) ;
#26904=CARTESIAN_POINT ( 'NONE',  ( 0.006871051546331624453, 7.365904273040736250, -29.97784191786578134 ) ) ;
#26909=CARTESIAN_POINT ( 'NONE',  ( 0.000000000000000000, -13.59935610937992401, 28.90010281771827039 ) ) ;
#26919=DIRECTION ( 'NONE',  ( 0.000000000000000000, 0.000000000000000000, 1.000000000000000000 ) ) ;
#26924=CARTESIAN_POINT ( 'NONE',  ( -5.210000000000000853, 0.000000000000000000, 0.000000000000000000 ) ) ;
#26925=ORIENTED_EDGE ( 'NONE', *, *, #24005, .F. ) ;
#26930=B_SPLINE_CURVE_WITH_KNOTS ( 'NONE', 3,
 ( #29517, #23979, #34678, #13492 ),
 .UNSPECIFIED., .F., .F.,
 ( 4, 4 ),
 ( 2.128468106751623115E-07, 0.0006879486673519059079 ),
 .UNSPECIFIED. ) ;
#26949=CARTESIAN_POINT ( 'NONE',  ( 0.7561992015540950351, -29.97203090897408018, -15.87187733271013990 ) ) ;
#26952=CARTESIAN_POINT ( 'NONE',  ( 6.420643415959871274E-16, 11.49079834592231819, -28.42701364291157873 ) ) ;
#26959=DIRECTION ( 'NONE',  ( -1.000000000000000000, -0.000000000000000000, -0.000000000000000000 ) ) ;
#26964=DIRECTION ( 'NONE',  ( 0.000000000000000000, 0.000000000000000000, 1.000000000000000000 ) ) ;
#26966=CARTESIAN_POINT ( 'NONE',  ( 0.7564103445415252258, -32.71412841873081589, -8.947071897915261474 ) ) ;
#26976=EDGE_LOOP ( 'NONE', ( #28981, #20141, #13658, #6217, #11669, #9923 ) ) ;
#26977=DIRECTION ( 'NONE',  ( -1.000000000000000000, -0.000000000000000000, -0.000000000000000000 ) ) ;
#26978=CARTESIAN_POINT ( 'NONE',  ( 2.719051678294378327, 26.43909160613360854, 17.47815001432931226 ) ) ;
#26980=VERTEX_POINT ( 'NONE', #18765 ) ;
#26990=TOROIDAL_SURFACE ( 'NONE', #9946, 30.47050528711511674, 8.000000000000000000 ) ;
#26991=ADVANCED_FACE ( 'NONE', ( #1112 ), #27984, .F. ) ;
#26993=EDGE_CURVE ( 'NONE', #6886, #31215, #814, .T. ) ;
#27003=TOROIDAL_SURFACE ( 'NONE', #4247, 30.47050528711511674, 8.000000000000000000 ) ;
#27005=DIRECTION ( 'NONE',  ( 0.000000000000000000, 0.000000000000000000, 1.000000000000000000 ) ) ;
#27010=CARTESIAN_POINT ( 'NONE',  ( 0.1835379170796097859, -16.25808774470393914, 27.87656317279337514 ) ) ;
#27018=DIRECTION ( 'NONE',  ( -1.000000000000000000, -0.000000000000000000, 0.000000000000000000 ) ) ;
#27021=CARTESIAN_POINT ( 'NONE',  ( 1.394999999999999574, 6.714005886384948774, 33.75364837705175347 ) ) ;
#27024=AXIS2_PLACEMENT_3D ( 'NONE', #10806, #29668, #35023 ) ;
#27043=ORIENTED_EDGE ( 'NONE', *, *, #24987, .F. ) ;
#27053=ORIENTED_EDGE ( 'NONE', *, *, #18265, .T. ) ;
#27057=CARTESIAN_POINT ( 'NONE',  ( 1.040000000000001812, -1.891117961019736393, -34.36292081097834483 ) ) ;
#27059=CARTESIAN_POINT ( 'NONE',  ( 0.07098931954374571029, -0.5906890623668855644, 31.68904954958502884 ) ) ;
#27061=DIRECTION ( 'NONE',  ( 0.000000000000000000, 0.000000000000000000, 1.000000000000000000 ) ) ;
#27064=AXIS2_PLACEMENT_3D ( 'NONE', #4509, #15402, #26239 ) ;
#27065=CARTESIAN_POINT ( 'NONE',  ( 0.3923936511923831194, 30.27116788629744804, 13.00174666746672969 ) ) ;
#27069=ADVANCED_FACE ( 'NONE', ( #27802 ), #12226, .T. ) ;
#27070=AXIS2_PLACEMENT_3D ( 'NONE', #3222, #11248, #21740 ) ;
#27075=CYLINDRICAL_SURFACE ( 'NONE', #11102, 2.524999999999999467 ) ;
#27080=ORIENTED_EDGE ( 'NONE', *, *, #26356, .F. ) ;
#27083=CARTESIAN_POINT ( 'NONE',  ( 2.783084753007022627, 27.98916443103619045, -12.86217335695007868 ) ) ;
#27093=LINE ( 'NONE', #27620, #16354 ) ;
#27096=CARTESIAN_POINT ( 'NONE',  ( 0.02407890056655781832, -29.68817180695682723, 9.232883799364120847 ) ) ;
#27099=DIRECTION ( 'NONE',  ( 0.000000000000000000, 0.000000000000000000, 1.000000000000000000 ) ) ;
#27109=ORIENTED_EDGE ( 'NONE', *, *, #30579, .T. ) ;
#27114=DIRECTION ( 'NONE',  ( 1.000000000000000000, -0.000000000000000000, 0.000000000000000000 ) ) ;
#27116=TOROIDAL_SURFACE ( 'NONE', #18635, 30.47050528711512030, 8.000000000000000000 ) ;
#27120=ORIENTED_EDGE ( 'NONE', *, *, #21253, .F. ) ;
#27128=ORIENTED_EDGE ( 'NONE', *, *, #7786, .F. ) ;
#27137=VERTEX_POINT ( 'NONE', #17513 ) ;
#27148=LINE ( 'NONE', #2761, #11475 ) ;
#27149=ORIENTED_EDGE ( 'NONE', *, *, #14148, .F. ) ;
#27162=ADVANCED_FACE ( 'NONE', ( #18026 ), #26531, .T. ) ;
#27170=AXIS2_PLACEMENT_3D ( 'NONE', #10513, #27225, #24537 ) ;
#27179=EDGE_CURVE ( 'NONE', #11797, #7570, #26200, .T. ) ;
#27180=VECTOR ( 'NONE', #34575, 1000.000000000000000 ) ;
#27186=EDGE_CURVE ( 'NONE', #34878, #23180, #24101, .T. ) ;
#27188=CARTESIAN_POINT ( 'NONE',  ( -5.210000000000000853, 0.000000000000000000, 0.000000000000000000 ) ) ;
#27191=EDGE_LOOP ( 'NONE', ( #25446, #34510, #15029, #19783, #2325, #27906 ) ) ;
#27193=CYLINDRICAL_SURFACE ( 'NONE', #34377, 2.524999999999999467 ) ;
#27203=AXIS2_PLACEMENT_3D ( 'NONE', #26473, #23811, #31986 ) ;
#27214=DIRECTION ( 'NONE',  ( 1.000000000000000000, 0.000000000000000000, 0.000000000000000000 ) ) ;
#27215=CIRCLE ( 'NONE', #11893, 30.47050528711512030 ) ;
#27217=ORIENTED_EDGE ( 'NONE', *, *, #16737, .T. ) ;
#27220=CARTESIAN_POINT ( 'NONE',  ( 2.765921099433443331, -3.506335382740311868, -30.89238256715869468 ) ) ;
#27225=DIRECTION ( 'NONE',  ( -1.000000000000000000, -0.000000000000000000, 0.000000000000000000 ) ) ;
#27231=TOROIDAL_SURFACE ( 'NONE', #6206, 30.47050528711512030, 8.000000000000000000 ) ;
#27241=EDGE_CURVE ( 'NONE', #30030, #32472, #11798, .T. ) ;
#27247=B_SPLINE_CURVE_WITH_KNOTS ( 'NONE', 3,
 ( #11463, #17173, #8434, #22320, #3611, #14141 ),
 .UNSPECIFIED., .F., .F.,
 ( 4, 2, 4 ),
 ( 2.078540822438843793E-07, 0.001873406157010511566, 0.003746604459938779504 ),
 .UNSPECIFIED. ) ;
#27258=EDGE_CURVE ( 'NONE', #8335, #7441, #10526, .T. ) ;
#27266=AXIS2_PLACEMENT_3D ( 'NONE', #13400, #8037, #24233 ) ;
#27269=CARTESIAN_POINT ( 'NONE',  ( 2.789999999999999147, -13.59935610937951900, -28.90010281771846223 ) ) ;
#27277=CARTESIAN_POINT ( 'NONE',  ( 2.606461820648786620, -32.24848086092536903, -1.209851624881845611 ) ) ;
#27278=AXIS2_PLACEMENT_3D ( 'NONE', #18563, #10177, #26183 ) ;
#27279=ORIENTED_EDGE ( 'NONE', *, *, #20060, .T. ) ;
#27290=ORIENTED_EDGE ( 'NONE', *, *, #25497, .F. ) ;
#27302=LINE ( 'NONE', #3101, #19477 ) ;
#27305=CARTESIAN_POINT ( 'NONE',  ( 0.000000000000000000, 9.869977788041397915, -30.37666815053925973 ) ) ;
#27313=CARTESIAN_POINT ( 'NONE',  ( 0.1859802831645324950, 21.49213631816453329, -24.08729967255597870 ) ) ;
#27318=AXIS2_PLACEMENT_3D ( 'NONE', #258, #16295, #8084 ) ;
#27320=EDGE_LOOP ( 'NONE', ( #13358, #33504, #17827, #23743 ) ) ;
#27330=CARTESIAN_POINT ( 'NONE',  ( 1.749999999999999778, -24.90160365674851306, -23.75493189058367349 ) ) ;
#27339=CARTESIAN_POINT ( 'NONE',  ( 2.789999999999999147, 27.60935207499570154, -12.89090262359623118 ) ) ;
#27341=FACE_OUTER_BOUND ( 'NONE', #1307, .T. ) ;
#27346=CYLINDRICAL_SURFACE ( 'NONE', #20831, 16.19999999999999574 ) ;
#27349=DIRECTION ( 'NONE',  ( 0.000000000000000000, 0.000000000000000000, 1.000000000000000000 ) ) ;
#27354=ADVANCED_FACE ( 'NONE', ( #24383 ), #19416, .T. ) ;
#27355=CARTESIAN_POINT ( 'NONE',  ( 2.789999999999999147, 11.30192140231231868, 28.29696565125074414 ) ) ;
#27356=CARTESIAN_POINT ( 'NONE',  ( 2.790000000000000036, 30.15879770317926756, 5.529954278609506169 ) ) ;
#27362=AXIS2_PLACEMENT_3D ( 'NONE', #2673, #29561, #11045 ) ;
#27371=ORIENTED_EDGE ( 'NONE', *, *, #10923, .T. ) ;
#27376=CARTESIAN_POINT ( 'NONE',  ( 2.606461808080008158, 14.82544181993015009, -28.66416816974122383 ) ) ;
#27379=ORIENTED_EDGE ( 'NONE', *, *, #30049, .T. ) ;
#27382=PRODUCT ( 'short pitch roller chain wheel_s_iso_Chain wheel ISO - 25Z 05B-1 --25SA20.0S1', 'short pitch roller chain wheel_s_iso_Chain wheel ISO - 25Z 05B-1 --25SA20.0S1', '', ( #8910 ) ) ;
#27387=DIRECTION ( 'NONE',  ( 0.000000000000000000, 0.000000000000000000, 1.000000000000000000 ) ) ;
#27389=CIRCLE ( 'NONE', #28516, 34.41491905851385269 ) ;
#27391=ORIENTED_EDGE ( 'NONE', *, *, #32617, .T. ) ;
#27392=FACE_OUTER_BOUND ( 'NONE', #31744, .T. ) ;
#27396=CARTESIAN_POINT ( 'NONE',  ( 2.765921099433442443, 31.00221527374952046, -2.344426712874310148 ) ) ;
#27402=ORIENTED_EDGE ( 'NONE', *, *, #19114, .T. ) ;
#27403=FACE_OUTER_BOUND ( 'NONE', #19125, .T. ) ;
#27407=EDGE_CURVE ( 'NONE', #2604, #23345, #29832, .T. ) ;
#27417=FACE_OUTER_BOUND ( 'NONE', #1078, .T. ) ;
#27422=CYLINDRICAL_SURFACE ( 'NONE', #15380, 16.19999999999999929 ) ;
#27423=ORIENTED_EDGE ( 'NONE', *, *, #34788, .T. ) ;
#27435=CARTESIAN_POINT ( 'NONE',  ( 2.789999999999999147, -23.41952779159748133, -19.49300927180569687 ) ) ;
#27445=ADVANCED_FACE ( 'NONE', ( #3730 ), #23035, .T. ) ;
#27447=TOROIDAL_SURFACE ( 'NONE', #22317, 30.47050528711511674, 8.000000000000000000 ) ;
#27448=AXIS2_PLACEMENT_3D ( 'NONE', #10947, #27489, #16657 ) ;
#27449=CARTESIAN_POINT ( 'NONE',  ( 0.07098932983996933399, -11.11630839801572890, -29.68118041677939445 ) ) ;
#27456=VERTEX_POINT ( 'NONE', #30789 ) ;
#27459=CIRCLE ( 'NONE', #12131, 2.525000000000000799 ) ;
#27470=EDGE_CURVE ( 'NONE', #30793, #10340, #26420, .T. ) ;
#27475=EDGE_LOOP ( 'NONE', ( #1060, #23143, #26145, #9422, #26691, #5660, #9775, #29575, #29303, #28699, #18574, #22525, #7944, #24422, #3215, #15461, #11209, #1502, #21547, #9301, #12663, #22033, #16682, #28295, #14715, #9430, #21815, #12776, #23947, #16481, #11500, #13706, #27680, #23599, #30561, #32150, #34269, #14996, #6546, #25334, #19599, #21117, #27801, #29875, #15000, #25363, #23245, #29856, #32117, #31274, #29311, #416, #16111, #16825, #2557, #1352, #19814 ) ) ;
#27484=EDGE_LOOP ( 'NONE', ( #9853, #1391, #15631, #21666, #20549, #16700 ) ) ;
#27489=DIRECTION ( 'NONE',  ( -1.000000000000000000, 0.000000000000000000, -0.000000000000000000 ) ) ;
#27492=VECTOR ( 'NONE', #1790, 1000.000000000000000 ) ;
#27495=CARTESIAN_POINT ( 'NONE',  ( 2.783084753007022627, 27.98916443103619045, -12.86217335695007868 ) ) ;
#27496=CARTESIAN_POINT ( 'NONE',  ( 2.719010676179473229, -27.07245655034563114, -16.48110659958421920 ) ) ;
#27505=CARTESIAN_POINT ( 'NONE',  ( 2.789999999999999147, 6.312585643774527355, 29.77790610619688394 ) ) ;
#27523=AXIS2_PLACEMENT_3D ( 'NONE', #4589, #2122, #31829 ) ;
#27524=CARTESIAN_POINT ( 'NONE',  ( 1.749999999999999778, 6.714005886384948774, 33.75364837705175347 ) ) ;
#27529=DIRECTION ( 'NONE',  ( -1.000000000000000000, 0.000000000000000000, 0.000000000000000000 ) ) ;
#27530=CARTESIAN_POINT ( 'NONE',  ( 2.790000000000081304, 4.061185680397615627, -30.39260865248084187 ) ) ;
#27531=CARTESIAN_POINT ( 'NONE',  ( 8.000000000000000000, 0.000000000000000000, 0.000000000000000000 ) ) ;
#27532=ORIENTED_EDGE ( 'NONE', *, *, #10636, .T. ) ;
#27534=CARTESIAN_POINT ( 'NONE',  ( 0.000000000000000000, 23.28319895603611300, -21.86437915510192909 ) ) ;
#27542=DIRECTION ( 'NONE',  ( 0.000000000000000000, 0.000000000000000000, 1.000000000000000000 ) ) ;
#27543=DIRECTION ( 'NONE',  ( 0.000000000000000000, 0.000000000000000000, 1.000000000000000000 ) ) ;
#27552=CARTESIAN_POINT ( 'NONE',  ( 2.261199742992266337, -33.38088972941607580, 0.7716149733912494035 ) ) ;
#27563=CYLINDRICAL_SURFACE ( 'NONE', #25083, 34.41491905851385269 ) ;
#27568=EDGE_CURVE ( 'NONE', #31871, #22788, #33844, .T. ) ;
#27580=ORIENTED_EDGE ( 'NONE', *, *, #22942, .F. ) ;
#27583=LINE ( 'NONE', #3196, #1362 ) ;
#27586=DIRECTION ( 'NONE',  ( -1.000000000000000000, -0.000000000000000000, -0.000000000000000000 ) ) ;
#27599=ORIENTED_EDGE ( 'NONE', *, *, #7941, .F. ) ;
#27603=CARTESIAN_POINT ( 'NONE',  ( 2.765921099433441110, -17.95514392185398833, -25.38201125280375692 ) ) ;
#27610=CARTESIAN_POINT ( 'NONE',  ( 0.02407890056655695096, 11.80989368511462523, 28.76039115933989976 ) ) ;
#27613=VERTEX_POINT ( 'NONE', #7261 ) ;
#27618=ORIENTED_EDGE ( 'NONE', *, *, #23868, .F. ) ;
#27620=CARTESIAN_POINT ( 'NONE',  ( 2.789999999999999147, -20.35927063852789232, -22.08513060777193004 ) ) ;
#27621=CARTESIAN_POINT ( 'NONE',  ( 0.02407890056655651728, 7.350529080603541487, 30.20932655202940254 ) ) ;
#27624=DIRECTION ( 'NONE',  ( -1.000000000000000000, -0.000000000000000000, -0.000000000000000000 ) ) ;
#27637=EDGE_CURVE ( 'NONE', #19620, #9427, #13928, .T. ) ;
#27642=ORIENTED_EDGE ( 'NONE', *, *, #5572, .T. ) ;
#27647=LINE ( 'NONE', #29793, #20375 ) ;
#27648=CARTESIAN_POINT ( 'NONE',  ( 2.789999999999999147, 0.000000000000000000, 0.000000000000000000 ) ) ;
#27662=CARTESIAN_POINT ( 'NONE',  ( 0.000000000000000000, 3.909681563762119172, -30.21863799912381054 ) ) ;
#27663=CARTESIAN_POINT ( 'NONE',  ( 1.749999999999999778, -18.21166265554811403, 29.20140402659732359 ) ) ;
#27665=DIRECTION ( 'NONE',  ( 0.000000000000000000, 0.000000000000000000, 1.000000000000000000 ) ) ;
#27668=LINE ( 'NONE', #16846, #2332 ) ;
#27669=CARTESIAN_POINT ( 'NONE',  ( 0.000000000000000000, 0.000000000000000000, 0.000000000000000000 ) ) ;
#27670=B_SPLINE_CURVE_WITH_KNOTS ( 'NONE', 3,
 ( #16227, #27059, #14953, #28467, #33281, #22431 ),
 .UNSPECIFIED., .F., .F.,
 ( 4, 2, 4 ),
 ( 2.078540817596000944E-07, 0.001873406157010270006, 0.003746604459938780371 ),
 .UNSPECIFIED. ) ;
#27673=ORIENTED_EDGE ( 'NONE', *, *, #3839, .F. ) ;
#27676=ORIENTED_EDGE ( 'NONE', *, *, #1099, .F. ) ;
#27677=EDGE_LOOP ( 'NONE', ( #30036, #2820, #9626, #18139 ) ) ;
#27679=CIRCLE ( 'NONE', #1548, 2.525000000000000799 ) ;
#27680=ORIENTED_EDGE ( 'NONE', *, *, #29895, .F. ) ;
#27684=ORIENTED_EDGE ( 'NONE', *, *, #13661, .F. ) ;
#27687=CARTESIAN_POINT ( 'NONE',  ( 2.606461903588221940, -22.67993007562043317, -22.95754798008726993 ) ) ;
#27689=B_SPLINE_CURVE_WITH_KNOTS ( 'NONE', 3,
 ( #9587, #25769, #26465, #17783, #14935, #4557 ),
 .UNSPECIFIED., .F., .F.,
 ( 4, 2, 4 ),
 ( 2.555309558362774114E-07, 0.001873453885876978078, 0.003746652240798119780 ),
 .UNSPECIFIED. ) ;
#27692=CARTESIAN_POINT ( 'NONE',  ( 0.1859802785888828025, -31.54566302605132222, 6.854274004867739301 ) ) ;
#27693=CARTESIAN_POINT ( 'NONE',  ( 1.395000000000002238, 27.68252950111368094, -20.44661865013457813 ) ) ;
#27727=VERTEX_POINT ( 'NONE', #17988 ) ;
#27736=CARTESIAN_POINT ( 'NONE',  ( -2.448281906437820454E-16, -29.22790002295985090, 9.266248432308520577 ) ) ;
#27737=B_SPLINE_CURVE_WITH_KNOTS ( 'NONE', 3,
 ( #5286, #27356, #10824, #2973 ),
 .UNSPECIFIED., .F., .F.,
 ( 4, 4 ),
 ( 0.005298484651059772073, 0.005985351487543621660 ),
 .UNSPECIFIED. ) ;
#27738=CARTESIAN_POINT ( 'NONE',  ( 2.261199765623164826, -29.62362497318111920, -15.40519487321921765 ) ) ;
#27741=VERTEX_POINT ( 'NONE', #23986 ) ;
#27743=CARTESIAN_POINT ( 'NONE',  ( 2.765921099433441110, -17.95514392185398833, -25.38201125280375692 ) ) ;
#27747=ORIENTED_EDGE ( 'NONE', *, *, #3213, .F. ) ;
#27750=AXIS2_PLACEMENT_3D ( 'NONE', #10545, #5354, #19267 ) ;
#27751=ADVANCED_FACE ( 'NONE', ( #16362 ), #27193, .F. ) ;
#27754=CARTESIAN_POINT ( 'NONE',  ( 2.765921099433442443, 20.99477179376825120, 22.93149026599753526 ) ) ;
#27766=ORIENTED_EDGE ( 'NONE', *, *, #25497, .T. ) ;
#27768=ORIENTED_EDGE ( 'NONE', *, *, #1408, .F. ) ;
#27771=EDGE_CURVE ( 'NONE', #29651, #30403, #23609, .T. ) ;
#27781=DIRECTION ( 'NONE',  ( -1.000000000000000000, 0.000000000000000000, 0.000000000000000000 ) ) ;
#27783=ORIENTED_EDGE ( 'NONE', *, *, #21401, .F. ) ;
#27794=CARTESIAN_POINT ( 'NONE',  ( 2.719010685383924208, 31.58942871418359744, -2.579295332369116789 ) ) ;
#27801=ORIENTED_EDGE ( 'NONE', *, *, #16935, .F. ) ;
#27802=FACE_OUTER_BOUND ( 'NONE', #24260, .T. ) ;
#27810=AXIS2_PLACEMENT_3D ( 'NONE', #34987, #16301, #13444 ) ;
#27811=B_SPLINE_CURVE_WITH_KNOTS ( 'NONE', 3,
 ( #4010, #14904, #1366, #17752 ),
 .UNSPECIFIED., .F., .F.,
 ( 4, 4 ),
 ( 0.005298419352602242068, 0.005985287046740441104 ),
 .UNSPECIFIED. ) ;
#27823=VERTEX_POINT ( 'NONE', #29873 ) ;
#27832=ADVANCED_FACE ( 'NONE', ( #7793 ), #32137, .T. ) ;
#27838=FACE_OUTER_BOUND ( 'NONE', #21884, .T. ) ;
#27839=LINE ( 'NONE', #14514, #26892 ) ;
#27849=EDGE_CURVE ( 'NONE', #18440, #14675, #5471, .T. ) ;
#27855=ORIENTED_EDGE ( 'NONE', *, *, #13110, .F. ) ;
#27857=ORIENTED_EDGE ( 'NONE', *, *, #2849, .T. ) ;
#27861=DIRECTION ( 'NONE',  ( 0.000000000000000000, 0.000000000000000000, 1.000000000000000000 ) ) ;
#27863=CARTESIAN_POINT ( 'NONE',  ( 0.006915246992955798207, 27.98916443103565399, -12.86217335695007868 ) ) ;
#27873=FACE_OUTER_BOUND ( 'NONE', #7895, .T. ) ;
#27877=FACE_OUTER_BOUND ( 'NONE', #13106, .T. ) ;
#27892=CYLINDRICAL_SURFACE ( 'NONE', #29701, 34.41491905851385269 ) ;
#27901=DIRECTION ( 'NONE',  ( 0.000000000000000000, 1.374038396813312784E-15, -1.000000000000000000 ) ) ;
#27906=ORIENTED_EDGE ( 'NONE', *, *, #16611, .F. ) ;
#27910=CARTESIAN_POINT ( 'NONE',  ( 0.02407890056655781832, -29.68817180695682723, 9.232883799364120847 ) ) ;
#27916=CYLINDRICAL_SURFACE ( 'NONE', #845, 34.41491905851385269 ) ;
#27920=DIRECTION ( 'NONE',  ( 0.000000000000000000, 0.000000000000000000, 1.000000000000000000 ) ) ;
#27926=ORIENTED_EDGE ( 'NONE', *, *, #4836, .T. ) ;
#27928=CIRCLE ( 'NONE', #12043, 2.525000000000001243 ) ;
#27968=AXIS2_PLACEMENT_3D ( 'NONE', #19185, #30022, #3136 ) ;
#27970=CARTESIAN_POINT ( 'NONE',  ( 0.000000000000000000, -20.35927063852789232, -24.61013060777193218 ) ) ;
#27975=DIRECTION ( 'NONE',  ( 0.000000000000000000, 0.000000000000000000, 1.000000000000000000 ) ) ;
#27980=CIRCLE ( 'NONE', #17210, 30.47050528711511674 ) ;
#27983=ORIENTED_EDGE ( 'NONE', *, *, #2127, .F. ) ;
#27984=CYLINDRICAL_SURFACE ( 'NONE', #23556, 2.524999999999999467 ) ;
#28000=EDGE_LOOP ( 'NONE', ( #17541, #2551, #23358, #1023 ) ) ;
#28001=CIRCLE ( 'NONE', #1851, 34.41491905851385269 ) ;
#28005=DIRECTION ( 'NONE',  ( -1.000000000000000000, -0.000000000000000000, -0.000000000000000000 ) ) ;
#28006=ADVANCED_FACE ( 'NONE', ( #25569 ), #8502, .T. ) ;
#28011=ORIENTED_EDGE ( 'NONE', *, *, #17426, .F. ) ;
#28019=CYLINDRICAL_SURFACE ( 'NONE', #23996, 2.525000000000001243 ) ;
#28028=FACE_OUTER_BOUND ( 'NONE', #25353, .T. ) ;
#28032=CIRCLE ( 'NONE', #21771, 10.00000000000000000 ) ;
#28036=ORIENTED_EDGE ( 'NONE', *, *, #7901, .F. ) ;
#28046=ORIENTED_EDGE ( 'NONE', *, *, #34382, .F. ) ;
#28047=ORIENTED_EDGE ( 'NONE', *, *, #14148, .T. ) ;
#28049=DIRECTION ( 'NONE',  ( 0.000000000000000000, 0.000000000000000000, 1.000000000000000000 ) ) ;
#28050=DIRECTION ( 'NONE',  ( -1.000000000000000000, -0.000000000000000000, -0.000000000000000000 ) ) ;
#28056=ADVANCED_FACE ( 'NONE', ( #31440 ), #22474, .T. ) ;
#28060=ORIENTED_EDGE ( 'NONE', *, *, #24788, .F. ) ;
#28061=CARTESIAN_POINT ( 'NONE',  ( 2.789999999999999147, 14.63235270440974922, -27.43224275967423509 ) ) ;
#28071=CARTESIAN_POINT ( 'NONE',  ( 2.261199741936142704, 14.91106968280055156, 29.87539438830526706 ) ) ;
#28078=EDGE_CURVE ( 'NONE', #19079, #7089, #9192, .T. ) ;
#28081=TOROIDAL_SURFACE ( 'NONE', #5907, 30.47050528711512030, 8.000000000000000000 ) ;
#28085=EDGE_CURVE ( 'NONE', #8194, #9865, #8303, .T. ) ;
#28097=VERTEX_POINT ( 'NONE', #20767 ) ;
#28115=CYLINDRICAL_SURFACE ( 'NONE', #21799, 16.19999999999999574 ) ;
#28117=DIRECTION ( 'NONE',  ( 0.000000000000000000, -0.2486898871648554887, 0.9685831611286309650 ) ) ;
#28134=VERTEX_POINT ( 'NONE', #14917 ) ;
#28147=DIRECTION ( 'NONE',  ( 0.000000000000000000, 0.8443279255020087470, 0.5358267949790064266 ) ) ;
#28151=ORIENTED_EDGE ( 'NONE', *, *, #13776, .T. ) ;
#28159=CARTESIAN_POINT ( 'NONE',  ( 0.02407890056655651728, 11.80989368511502846, -28.76039115933972923 ) ) ;
#28160=DIRECTION ( 'NONE',  ( -1.000000000000000000, 0.000000000000000000, 0.000000000000000000 ) ) ;
#28163=CARTESIAN_POINT ( 'NONE',  ( 2.606461941304143881, -8.814691041839068930, -31.04399216667579964 ) ) ;
#28165=AXIS2_PLACEMENT_3D ( 'NONE', #15740, #12370, #12533 ) ;
#28168=EDGE_CURVE ( 'NONE', #2456, #23263, #10456, .T. ) ;
#28175=VERTEX_POINT ( 'NONE', #16141 ) ;
#28186=DIRECTION ( 'NONE',  ( -1.000000000000000000, 0.000000000000000000, -0.000000000000000000 ) ) ;
#28187=B_SPLINE_CURVE_WITH_KNOTS ( 'NONE', 3,
 ( #5506, #14072, #24382, #9 ),
 .UNSPECIFIED., .F., .F.,
 ( 4, 4 ),
 ( 2.075676022607228905E-07, 0.0006879433439099471746 ),
 .UNSPECIFIED. ) ;
#28189=CARTESIAN_POINT ( 'NONE',  ( 0.02407890056655738464, -29.68817180695669578, -9.232883799364548949 ) ) ;
#28197=CARTESIAN_POINT ( 'NONE',  ( 0.0001801434340936737804, -25.83993731729792742, -16.24881338200996694 ) ) ;
#28202=EDGE_CURVE ( 'NONE', #26104, #5255, #14701, .T. ) ;
#28214=ORIENTED_EDGE ( 'NONE', *, *, #12067, .T. ) ;
#28217=ORIENTED_EDGE ( 'NONE', *, *, #21645, .T. ) ;
#28221=DIRECTION ( 'NONE',  ( 0.000000000000000000, 0.000000000000000000, 1.000000000000000000 ) ) ;
#28225=CARTESIAN_POINT ( 'NONE',  ( 1.040000000000000702, -10.89151784028311809, 32.64600270996213283 ) ) ;
#28226=VECTOR ( 'NONE', #9627, 1000.000000000000000 ) ;
#28232=DIRECTION ( 'NONE',  ( -1.000000000000000000, 0.000000000000000000, 0.000000000000000000 ) ) ;
#28233=CARTESIAN_POINT ( 'NONE',  ( -10.00000000000000000, 0.000000000000000000, 0.000000000000000000 ) ) ;
#28234=LINE ( 'NONE', #30369, #12946 ) ;
#28237=DIRECTION ( 'NONE',  ( 0.000000000000000000, 0.000000000000000000, 1.000000000000000000 ) ) ;
#28238=CARTESIAN_POINT ( 'NONE',  ( 0.02407890056655825201, -3.506335382740311868, -30.89238256715869468 ) ) ;
#28239=DIRECTION ( 'NONE',  ( -1.000000000000000000, 0.000000000000000000, -0.000000000000000000 ) ) ;
#28247=ORIENTED_EDGE ( 'NONE', *, *, #28761, .F. ) ;
#28251=AXIS2_PLACEMENT_3D ( 'NONE', #26513, #2135, #7641 ) ;
#28258=EDGE_CURVE ( 'NONE', #21475, #9815, #27148, .T. ) ;
#28262=CARTESIAN_POINT ( 'NONE',  ( 2.765921099433442443, -30.46391896562403190, -6.211548095912885259 ) ) ;
#28264=DIRECTION ( 'NONE',  ( -1.000000000000000000, 0.000000000000000000, -0.000000000000000000 ) ) ;
#28266=CARTESIAN_POINT ( 'NONE',  ( 0.02407890056655608360, 14.63235270440974922, -27.43224275967423509 ) ) ;
#28267=FACE_OUTER_BOUND ( 'NONE', #29570, .T. ) ;
#28270=ORIENTED_EDGE ( 'NONE', *, *, #28660, .T. ) ;
#28280=CARTESIAN_POINT ( 'NONE',  ( 2.765921099433441110, 11.80989368511462523, 28.76039115933989976 ) ) ;
#28282=CARTESIAN_POINT ( 'NONE',  ( 1.040000000000000924, 0.000000000000000000, 0.000000000000000000 ) ) ;
#28295=ORIENTED_EDGE ( 'NONE', *, *, #4836, .F. ) ;
#28316=CARTESIAN_POINT ( 'NONE',  ( 0.02407890056655738464, 24.20451283648857554, -19.51346322004903300 ) ) ;
#28319=CARTESIAN_POINT ( 'NONE',  ( 2.789999999999999147, -30.43331811787861341, 0.6209492052231032622 ) ) ;
#28323=CARTESIAN_POINT ( 'NONE',  ( 1.039999999999999591, -18.21166265554809627, 29.20140402659733425 ) ) ;
#28324=DIRECTION ( 'NONE',  ( -1.000000000000000000, 0.000000000000000000, -0.000000000000000000 ) ) ;
#28327=EDGE_CURVE ( 'NONE', #23446, #24976, #21487, .T. ) ;
#28337=CIRCLE ( 'NONE', #31179, 30.47050528711512030 ) ;
#28345=CYLINDRICAL_SURFACE ( 'NONE', #8048, 2.524999999999999467 ) ;
#28346=CIRCLE ( 'NONE', #11867, 30.47050528711512030 ) ;
#28351=AXIS2_PLACEMENT_3D ( 'NONE', #8864, #22578, #6003 ) ;
#28354=VERTEX_POINT ( 'NONE', #33001 ) ;
#28355=ORIENTED_EDGE ( 'NONE', *, *, #21069, .T. ) ;
#28357=CARTESIAN_POINT ( 'NONE',  ( 2.789999999999999147, -17.83604598421683107, 24.70480026434158916 ) ) ;
#28358=AXIS2_PLACEMENT_3D ( 'NONE', #33566, #1013, #3664 ) ;
#28359=VERTEX_POINT ( 'NONE', #24827 ) ;
#28360=CARTESIAN_POINT ( 'NONE',  ( 1.749999999999999778, -2.430610048905780030, -34.32897884578301984 ) ) ;
#28368=CYLINDRICAL_SURFACE ( 'NONE', #15417, 16.19999999999999574 ) ;
#28370=ORIENTED_EDGE ( 'NONE', *, *, #16448, .T. ) ;
#28378=CARTESIAN_POINT ( 'NONE',  ( 2.789999999999999147, 28.95078156989557527, 9.502838467758159879 ) ) ;
#28379=DIRECTION ( 'NONE',  ( -1.000000000000000000, -0.000000000000000000, 0.000000000000000000 ) ) ;
#28390=B_SPLINE_CURVE_WITH_KNOTS ( 'NONE', 3,
 ( #12483, #23327, #7113, #18013, #28837, #13698 ),
 .UNSPECIFIED., .F., .F.,
 ( 4, 2, 4 ),
 ( 4.404817130267440109E-07, 0.001874269701320914775, 0.003748098920928802889 ),
 .UNSPECIFIED. ) ;
#28392=FACE_OUTER_BOUND ( 'NONE', #12884, .T. ) ;
#28404=ORIENTED_EDGE ( 'NONE', *, *, #24356, .T. ) ;
#28406=EDGE_CURVE ( 'NONE', #16394, #245, #4602, .T. ) ;
#28413=AXIS2_PLACEMENT_3D ( 'NONE', #638, #3300, #11499 ) ;
#28415=EDGE_CURVE ( 'NONE', #9440, #19893, #21116, .T. ) ;
#28418=ADVANCED_FACE ( 'NONE', ( #28392 ), #20386, .T. ) ;
#28425=CARTESIAN_POINT ( 'NONE',  ( 2.765921099433441999, 4.286445725888479608, -30.79383171238939809 ) ) ;
#28426=DIRECTION ( 'NONE',  ( -1.000000000000000000, -0.000000000000000000, -0.000000000000000000 ) ) ;
#28433=AXIS2_PLACEMENT_3D ( 'NONE', #13036, #34383, #13386 ) ;
#28438=CARTESIAN_POINT ( 'NONE',  ( 2.789999999999999147, 29.94779062842786743, 5.619744560739183825 ) ) ;
#28439=DIRECTION ( 'NONE',  ( -1.000000000000000000, 0.000000000000000000, -0.000000000000000000 ) ) ;
#28450=DIRECTION ( 'NONE',  ( -1.000000000000000000, -0.000000000000000000, -0.000000000000000000 ) ) ;
#28456=VERTEX_POINT ( 'NONE', #25710 ) ;
#28460=CARTESIAN_POINT ( 'NONE',  ( 50.00050000000000239, 12.80000000000000071, -3.000000000000000000 ) ) ;
#28466=AXIS2_PLACEMENT_3D ( 'NONE', #21632, #32475, #29821 ) ;
#28467=CARTESIAN_POINT ( 'NONE',  ( 0.5248942429777062602, -1.320925567293482761, 33.35364885818385972 ) ) ;
#28481=FACE_OUTER_BOUND ( 'NONE', #28000, .T. ) ;
#28483=ORIENTED_EDGE ( 'NONE', *, *, #27637, .T. ) ;
#28484=CARTESIAN_POINT ( 'NONE',  ( 1.039999999999999591, -25.27164158951584483, 23.36088151536909052 ) ) ;
#28488=CIRCLE ( 'NONE', #14302, 2.525000000000001243 ) ;
#28495=DIRECTION ( 'NONE',  ( -1.000000000000000000, -0.000000000000000000, -0.000000000000000000 ) ) ;
#28500=B_SPLINE_CURVE_WITH_KNOTS ( 'NONE', 3,
 ( #5239, #18801, #5590, #27313, #19326, #24636 ),
 .UNSPECIFIED., .F., .F.,
 ( 4, 2, 4 ),
 ( 4.404817058690223214E-07, 0.001874269648070855032, 0.003748098814435841305 ),
 .UNSPECIFIED. ) ;
#28503=DIRECTION ( 'NONE',  ( 0.000000000000000000, 0.000000000000000000, 1.000000000000000000 ) ) ;
#28509=CARTESIAN_POINT ( 'NONE',  ( 0.000000000000000000, -7.666252171205264254, -29.49034198003815632 ) ) ;
#28516=AXIS2_PLACEMENT_3D ( 'NONE', #22023, #3322, #24324 ) ;
#28517=AXIS2_PLACEMENT_3D ( 'NONE', #14709, #3981, #21385 ) ;
#28519=ORIENTED_EDGE ( 'NONE', *, *, #23153, .T. ) ;
#28523=EDGE_CURVE ( 'NONE', #30531, #7014, #7466, .T. ) ;
#28530=CIRCLE ( 'NONE', #13193, 2.524999999999999467 ) ;
#28533=DIRECTION ( 'NONE',  ( -1.000000000000000000, -0.000000000000000000, -0.000000000000000000 ) ) ;
#28538=CARTESIAN_POINT ( 'NONE',  ( 0.5288002343768358759, -29.62362497318133947, 15.40519487321878778 ) ) ;
#28539=CARTESIAN_POINT ( 'NONE',  ( 0.006892381647577837216, 18.40335333576913612, -24.78429060331921718 ) ) ;
#28540=DIRECTION ( 'NONE',  ( 0.000000000000000000, 0.000000000000000000, 1.000000000000000000 ) ) ;
#28541=CARTESIAN_POINT ( 'NONE',  ( 2.789999999999999147, 25.67797970382134309, 16.40405592474765939 ) ) ;
#28542=ORIENTED_EDGE ( 'NONE', *, *, #19016, .F. ) ;
#28560=ORIENTED_EDGE ( 'NONE', *, *, #8197, .T. ) ;
#28566=AXIS2_PLACEMENT_3D ( 'NONE', #26579, #2200, #13073 ) ;
#28567=EDGE_CURVE ( 'NONE', #16094, #24969, #4883, .T. ) ;
#28575=CARTESIAN_POINT ( 'NONE',  ( 0.07094833748228242254, -18.14830959286913270, 25.98365187356515804 ) ) ;
#28582=LINE ( 'NONE', #26077, #30559 ) ;
#28596=CIRCLE ( 'NONE', #13252, 2.525000000000001688 ) ;
#28598=ORIENTED_EDGE ( 'NONE', *, *, #4490, .T. ) ;
#28601=VERTEX_POINT ( 'NONE', #13551 ) ;
#28606=ADVANCED_FACE ( 'NONE', ( #27417 ), #3025, .T. ) ;
#28621=CARTESIAN_POINT ( 'NONE',  ( 2.765921099433441555, 24.20451283648857554, -19.51346322004903300 ) ) ;
#28623=CARTESIAN_POINT ( 'NONE',  ( 0.02407890056655825201, -31.05158812718220673, -1.559667679918931738 ) ) ;
#28634=CARTESIAN_POINT ( 'NONE',  ( 2.789999999999999147, -20.92506858792771851, 22.14933852381669510 ) ) ;
#28637=AXIS2_PLACEMENT_3D ( 'NONE', #33537, #20030, #798 ) ;
#28645=B_SPLINE_CURVE_WITH_KNOTS ( 'NONE', 3,
 ( #23532, #28700, #31711, #7319 ),
 .UNSPECIFIED., .F., .F.,
 ( 4, 4 ),
 ( 0.005298392425857884405, 0.005985260475359765499 ),
 .UNSPECIFIED. ) ;
#28649=CARTESIAN_POINT ( 'NONE',  ( 2.765921099433441999, -29.68817180695669578, -9.232883799364548949 ) ) ;
#28658=AXIS2_PLACEMENT_3D ( 'NONE', #32727, #26860, #32203 ) ;
#28660=EDGE_CURVE ( 'NONE', #24520, #18645, #9228, .T. ) ;
#28662=CARTESIAN_POINT ( 'NONE',  ( 2.789999999999999147, 27.98916443103621177, -15.38717335695007904 ) ) ;
#28673=ORIENTED_EDGE ( 'NONE', *, *, #18028, .T. ) ;
#28690=EDGE_CURVE ( 'NONE', #2454, #7193, #25237, .T. ) ;
#28691=CYLINDRICAL_SURFACE ( 'NONE', #17069, 16.19999999999999929 ) ;
#28694=ORIENTED_EDGE ( 'NONE', *, *, #30379, .T. ) ;
#28695=ORIENTED_EDGE ( 'NONE', *, *, #31270, .T. ) ;
#28699=ORIENTED_EDGE ( 'NONE', *, *, #7630, .F. ) ;
#28700=CARTESIAN_POINT ( 'NONE',  ( 2.789999999999998703, 14.57887998322662781, -26.97387222978612797 ) ) ;
#28703=EDGE_LOOP ( 'NONE', ( #7235, #27747, #10108, #24714, #29398, #17991 ) ) ;
#28712=CARTESIAN_POINT ( 'NONE',  ( 8.000000000000000000, 0.000000000000000000, 0.000000000000000000 ) ) ;
#28717=CARTESIAN_POINT ( 'NONE',  ( 1.040000000000001368, -33.26546734453825138, 8.820166447041648539 ) ) ;
#28730=ADVANCED_FACE ( 'NONE', ( #17084 ), #2861, .T. ) ;
#28731=VECTOR ( 'NONE', #12560, 1000.000000000000000 ) ;
#28740=EDGE_LOOP ( 'NONE', ( #13013, #765, #13213, #14219 ) ) ;
#28747=VERTEX_POINT ( 'NONE', #30945 ) ;
#28760=CARTESIAN_POINT ( 'NONE',  ( 2.789999999999999147, -29.63162325403024511, 6.967017504691655816 ) ) ;
#28761=EDGE_CURVE ( 'NONE', #32672, #21866, #7405, .T. ) ;
#28770=CARTESIAN_POINT ( 'NONE',  ( 1.040000000000000036, 31.89769921723006263, -12.91988538846923973 ) ) ;
#28771=AXIS2_PLACEMENT_3D ( 'NONE', #16045, #4980, #34722 ) ;
#28775=EDGE_CURVE ( 'NONE', #33378, #31064, #30349, .T. ) ;
#28776=CARTESIAN_POINT ( 'NONE',  ( -5.210000000000000853, 0.000000000000000000, 0.000000000000000000 ) ) ;
#28794=CARTESIAN_POINT ( 'NONE',  ( 0.006871054928023897015, -3.550602046213657381, 30.66465032581540839 ) ) ;
#28808=CARTESIAN_POINT ( 'NONE',  ( 2.265105833353615150, -24.85743842207130427, 22.27820639183311968 ) ) ;
#28809=ORIENTED_EDGE ( 'NONE', *, *, #12159, .F. ) ;
#28822=AXIS2_PLACEMENT_3D ( 'NONE', #9981, #2490, #20838 ) ;
#28824=CARTESIAN_POINT ( 'NONE',  ( 0.02407890056655695096, 11.80989368511462523, 28.76039115933989976 ) ) ;
#28837=CARTESIAN_POINT ( 'NONE',  ( 2.719051674337184199, 19.10378521888278058, -25.28945800968145363 ) ) ;
#28847=LINE ( 'NONE', #18192, #27492 ) ;
#28859=( NAMED_UNIT ( * ) PLANE_ANGLE_UNIT ( ) SI_UNIT ( $, .RADIAN. ) );
#28860=ORIENTED_EDGE ( 'NONE', *, *, #4129, .T. ) ;
#28864=ORIENTED_EDGE ( 'NONE', *, *, #13987, .T. ) ;
#28878=CARTESIAN_POINT ( 'NONE',  ( -8.331222508929960727E-14, -29.22921979676802451, -9.265873697119378249 ) ) ;
#28899=ORIENTED_EDGE ( 'NONE', *, *, #27241, .F. ) ;
#28919=DIRECTION ( 'NONE',  ( -1.000000000000000000, -0.000000000000000000, -0.000000000000000000 ) ) ;
#28927=ORIENTED_EDGE ( 'NONE', *, *, #17651, .F. ) ;
#28931=CARTESIAN_POINT ( 'NONE',  ( 0.02407890056655695096, -21.56796757982826307, 22.39322359481599278 ) ) ;
#28935=AXIS2_PLACEMENT_3D ( 'NONE', #24102, #26959, #26605 ) ;
#28943=FACE_OUTER_BOUND ( 'NONE', #7585, .T. ) ;
#28945=EDGE_CURVE ( 'NONE', #17061, #33511, #1048, .T. ) ;
#28950=EDGE_LOOP ( 'NONE', ( #28270, #4116, #10837, #31779, #11911, #1732 ) ) ;
#28954=CARTESIAN_POINT ( 'NONE',  ( 2.783107534982237841, -0.3207854480225766913, -30.86813304286363646 ) ) ;
#28956=DIRECTION ( 'NONE',  ( 1.000000000000000000, -0.000000000000000000, -0.000000000000000000 ) ) ;
#28962=CARTESIAN_POINT ( 'NONE',  ( 0.7564103424913883877, 33.71046419695405660, -3.724096820061226332 ) ) ;
#28970=EDGE_CURVE ( 'NONE', #27456, #5322, #21627, .T. ) ;
#28981=ORIENTED_EDGE ( 'NONE', *, *, #926, .F. ) ;
#28982=CARTESIAN_POINT ( 'NONE',  ( 2.789999999999999147, 20.79173593595296055, -22.27454621808740853 ) ) ;
#28983=ORIENTED_EDGE ( 'NONE', *, *, #32376, .F. ) ;
#28985=CARTESIAN_POINT ( 'NONE',  ( 0.5288002349688907255, -17.23487904370236734, -28.59786932736749421 ) ) ;
#28986=AXIS2_PLACEMENT_3D ( 'NONE', #25623, #1254, #4074 ) ;
#28988=CARTESIAN_POINT ( 'NONE',  ( 0.02407890056655564992, -0.3931553186911057041, -31.08824725498900676 ) ) ;
#28990=ORIENTED_EDGE ( 'NONE', *, *, #31875, .F. ) ;
#28994=ADVANCED_FACE ( 'NONE', ( #25153 ), #16341, .F. ) ;
#28995=EDGE_CURVE ( 'NONE', #13078, #3245, #22686, .T. ) ;
#29003=CARTESIAN_POINT ( 'NONE',  ( 2.265105769669975455, 26.54141775410149862, 20.24262527923012911 ) ) ;
#29007=CARTESIAN_POINT ( 'NONE',  ( 2.719010690716784140, 21.26205330531154658, -23.50467731722535447 ) ) ;
#29015=CARTESIAN_POINT ( 'NONE',  ( 2.789999999999999147, 0.000000000000000000, 0.000000000000000000 ) ) ;
#29019=DIRECTION ( 'NONE',  ( 0.000000000000000000, 0.000000000000000000, 1.000000000000000000 ) ) ;
#29022=CARTESIAN_POINT ( 'NONE',  ( 1.040000000000000702, -10.37741591188916779, 32.81304455236864470 ) ) ;
#29025=AXIS2_PLACEMENT_3D ( 'NONE', #1389, #33424, #8866 ) ;
#29029=ADVANCED_FACE ( 'NONE', ( #7952 ), #25332, .F. ) ;
#29031=VECTOR ( 'NONE', #3269, 1000.000000000000000 ) ;
#29032=CARTESIAN_POINT ( 'NONE',  ( 1.039999999999999813, 14.89726405156260114, -31.02351007835961383 ) ) ;
#29034=ORIENTED_EDGE ( 'NONE', *, *, #10081, .F. ) ;
#29035=VECTOR ( 'NONE', #23781, 1000.000000000000000 ) ;
#29038=EDGE_CURVE ( 'NONE', #30641, #7395, #24319, .T. ) ;
#29047=CARTESIAN_POINT ( 'NONE',  ( 0.000000000000000000, 0.000000000000000000, 0.000000000000000000 ) ) ;
#29050=CARTESIAN_POINT ( 'NONE',  ( 0.1835381919199922940, 14.82544181992975396, 28.66416816974143345 ) ) ;
#29061=DIRECTION ( 'NONE',  ( -1.000000000000000000, -0.000000000000000000, -0.000000000000000000 ) ) ;
#29072=CARTESIAN_POINT ( 'NONE',  ( 0.02407890056655651728, -15.32140196853772984, 27.05343472112986092 ) ) ;
#29079=ORIENTED_EDGE ( 'NONE', *, *, #30128, .F. ) ;
#29081=CARTESIAN_POINT ( 'NONE',  ( 2.773602559888816987, 28.19409568634637964, -12.86837344186502818 ) ) ;
#29094=CARTESIAN_POINT ( 'NONE',  ( 0.000000000000000000, 25.67797970382135375, 16.40405592474768426 ) ) ;
#29101=VERTEX_POINT ( 'NONE', #12704 ) ;
#29105=ORIENTED_EDGE ( 'NONE', *, *, #29895, .T. ) ;
#29110=CYLINDRICAL_SURFACE ( 'NONE', #17792, 16.19999999999999929 ) ;
#29117=B_SPLINE_CURVE_WITH_KNOTS ( 'NONE', 3,
 ( #17258, #15278, #20604, #33956, #12084, #15101 ),
 .UNSPECIFIED., .F., .F.,
 ( 4, 2, 4 ),
 ( 2.036796643444265524E-07, 0.001873401978039416615, 0.003746600276414489058 ),
 .UNSPECIFIED. ) ;
#29127=CARTESIAN_POINT ( 'NONE',  ( 2.765921099433441555, -0.3931553186911057041, -31.08824725498900676 ) ) ;
#29128=VERTEX_POINT ( 'NONE', #20189 ) ;
#29129=CARTESIAN_POINT ( 'NONE',  ( 2.783107615553614078, -15.15194214258576011, -26.89541087693596211 ) ) ;
#29138=VERTEX_POINT ( 'NONE', #14684 ) ;
#29142=LINE ( 'NONE', #13316, #24150 ) ;
#29143=B_SPLINE_CURVE_WITH_KNOTS ( 'NONE', 3,
 ( #7423, #2266, #15464, #7598, #20796, #18318 ),
 .UNSPECIFIED., .F., .F.,
 ( 4, 2, 4 ),
 ( 4.404817164049666791E-07, 0.001874269726455598173, 0.003748098971194791310 ),
 .UNSPECIFIED. ) ;
#29149=DIRECTION ( 'NONE',  ( 0.000000000000000000, 0.000000000000000000, 1.000000000000000000 ) ) ;
#29151=CARTESIAN_POINT ( 'NONE',  ( 0.7564103408419841079, -24.35732449877335881, -23.60053042972057824 ) ) ;
#29163=ADVANCED_FACE ( 'NONE', ( #1139 ), #28368, .T. ) ;
#29175=TOROIDAL_SURFACE ( 'NONE', #30306, 30.47050528711512030, 8.000000000000000000 ) ;
#29199=VECTOR ( 'NONE', #9250, 1000.000000000000000 ) ;
#29205=FACE_OUTER_BOUND ( 'NONE', #28950, .T. ) ;
#29207=DIRECTION ( 'NONE',  ( -1.000000000000000000, -0.000000000000000000, -0.000000000000000000 ) ) ;
#29212=CARTESIAN_POINT ( 'NONE',  ( 2.897437953906695165E-16, -0.2191908000481288532, 30.66081142815914973 ) ) ;
#29219=CARTESIAN_POINT ( 'NONE',  ( 2.606461977389332940, 19.62374805819733581, 25.61906966869699431 ) ) ;
#29226=CARTESIAN_POINT ( 'NONE',  ( 8.000000000000000000, 0.000000000000000000, 0.000000000000000000 ) ) ;
#29228=LINE ( 'NONE', #4824, #15859 ) ;
#29229=CARTESIAN_POINT ( 'NONE',  ( 2.789999999999999147, 17.98401995359633077, 24.59729088254962548 ) ) ;
#29233=CARTESIAN_POINT ( 'NONE',  ( 0.5248942108473680923, 5.490830290250059420, -32.92508943594307880 ) ) ;
#29234=CARTESIAN_POINT ( 'NONE',  ( 2.787883829527677548, 27.86222219983571335, -12.86217335695008046 ) ) ;
#29238=ORIENTED_EDGE ( 'NONE', *, *, #18110, .F. ) ;
#29245=CARTESIAN_POINT ( 'NONE',  ( 2.789999999999999147, -29.69698570178027808, 11.75786841620004175 ) ) ;
#29248=EDGE_CURVE ( 'NONE', #23973, #17221, #20703, .T. ) ;
#29249=CARTESIAN_POINT ( 'NONE',  ( 2.033800788961415140, 21.20694131899045942, 26.46705060818966260 ) ) ;
#29264=DIRECTION ( 'NONE',  ( 0.000000000000000000, 0.000000000000000000, 1.000000000000000000 ) ) ;
#29266=B_SPLINE_CURVE_WITH_KNOTS ( 'NONE', 3,
 ( #31194, #1467, #17859, #6793 ),
 .UNSPECIFIED., .F., .F.,
 ( 4, 4 ),
 ( 2.436748180515341377E-07, 0.0006879797535939411769 ),
 .UNSPECIFIED. ) ;
#29277=CYLINDRICAL_SURFACE ( 'NONE', #19678, 16.19999999999999574 ) ;
#29279=CYLINDRICAL_SURFACE ( 'NONE', #22057, 2.524999999999999467 ) ;
#29282=DIRECTION ( 'NONE',  ( 1.000000000000000000, 0.000000000000000000, 0.000000000000000000 ) ) ;
#29285=DIRECTION ( 'NONE',  ( 0.000000000000000000, 0.000000000000000000, 1.000000000000000000 ) ) ;
#29291=CARTESIAN_POINT ( 'NONE',  ( 1.749999999999999778, -10.37741591188916424, 32.81304455236865181 ) ) ;
#29292=VERTEX_POINT ( 'NONE', #5361 ) ;
#29303=ORIENTED_EDGE ( 'NONE', *, *, #11773, .F. ) ;
#29309=B_SPLINE_CURVE_WITH_KNOTS ( 'NONE', 3,
 ( #20087, #30930, #8512, #6001, #2985, #686 ),
 .UNSPECIFIED., .F., .F.,
 ( 4, 2, 4 ),
 ( 4.404817102045565444E-07, 0.001874269680285066582, 0.003748098878859928897 ),
 .UNSPECIFIED. ) ;
#29311=ORIENTED_EDGE ( 'NONE', *, *, #1651, .F. ) ;
#29336=FACE_OUTER_BOUND ( 'NONE', #12927, .T. ) ;
#29345=VERTEX_POINT ( 'NONE', #10365 ) ;
#29359=CARTESIAN_POINT ( 'NONE',  ( 1.040000000000000924, 0.000000000000000000, 0.000000000000000000 ) ) ;
#29363=DIRECTION ( 'NONE',  ( 1.000000000000000000, 0.000000000000000000, 0.000000000000000000 ) ) ;
#29364=EDGE_CURVE ( 'NONE', #27823, #245, #8661, .T. ) ;
#29366=VECTOR ( 'NONE', #33121, 1000.000000000000000 ) ;
#29371=EDGE_LOOP ( 'NONE', ( #6190, #5954, #1166, #3876 ) ) ;
#29386=EDGE_CURVE ( 'NONE', #2950, #6306, #14234, .T. ) ;
#29394=B_SPLINE_CURVE_WITH_KNOTS ( 'NONE', 3,
 ( #4147, #15208, #12369, #12198 ),
 .UNSPECIFIED., .F., .F.,
 ( 4, 4 ),
 ( 0.005298392425857880068, 0.005985260475359764631 ),
 .UNSPECIFIED. ) ;
#29397=EDGE_LOOP ( 'NONE', ( #28060, #1187, #4175, #13996, #26764, #28809, #31713 ) ) ;
#29398=ORIENTED_EDGE ( 'NONE', *, *, #3652, .T. ) ;
#29406=ADVANCED_FACE ( 'NONE', ( #19624 ), #22107, .T. ) ;
#29407=CARTESIAN_POINT ( 'NONE',  ( 1.394999999999999574, -33.26546734453813059, -8.820166447042129931 ) ) ;
#29421=FACE_OUTER_BOUND ( 'NONE', #6739, .T. ) ;
#29427=DIRECTION ( 'NONE',  ( -1.000000000000000000, 0.000000000000000000, -0.000000000000000000 ) ) ;
#29436=CARTESIAN_POINT ( 'NONE',  ( 2.765921099433442887, -23.70329957282599764, 20.11932597908820242 ) ) ;
#29448=AXIS2_PLACEMENT_3D ( 'NONE', #30320, #28005, #14322 ) ;
#29457=LINE ( 'NONE', #2560, #34549 ) ;
#29458=CARTESIAN_POINT ( 'NONE',  ( 1.395000000000002238, -33.39989884085097316, 8.296590337300143503 ) ) ;
#29459=DIRECTION ( 'NONE',  ( 0.000000000000000000, -0.1253332335642985129, -0.9921147013144785420 ) ) ;
#29467=CYLINDRICAL_SURFACE ( 'NONE', #35088, 16.19999999999999929 ) ;
#29475=CARTESIAN_POINT ( 'NONE',  ( 0.000000000000000000, -3.728217946242704972, -30.24156218513559580 ) ) ;
#29511=CYLINDRICAL_SURFACE ( 'NONE', #17436, 2.525000000000001243 ) ;
#29517=CARTESIAN_POINT ( 'NONE',  ( 0.02407890056655781832, 31.00221527374952046, -2.344426712874310148 ) ) ;
#29524=CARTESIAN_POINT ( 'NONE',  ( 2.789999999999999147, -15.32140196853772984, 27.05343472112986092 ) ) ;
#29535=DIRECTION ( 'NONE',  ( -1.000000000000000000, 0.000000000000000000, -0.000000000000000000 ) ) ;
#29543=ORIENTED_EDGE ( 'NONE', *, *, #12271, .T. ) ;
#29546=ADVANCED_FACE ( 'NONE', ( #15330 ), #12484, .F. ) ;
#29550=CARTESIAN_POINT ( 'NONE',  ( 1.040000000000000924, 0.000000000000000000, 0.000000000000000000 ) ) ;
#29561=DIRECTION ( 'NONE',  ( -1.000000000000000000, -0.000000000000000000, -0.000000000000000000 ) ) ;
#29565=ORIENTED_EDGE ( 'NONE', *, *, #1510, .T. ) ;
#29570=EDGE_LOOP ( 'NONE', ( #20125, #32097, #14487, #4123 ) ) ;
#29575=ORIENTED_EDGE ( 'NONE', *, *, #16204, .F. ) ;
#29580=ORIENTED_EDGE ( 'NONE', *, *, #12797, .T. ) ;
#29584=CARTESIAN_POINT ( 'NONE',  ( 0.000000000000000000, 2.005524111408194088, 31.87689292423238996 ) ) ;
#29585=CARTESIAN_POINT ( 'NONE',  ( 1.394999999999999574, -10.37741591188871659, -32.81304455236878681 ) ) ;
#29595=DIRECTION ( 'NONE',  ( -1.000000000000000000, -0.000000000000000000, -0.000000000000000000 ) ) ;
#29603=EDGE_CURVE ( 'NONE', #13768, #29101, #27928, .T. ) ;
#29611=ORIENTED_EDGE ( 'NONE', *, *, #5899, .T. ) ;
#29625=DIRECTION ( 'NONE',  ( 0.000000000000000000, 0.000000000000000000, 1.000000000000000000 ) ) ;
#29627=ORIENTED_EDGE ( 'NONE', *, *, #12540, .F. ) ;
#29635=DIRECTION ( 'NONE',  ( -1.000000000000000000, 0.000000000000000000, 0.000000000000000000 ) ) ;
#29644=EDGE_CURVE ( 'NONE', #15534, #5282, #8339, .T. ) ;
#29649=B_SPLINE_CURVE_WITH_KNOTS ( 'NONE', 3,
 ( #14724, #12048, #20745, #18096, #17922, #17741 ),
 .UNSPECIFIED., .F., .F.,
 ( 4, 2, 4 ),
 ( 4.404817002931014679E-07, 0.001874269606490522972, 0.003748098731280752587 ),
 .UNSPECIFIED. ) ;
#29651=VERTEX_POINT ( 'NONE', #4605 ) ;
#29656=ORIENTED_EDGE ( 'NONE', *, *, #1959, .F. ) ;
#29661=CARTESIAN_POINT ( 'NONE',  ( 2.789999999999999591, -14.96303950468899480, -26.76267923430003393 ) ) ;
#29665=VERTEX_POINT ( 'NONE', #23496 ) ;
#29668=DIRECTION ( 'NONE',  ( -1.000000000000000000, -0.000000000000000000, -0.000000000000000000 ) ) ;
#29671=AXIS2_PLACEMENT_3D ( 'NONE', #15634, #18308, #12962 ) ;
#29672=DIRECTION ( 'NONE',  ( 0.000000000000000000, 0.000000000000000000, 1.000000000000000000 ) ) ;
#29677=CARTESIAN_POINT ( 'NONE',  ( 2.789999999999999147, -8.112136323389137260, 30.01377904834206589 ) ) ;
#29687=EDGE_CURVE ( 'NONE', #509, #19620, #10326, .T. ) ;
#29691=DIRECTION ( 'NONE',  ( -1.000000000000000000, 0.000000000000000000, -0.000000000000000000 ) ) ;
#29696=ORIENTED_EDGE ( 'NONE', *, *, #29824, .F. ) ;
#29701=AXIS2_PLACEMENT_3D ( 'NONE', #33053, #30045, #5638 ) ;
#29704=CARTESIAN_POINT ( 'NONE',  ( 0.000000000000000000, -25.77598557799239742, -16.24962337825829195 ) ) ;
#29705=CARTESIAN_POINT ( 'NONE',  ( 1.394999999999999574, 34.17636915695680244, -4.045051921974837761 ) ) ;
#29722=CARTESIAN_POINT ( 'NONE',  ( 1.749999999999999778, -24.90160365674886478, 23.75493189058330756 ) ) ;
#29726=DIRECTION ( 'NONE',  ( 1.000000000000000000, 0.000000000000000000, 0.000000000000000000 ) ) ;
#29727=EDGE_CURVE ( 'NONE', #17530, #22891, #28488, .T. ) ;
#29734=CYLINDRICAL_SURFACE ( 'NONE', #27362, 34.41491905851385269 ) ;
#29736=CARTESIAN_POINT ( 'NONE',  ( -5.210000000000000853, 0.000000000000000000, 0.000000000000000000 ) ) ;
#29738=ORIENTED_EDGE ( 'NONE', *, *, #28567, .T. ) ;
#29748=VERTEX_POINT ( 'NONE', #35073 ) ;
#29750=B_SPLINE_CURVE_WITH_KNOTS ( 'NONE', 3,
 ( #32510, #19716, #8135, #5281 ),
 .UNSPECIFIED., .F., .F.,
 ( 4, 4 ),
 ( 2.080333525987768553E-07, 0.0006879438135628904464 ),
 .UNSPECIFIED. ) ;
#29754=ORIENTED_EDGE ( 'NONE', *, *, #20498, .T. ) ;
#29766=DIRECTION ( 'NONE',  ( -1.000000000000000000, 0.000000000000000000, 0.000000000000000000 ) ) ;
#29773=CARTESIAN_POINT ( 'NONE',  ( -10.00000000000000000, 0.000000000000000000, 0.000000000000000000 ) ) ;
#29788=ORIENTED_EDGE ( 'NONE', *, *, #31875, .T. ) ;
#29791=EDGE_CURVE ( 'NONE', #24353, #22184, #25359, .T. ) ;
#29793=CARTESIAN_POINT ( 'NONE',  ( 2.789999999999999147, 26.03801215795517621, 16.98986790278620873 ) ) ;
#29797=FACE_OUTER_BOUND ( 'NONE', #33461, .T. ) ;
#29817=DIRECTION ( 'NONE',  ( 1.000000000000000000, 0.000000000000000000, 0.000000000000000000 ) ) ;
#29821=DIRECTION ( 'NONE',  ( 0.000000000000000000, 0.000000000000000000, 1.000000000000000000 ) ) ;
#29824=EDGE_CURVE ( 'NONE', #16094, #9347, #21671, .T. ) ;
#29830=EDGE_CURVE ( 'NONE', #1305, #7253, #853, .T. ) ;
#29832=CIRCLE ( 'NONE', #7079, 34.41491905851385269 ) ;
#29833=EDGE_LOOP ( 'NONE', ( #31025, #16599, #7564, #16739, #3567, #4083 ) ) ;
#29836=ORIENTED_EDGE ( 'NONE', *, *, #32339, .F. ) ;
#29837=ORIENTED_EDGE ( 'NONE', *, *, #2390, .F. ) ;
#29846=B_SPLINE_CURVE_WITH_KNOTS ( 'NONE', 3,
 ( #32725, #8349, #27738, #21217, #33074, #22405 ),
 .UNSPECIFIED., .F., .F.,
 ( 4, 2, 4 ),
 ( 4.404817209422835260E-07, 0.001874269760234689892, 0.003748099038748437580 ),
 .UNSPECIFIED. ) ;
#29856=ORIENTED_EDGE ( 'NONE', *, *, #11064, .F. ) ;
#29862=CARTESIAN_POINT ( 'NONE',  ( 0.000000000000000000, 0.000000000000000000, 0.000000000000000000 ) ) ;
#29870=DIRECTION ( 'NONE',  ( 0.000000000000000000, 0.000000000000000000, 1.000000000000000000 ) ) ;
#29873=CARTESIAN_POINT ( 'NONE',  ( 0.02407890056655825201, 14.63235270440936731, 27.43224275967444470 ) ) ;
#29874=CARTESIAN_POINT ( 'NONE',  ( 2.783128942445853404, -26.23443237966589692, 16.26905388445657508 ) ) ;
#29875=ORIENTED_EDGE ( 'NONE', *, *, #3094, .F. ) ;
#29879=DIRECTION ( 'NONE',  ( 1.000000000000000000, 0.000000000000000000, 0.000000000000000000 ) ) ;
#29881=EDGE_LOOP ( 'NONE', ( #32999, #30592, #1468, #33812 ) ) ;
#29895=EDGE_CURVE ( 'NONE', #30046, #21299, #22827, .T. ) ;
#29903=ORIENTED_EDGE ( 'NONE', *, *, #26483, .F. ) ;
#29904=EDGE_LOOP ( 'NONE', ( #25327, #32178, #27379, #1122 ) ) ;
#29908=VERTEX_POINT ( 'NONE', #706 ) ;
#29911=LINE ( 'NONE', #10865, #15474 ) ;
#29912=CARTESIAN_POINT ( 'NONE',  ( 0.1859802889711900942, -0.8217981779190254299, -32.27126551972443735 ) ) ;
#29917=CARTESIAN_POINT ( 'NONE',  ( 2.033800780627561533, 5.833185478271119884, 33.40977515897103700 ) ) ;
#29920=CARTESIAN_POINT ( 'NONE',  ( 0.7752961785294064656, 31.37228877271656913, 12.97290618475348012 ) ) ;
#29924=CIRCLE ( 'NONE', #8323, 30.47050528711511674 ) ;
#29931=EDGE_CURVE ( 'NONE', #29748, #8703, #7453, .T. ) ;
#29933=CARTESIAN_POINT ( 'NONE',  ( 2.789999999999999147, -3.728217946243117087, 30.24156218513554606 ) ) ;
#29936=CARTESIAN_POINT ( 'NONE',  ( 2.789999999999999147, 11.80989368511502846, -28.76039115933972923 ) ) ;
#29942=DIRECTION ( 'NONE',  ( 1.000000000000000000, 0.000000000000000000, 0.000000000000000000 ) ) ;
#29946=FACE_OUTER_BOUND ( 'NONE', #33633, .T. ) ;
#29952=DIRECTION ( 'NONE',  ( -1.000000000000000000, -0.000000000000000000, -0.000000000000000000 ) ) ;
#29953=CIRCLE ( 'NONE', #32230, 2.524999999999999467 ) ;
#29954=CARTESIAN_POINT ( 'NONE',  ( 2.765921099433442443, 7.350529080603967813, -30.20932655202929595 ) ) ;
#29955=ORIENTED_EDGE ( 'NONE', *, *, #14478, .T. ) ;
#29957=CARTESIAN_POINT ( 'NONE',  ( 2.789999999999999147, 18.59128259035506758, -24.91982945642901726 ) ) ;
#29972=ORIENTED_EDGE ( 'NONE', *, *, #4668, .T. ) ;
#29988=FACE_OUTER_BOUND ( 'NONE', #27475, .T. ) ;
#29996=CARTESIAN_POINT ( 'NONE',  ( 1.749999999999999778, -30.02688531850381182, -16.81585001935615153 ) ) ;
#30003=CARTESIAN_POINT ( 'NONE',  ( 2.033589659274374295, -32.97789401874100434, -7.919772684713185740 ) ) ;
#30022=DIRECTION ( 'NONE',  ( -1.000000000000000000, -0.000000000000000000, -0.000000000000000000 ) ) ;
#30026=ADVANCED_FACE ( 'NONE', ( #33798 ), #15469, .T. ) ;
#30030=VERTEX_POINT ( 'NONE', #12451 ) ;
#30033=EDGE_CURVE ( 'NONE', #2604, #5830, #23660, .T. ) ;
#30034=AXIS2_PLACEMENT_3D ( 'NONE', #29047, #10551, #7324 ) ;
#30036=ORIENTED_EDGE ( 'NONE', *, *, #28970, .T. ) ;
#30037=DIRECTION ( 'NONE',  ( 0.000000000000000000, 0.3681245526846860794, -0.9297764858882481276 ) ) ;
#30042=VERTEX_POINT ( 'NONE', #34136 ) ;
#30045=DIRECTION ( 'NONE',  ( -1.000000000000000000, -0.000000000000000000, -0.000000000000000000 ) ) ;
#30046=VERTEX_POINT ( 'NONE', #30774 ) ;
#30049=EDGE_CURVE ( 'NONE', #14706, #23769, #29143, .T. ) ;
#30054=CARTESIAN_POINT ( 'NONE',  ( 0.000000000000000000, 0.000000000000000000, 3.000000000000000000 ) ) ;
#30063=ORIENTED_EDGE ( 'NONE', *, *, #27407, .F. ) ;
#30065=ADVANCED_FACE ( 'NONE', ( #29336 ), #35034, .T. ) ;
#30073=EDGE_LOOP ( 'NONE', ( #12558, #3541, #19717, #10088 ) ) ;
#30078=ORIENTED_EDGE ( 'NONE', *, *, #26687, .F. ) ;
#30085=CIRCLE ( 'NONE', #27810, 2.524999999999999467 ) ;
#30092=CARTESIAN_POINT ( 'NONE',  ( 1.039999999999999591, 31.89769921722987434, 12.91988538846969803 ) ) ;
#30097=FACE_OUTER_BOUND ( 'NONE', #20148, .T. ) ;
#30108=FACE_OUTER_BOUND ( 'NONE', #25145, .T. ) ;
#30110=DIRECTION ( 'NONE',  ( 0.000000000000000000, -3.435095992033281961E-15, -1.000000000000000000 ) ) ;
#30112=CARTESIAN_POINT ( 'NONE',  ( 0.000000000000000000, 20.79173593595294633, -22.27454621808743340 ) ) ;
#30118=DIRECTION ( 'NONE',  ( 1.000000000000000000, 0.000000000000000000, 0.000000000000000000 ) ) ;
#30128=EDGE_CURVE ( 'NONE', #7115, #34482, #22264, .T. ) ;
#30137=B_SPLINE_CURVE_WITH_KNOTS ( 'NONE', 3,
 ( #26089, #1705, #15075, #31601, #12573, #6513 ),
 .UNSPECIFIED., .F., .F.,
 ( 4, 2, 4 ),
 ( 4.404817006176418240E-07, 0.001874269609036405965, 0.003748098736372194612 ),
 .UNSPECIFIED. ) ;
#30139=CYLINDRICAL_SURFACE ( 'NONE', #18836, 10.00000000000000000 ) ;
#30147=VECTOR ( 'NONE', #14505, 1000.000000000000000 ) ;
#30162=DIRECTION ( 'NONE',  ( 0.000000000000000000, 0.000000000000000000, 1.000000000000000000 ) ) ;
#30163=EDGE_CURVE ( 'NONE', #26980, #13600, #5801, .T. ) ;
#30169=EDGE_CURVE ( 'NONE', #10663, #22622, #25295, .T. ) ;
#30174=ORIENTED_EDGE ( 'NONE', *, *, #26634, .T. ) ;
#30181=DIRECTION ( 'NONE',  ( -1.000000000000000000, 0.000000000000000000, -0.000000000000000000 ) ) ;
#30199=DIRECTION ( 'NONE',  ( 0.000000000000000000, 0.000000000000000000, 1.000000000000000000 ) ) ;
#30201=CARTESIAN_POINT ( 'NONE',  ( 0.000000000000000000, -5.984944020945660803, -28.84917528048448787 ) ) ;
#30208=ORIENTED_EDGE ( 'NONE', *, *, #23153, .F. ) ;
#30211=CARTESIAN_POINT ( 'NONE',  ( 2.789999999999999147, -15.78270255339092287, 26.02842157509082455 ) ) ;
#30214=ORIENTED_EDGE ( 'NONE', *, *, #11503, .T. ) ;
#30218=CARTESIAN_POINT ( 'NONE',  ( 0.07098932344682959417, -31.66360817300142827, 1.400248398912060210 ) ) ;
#30230=DIRECTION ( 'NONE',  ( -1.000000000000000000, -0.000000000000000000, 0.000000000000000000 ) ) ;
#30232=CARTESIAN_POINT ( 'NONE',  ( 2.765921099433441999, -21.56796757982826307, 22.39322359481599278 ) ) ;
#30244=EDGE_CURVE ( 'NONE', #7395, #18440, #27389, .T. ) ;
#30249=DIRECTION ( 'NONE',  ( 0.000000000000000000, 0.000000000000000000, 1.000000000000000000 ) ) ;
#30251=ADVANCED_FACE ( 'NONE', ( #8315 ), #16521, .T. ) ;
#30261=EDGE_CURVE ( 'NONE', #26414, #19893, #33814, .T. ) ;
#30274=CARTESIAN_POINT ( 'NONE',  ( 1.749999999999999778, -18.66807150955433769, 28.91175816027496381 ) ) ;
#30283=EDGE_CURVE ( 'NONE', #32497, #19094, #13839, .T. ) ;
#30287=EDGE_CURVE ( 'NONE', #33511, #26400, #6179, .T. ) ;
#30292=DIRECTION ( 'NONE',  ( -1.000000000000000000, -0.000000000000000000, 0.000000000000000000 ) ) ;
#30295=DIRECTION ( 'NONE',  ( 0.000000000000000000, 0.000000000000000000, -1.000000000000000000 ) ) ;
#30306=AXIS2_PLACEMENT_3D ( 'NONE', #34059, #2187, #12715 ) ;
#30318=VERTEX_POINT ( 'NONE', #11521 ) ;
#30320=CARTESIAN_POINT ( 'NONE',  ( 0.000000000000000000, 31.93991905851385837, 0.000000000000000000 ) ) ;
#30321=B_SPLINE_CURVE_WITH_KNOTS ( 'NONE', 3,
 ( #27621, #5371, #13581, #2531, #8573, #5712 ),
 .UNSPECIFIED., .F., .F.,
 ( 4, 2, 4 ),
 ( 1.978909662040517630E-07, 0.001873396183027085504, 0.003746594475087967023 ),
 .UNSPECIFIED. ) ;
#30324=LINE ( 'NONE', #16833, #7440 ) ;
#30327=CARTESIAN_POINT ( 'NONE',  ( 2.789999999999999147, -25.83993731729808729, 18.77381338200959604 ) ) ;
#30331=EDGE_LOOP ( 'NONE', ( #28036, #22454, #4710, #5909 ) ) ;
#30336=DIRECTION ( 'NONE',  ( -1.000000000000000000, -0.000000000000000000, -0.000000000000000000 ) ) ;
#30342=CARTESIAN_POINT ( 'NONE',  ( 2.033800793007967123, 27.74641878906490788, -19.50321439924927702 ) ) ;
#30346=CARTESIAN_POINT ( 'NONE',  ( 2.789999999999999147, -30.41598411195407081, -1.821977758773984490 ) ) ;
#30349=B_SPLINE_CURVE_WITH_KNOTS ( 'NONE', 3,
 ( #33607, #1222, #33260, #28280 ),
 .UNSPECIFIED., .F., .F.,
 ( 4, 4 ),
 ( 0.005298346188946770341, 0.005985214897255175526 ),
 .UNSPECIFIED. ) ;
#30352=DIRECTION ( 'NONE',  ( 0.000000000000000000, 0.9980267284282708928, 0.06279051952932451774 ) ) ;
#30354=ORIENTED_EDGE ( 'NONE', *, *, #16342, .F. ) ;
#30358=CARTESIAN_POINT ( 'NONE',  ( 1.749999999999999778, -18.21166265554811403, 29.20140402659732359 ) ) ;
#30369=CARTESIAN_POINT ( 'NONE',  ( 1.395000000000002238, -1.891117961019738836, -34.36292081097834483 ) ) ;
#30373=CARTESIAN_POINT ( 'NONE',  ( 2.261199740935803781, 7.012902549146583731, 32.64503617578046857 ) ) ;
#30374=DIRECTION ( 'NONE',  ( 0.000000000000000000, 0.000000000000000000, 1.000000000000000000 ) ) ;
#30379=EDGE_CURVE ( 'NONE', #7570, #23345, #14287, .T. ) ;
#30381=CARTESIAN_POINT ( 'NONE',  ( -8.300095185491707450E-14, -14.96425809614971669, -26.76330950827351174 ) ) ;
#30388=CARTESIAN_POINT ( 'NONE',  ( 0.000000000000000000, 0.000000000000000000, 0.000000000000000000 ) ) ;
#30389=AXIS2_PLACEMENT_3D ( 'NONE', #10229, #3392, #22799 ) ;
#30393=CARTESIAN_POINT ( 'NONE',  ( 2.033589655458472034, -32.71412841873095090, 8.947071897914785410 ) ) ;
#30397=CARTESIAN_POINT ( 'NONE',  ( 1.040000000000000924, 0.000000000000000000, 0.000000000000000000 ) ) ;
#30400=VERTEX_POINT ( 'NONE', #30910 ) ;
#30403=VERTEX_POINT ( 'NONE', #17233 ) ;
#30405=CARTESIAN_POINT ( 'NONE',  ( 2.033589656346549202, -33.91140021655721881, 0.5303102773909653678 ) ) ;
#30410=ORIENTED_EDGE ( 'NONE', *, *, #4044, .T. ) ;
#30421=DIRECTION ( 'NONE',  ( 0.000000000000000000, 0.000000000000000000, 1.000000000000000000 ) ) ;
#30449=EDGE_CURVE ( 'NONE', #29651, #25284, #27811, .T. ) ;
#30457=CARTESIAN_POINT ( 'NONE',  ( 1.040000000000002034, 6.714005886384948774, 33.75364837705175347 ) ) ;
#30461=CARTESIAN_POINT ( 'NONE',  ( 1.394999999999999574, -18.21166265554809627, 29.20140402659733780 ) ) ;
#30474=ADVANCED_FACE ( 'NONE', ( #4363 ), #4700, .T. ) ;
#30475=ORIENTED_EDGE ( 'NONE', *, *, #9274, .T. ) ;
#30476=CIRCLE ( 'NONE', #4897, 2.525000000000001243 ) ;
#30477=CARTESIAN_POINT ( 'NONE',  ( 0.02407890056655738464, -11.07880054387200985, -29.04985141099774637 ) ) ;
#30479=EDGE_CURVE ( 'NONE', #13866, #7179, #5774, .T. ) ;
#30483=VECTOR ( 'NONE', #23579, 1000.000000000000000 ) ;
#30495=ORIENTED_EDGE ( 'NONE', *, *, #12208, .T. ) ;
#30497=ORIENTED_EDGE ( 'NONE', *, *, #25953, .T. ) ;
#30500=AXIS2_PLACEMENT_3D ( 'NONE', #24456, #16312, #21802 ) ;
#30501=EDGE_CURVE ( 'NONE', #28175, #30403, #3231, .T. ) ;
#30503=FACE_OUTER_BOUND ( 'NONE', #24629, .T. ) ;
#30516=CARTESIAN_POINT ( 'NONE',  ( 1.749999999999999778, -33.26546734453812348, -8.820166447042147695 ) ) ;
#30523=CARTESIAN_POINT ( 'NONE',  ( 0.000000000000000000, 9.539392014169456147, -3.000000000000000000 ) ) ;
#30529=FACE_OUTER_BOUND ( 'NONE', #4942, .T. ) ;
#30530=DIRECTION ( 'NONE',  ( 0.000000000000000000, 0.000000000000000000, 1.000000000000000000 ) ) ;
#30531=VERTEX_POINT ( 'NONE', #23771 ) ;
#30535=EDGE_CURVE ( 'NONE', #18033, #34278, #22294, .T. ) ;
#30538=AXIS2_PLACEMENT_3D ( 'NONE', #30954, #13227, #10735 ) ;
#30553=CARTESIAN_POINT ( 'NONE',  ( 2.765921099433441555, 11.80989368511502846, -28.76039115933972923 ) ) ;
#30559=VECTOR ( 'NONE', #25908, 1000.000000000000000 ) ;
#30561=ORIENTED_EDGE ( 'NONE', *, *, #28660, .F. ) ;
#30570=ORIENTED_EDGE ( 'NONE', *, *, #20487, .T. ) ;
#30573=ORIENTED_EDGE ( 'NONE', *, *, #10132, .T. ) ;
#30579=EDGE_CURVE ( 'NONE', #26431, #18208, #9231, .T. ) ;
#30592=ORIENTED_EDGE ( 'NONE', *, *, #7941, .T. ) ;
#30593=ORIENTED_EDGE ( 'NONE', *, *, #15719, .F. ) ;
#30597=CARTESIAN_POINT ( 'NONE',  ( 2.789999999999999147, 17.98401995359667893, -24.59729088254936613 ) ) ;
#30598=CARTESIAN_POINT ( 'NONE',  ( 0.000000000000000000, 14.59907093257252164, -26.74544485249453274 ) ) ;
#30601=CARTESIAN_POINT ( 'NONE',  ( 0.000000000000000000, 2.005524111408653720, -31.87689292423236154 ) ) ;
#30604=DIRECTION ( 'NONE',  ( -1.000000000000000000, -0.000000000000000000, -0.000000000000000000 ) ) ;
#30608=AXIS2_PLACEMENT_3D ( 'NONE', #28662, #32020, #6934 ) ;
#30610=ORIENTED_EDGE ( 'NONE', *, *, #28085, .F. ) ;
#30614=AXIS2_PLACEMENT_3D ( 'NONE', #33639, #25450, #19606 ) ;
#30617=CARTESIAN_POINT ( 'NONE',  ( 2.033800789375341367, 31.72496621377067427, -11.99023130257920045 ) ) ;
#30619=EDGE_CURVE ( 'NONE', #8440, #32621, #33367, .T. ) ;
#30632=EDGE_CURVE ( 'NONE', #19421, #31298, #15100, .T. ) ;
#30636=EDGE_CURVE ( 'NONE', #18981, #24353, #27302, .T. ) ;
#30641=VERTEX_POINT ( 'NONE', #24811 ) ;
#30647=VERTEX_POINT ( 'NONE', #18792 ) ;
#30653=DIRECTION ( 'NONE',  ( 0.000000000000000000, 0.000000000000000000, 1.000000000000000000 ) ) ;
#30654=DIRECTION ( 'NONE',  ( -1.000000000000000000, -0.000000000000000000, 0.000000000000000000 ) ) ;
#30655=CARTESIAN_POINT ( 'NONE',  ( 1.040000000000002034, 34.17636915695680244, 4.045051921974835096 ) ) ;
#30668=EDGE_CURVE ( 'NONE', #8703, #28747, #20639, .T. ) ;
#30673=ORIENTED_EDGE ( 'NONE', *, *, #7697, .T. ) ;
#30675=CIRCLE ( 'NONE', #27266, 2.524999999999999467 ) ;
#30679=ORIENTED_EDGE ( 'NONE', *, *, #24004, .T. ) ;
#30685=ADVANCED_FACE ( 'NONE', ( #29988, #11303 ), #10945, .F. ) ;
#30705=CARTESIAN_POINT ( 'NONE',  ( 2.783128833706969729, 11.66139262930099640, -28.58215465626852136 ) ) ;
#30708=CARTESIAN_POINT ( 'NONE',  ( -10.00000000000000000, 0.000000000000000000, 0.000000000000000000 ) ) ;
#30723=CARTESIAN_POINT ( 'NONE',  ( 0.006892394228582813739, 29.25821015115251811, 9.843862221888281638 ) ) ;
#30729=FACE_OUTER_BOUND ( 'NONE', #30073, .T. ) ;
#30732=CARTESIAN_POINT ( 'NONE',  ( 0.5248942696725308332, 30.74170660486493389, -13.00608379084241939 ) ) ;
#30734=CYLINDRICAL_SURFACE ( 'NONE', #5831, 2.524999999999999467 ) ;
#30747=ORIENTED_EDGE ( 'NONE', *, *, #2567, .F. ) ;
#30754=CARTESIAN_POINT ( 'NONE',  ( 2.789819856565905809, -25.83993731729781373, -16.24881338200996694 ) ) ;
#30765=CARTESIAN_POINT ( 'NONE',  ( -8.501468252432740527E-14, 14.57875922523702705, -26.97523840778871573 ) ) ;
#30768=CARTESIAN_POINT ( 'NONE',  ( 2.765921099433442887, -30.46391896562411716, 6.211548095912460710 ) ) ;
#30772=ADVANCED_FACE ( 'NONE', ( #27838 ), #28019, .F. ) ;
#30773=CARTESIAN_POINT ( 'NONE',  ( 2.765921099433442443, 30.61125888652969707, -5.439165181698684570 ) ) ;
#30774=CARTESIAN_POINT ( 'NONE',  ( 2.789999999999999147, -14.75935258146392570, -26.65732927035534772 ) ) ;
#30781=AXIS2_PLACEMENT_3D ( 'NONE', #14353, #25176, #5769 ) ;
#30783=EDGE_CURVE ( 'NONE', #24367, #16094, #12194, .T. ) ;
#30785=CARTESIAN_POINT ( 'NONE',  ( 2.783128948542799908, -11.06504178053264198, -28.81826507853140740 ) ) ;
#30789=CARTESIAN_POINT ( 'NONE',  ( 2.790000000000000924, 0.000000000000000000, 10.00000000000000000 ) ) ;
#30793=VERTEX_POINT ( 'NONE', #28378 ) ;
#30803=CIRCLE ( 'NONE', #15470, 34.41491905851385269 ) ;
#30806=TOROIDAL_SURFACE ( 'NONE', #17186, 30.47050528711511674, 8.000000000000000000 ) ;
#30810=FACE_OUTER_BOUND ( 'NONE', #10144, .T. ) ;
#30811=ORIENTED_EDGE ( 'NONE', *, *, #13779, .F. ) ;
#30815=CYLINDRICAL_SURFACE ( 'NONE', #15341, 16.19999999999999574 ) ;
#30819=CARTESIAN_POINT ( 'NONE',  ( 1.039999999999999813, -24.90160365674851661, -23.75493189058366994 ) ) ;
#30827=CARTESIAN_POINT ( 'NONE',  ( 0.7564103436534542757, -33.91140021655721881, -0.5303102773914404322 ) ) ;
#30833=CARTESIAN_POINT ( 'NONE',  ( 1.039999999999999147, -24.90160365674884346, 23.75493189058332177 ) ) ;
#30835=CARTESIAN_POINT ( 'NONE',  ( 0.000000000000000000, 11.30192140231230091, 28.29696565125076191 ) ) ;
#30836=EDGE_CURVE ( 'NONE', #26849, #5629, #2336, .T. ) ;
#30843=VERTEX_POINT ( 'NONE', #615 ) ;
#30849=CARTESIAN_POINT ( 'NONE',  ( 0.006871193125022706863, 29.25797949657101782, -9.843693408253376020 ) ) ;
#30852=VECTOR ( 'NONE', #31095, 1000.000000000000000 ) ;
#30869=EDGE_CURVE ( 'NONE', #21081, #18600, #34183, .T. ) ;
#30872=DIRECTION ( 'NONE',  ( 0.000000000000000000, 0.7705132427757948044, -0.6374239897486828621 ) ) ;
#30874=CARTESIAN_POINT ( 'NONE',  ( 2.790000000000083080, 11.49192876466753965, -28.42779197341999264 ) ) ;
#30886=ORIENTED_EDGE ( 'NONE', *, *, #1080, .F. ) ;
#30894=ADVANCED_FACE ( 'NONE', ( #14693 ), #16638, .T. ) ;
#30896=ORIENTED_EDGE ( 'NONE', *, *, #3548, .T. ) ;
#30905=CARTESIAN_POINT ( 'NONE',  ( 2.790000000000082636, 30.16006060148120582, -5.529416874851581731 ) ) ;
#30910=CARTESIAN_POINT ( 'NONE',  ( 0.000000000000000000, 9.869977788041397915, -27.85166815053926115 ) ) ;
#30916=ORIENTED_EDGE ( 'NONE', *, *, #19004, .F. ) ;
#30918=CARTESIAN_POINT ( 'NONE',  ( 2.765921099433442443, -30.46391896562403190, -6.211548095912885259 ) ) ;
#30923=CARTESIAN_POINT ( 'NONE',  ( 2.790000000000081304, -26.00660110917952750, 16.24378060718745687 ) ) ;
#30930=CARTESIAN_POINT ( 'NONE',  ( 0.7564103397028663078, -25.08336923281162001, 22.82737131378414119 ) ) ;
#30931=CIRCLE ( 'NONE', #32059, 34.41491905851385269 ) ;
#30944=CARTESIAN_POINT ( 'NONE',  ( 2.033589657508612536, 33.71046419695407081, 3.724096820061226332 ) ) ;
#30945=CARTESIAN_POINT ( 'NONE',  ( 0.02407890056655781832, 4.286445725888479608, -30.79383171238939809 ) ) ;
#30954=CARTESIAN_POINT ( 'NONE',  ( 2.789999999999999147, 0.000000000000000000, 0.000000000000000000 ) ) ;
#30959=CARTESIAN_POINT ( 'NONE',  ( 2.765921099433442887, -23.70329957282599764, 20.11932597908820242 ) ) ;
#30966=CARTESIAN_POINT ( 'NONE',  ( 2.606461982302225699, 30.42925477731488826, -10.74656554331663827 ) ) ;
#30971=ORIENTED_EDGE ( 'NONE', *, *, #19615, .F. ) ;
#30984=FACE_OUTER_BOUND ( 'NONE', #32808, .T. ) ;
#30994=CARTESIAN_POINT ( 'NONE',  ( 2.789999999999999147, 17.11426446101236820, -26.96776559937708129 ) ) ;
#30999=AXIS2_PLACEMENT_3D ( 'NONE', #6328, #25019, #30374 ) ;
#31007=CARTESIAN_POINT ( 'NONE',  ( 0.5248940958085364095, 13.50646231473678327, -30.52517305359770816 ) ) ;
#31008=CARTESIAN_POINT ( 'NONE',  ( 0.02407890056655695096, -21.56796757982826307, 22.39322359481599278 ) ) ;
#31011=CARTESIAN_POINT ( 'NONE',  ( 2.719010707633259916, -8.452877438714052616, -30.54658108095620861 ) ) ;
#31012=CARTESIAN_POINT ( 'NONE',  ( 0.7564103437026272747, -29.46130761496082329, -16.80165608683667955 ) ) ;
#31017=ORIENTED_EDGE ( 'NONE', *, *, #34159, .F. ) ;
#31023=B_SPLINE_CURVE_WITH_KNOTS ( 'NONE', 3,
 ( #25705, #30705, #30874, #9343 ),
 .UNSPECIFIED., .F., .F.,
 ( 4, 4 ),
 ( 3.087659402382905059E-07, 0.0006880453895801965291 ),
 .UNSPECIFIED. ) ;
#31025=ORIENTED_EDGE ( 'NONE', *, *, #29727, .T. ) ;
#31036=CARTESIAN_POINT ( 'NONE',  ( 0.07094831638746298963, -28.42120447776880354, 14.02663268823279630 ) ) ;
#31047=CARTESIAN_POINT ( 'NONE',  ( 0.02407890056655521624, 28.29688452313399338, 12.88099432405614309 ) ) ;
#31056=LINE ( 'NONE', #3977, #14457 ) ;
#31064=VERTEX_POINT ( 'NONE', #22245 ) ;
#31074=CARTESIAN_POINT ( 'NONE',  ( 2.033589658210382733, 22.02455111472429650, 25.79115045147389296 ) ) ;
#31078=EDGE_CURVE ( 'NONE', #30843, #26104, #32912, .T. ) ;
#31081=ORIENTED_EDGE ( 'NONE', *, *, #26682, .F. ) ;
#31092=CARTESIAN_POINT ( 'NONE',  ( 0.000000000000000000, -30.41598411195412055, 1.821977758773545952 ) ) ;
#31095=DIRECTION ( 'NONE',  ( -1.000000000000000000, -0.000000000000000000, 0.000000000000000000 ) ) ;
#31099=CARTESIAN_POINT ( 'NONE',  ( 2.765921099433441999, -3.506335382740735529, 30.89238256715863784 ) ) ;
#31100=DIRECTION ( 'NONE',  ( -1.000000000000000000, 0.000000000000000000, -0.000000000000000000 ) ) ;
#31106=CARTESIAN_POINT ( 'NONE',  ( 0.02407890056655608360, -31.05158812718222450, 1.559667679918499417 ) ) ;
#31107=CARTESIAN_POINT ( 'NONE',  ( 1.749999999999999778, 14.40815186467775888, 31.25366880301323746 ) ) ;
#31110=VECTOR ( 'NONE', #3474, 1000.000000000000000 ) ;
#31111=CYLINDRICAL_SURFACE ( 'NONE', #15928, 34.41491905851385269 ) ;
#31112=B_SPLINE_CURVE_WITH_KNOTS ( 'NONE', 3,
 ( #20521, #12001, #28538, #20184, #31036, #9836 ),
 .UNSPECIFIED., .F., .F.,
 ( 4, 2, 4 ),
 ( 4.404817209449920197E-07, 0.001874269760234692061, 0.003748099038748438881 ),
 .UNSPECIFIED. ) ;
#31127=AXIS2_PLACEMENT_3D ( 'NONE', #405, #930, #30653 ) ;
#31136=CARTESIAN_POINT ( 'NONE',  ( 2.719010744112896116, -15.78394019282702132, -27.48475859319554715 ) ) ;
#31147=CARTESIAN_POINT ( 'NONE',  ( 2.789999999999999147, 30.93646776788796160, 7.943134866716423659 ) ) ;
#31149=EDGE_CURVE ( 'NONE', #21389, #31871, #21010, .T. ) ;
#31160=ORIENTED_EDGE ( 'NONE', *, *, #19594, .F. ) ;
#31164=CYLINDRICAL_SURFACE ( 'NONE', #2744, 16.19999999999999574 ) ;
#31175=ORIENTED_EDGE ( 'NONE', *, *, #13740, .T. ) ;
#31179=AXIS2_PLACEMENT_3D ( 'NONE', #23880, #2698, #10727 ) ;
#31184=CARTESIAN_POINT ( 'NONE',  ( 0.000000000000000000, -11.13185981125856294, -28.36429779836965182 ) ) ;
#31186=ORIENTED_EDGE ( 'NONE', *, *, #26993, .F. ) ;
#31192=ORIENTED_EDGE ( 'NONE', *, *, #163, .F. ) ;
#31194=CARTESIAN_POINT ( 'NONE',  ( 0.02407890056655781832, 18.59128259035472297, 24.91982945642928016 ) ) ;
#31198=CARTESIAN_POINT ( 'NONE',  ( 0.000000000000000000, 0.000000000000000000, 0.000000000000000000 ) ) ;
#31212=DIRECTION ( 'NONE',  ( -1.000000000000000000, -0.000000000000000000, -0.000000000000000000 ) ) ;
#31215=VERTEX_POINT ( 'NONE', #22950 ) ;
#31217=CARTESIAN_POINT ( 'NONE',  ( 0.006892382889170392546, 23.98878059851183764, -19.42891868047383142 ) ) ;
#31220=CARTESIAN_POINT ( 'NONE',  ( 0.006892381134854739730, -23.57982834652831627, -19.92325699910571046 ) ) ;
#31225=CARTESIAN_POINT ( 'NONE',  ( 2.033589656860156136, -1.600050605840442008, 33.87778227150285915 ) ) ;
#31230=CARTESIAN_POINT ( 'NONE',  ( 0.5288002579745525455, -2.866095775114346988, 33.26657006572082054 ) ) ;
#31240=CARTESIAN_POINT ( 'NONE',  ( 0.5288002558916620188, -18.53787122671754162, 27.77096539590122504 ) ) ;
#31243=CARTESIAN_POINT ( 'NONE',  ( 2.789999999999999147, 9.869977788041397915, -27.85166815053926115 ) ) ;
#31249=CARTESIAN_POINT ( 'NONE',  ( 2.789999999999999147, 0.000000000000000000, 0.000000000000000000 ) ) ;
#31251=AXIS2_PLACEMENT_3D ( 'NONE', #11902, #17250, #33245 ) ;
#31255=CARTESIAN_POINT ( 'NONE',  ( 0.006892384446387221988, -15.15194214258620242, 26.89541087693579868 ) ) ;
#31261=CARTESIAN_POINT ( 'NONE',  ( 2.789999999999999147, 17.98401995359633077, 24.59729088254962548 ) ) ;
#31266=DIRECTION ( 'NONE',  ( 0.000000000000000000, 0.000000000000000000, 1.000000000000000000 ) ) ;
#31267=EDGE_CURVE ( 'NONE', #14449, #8838, #14948, .T. ) ;
#31270=EDGE_CURVE ( 'NONE', #28601, #17012, #14383, .T. ) ;
#31271=CARTESIAN_POINT ( 'NONE',  ( 2.789999999999999147, -11.13185981125856827, -28.36429779836962339 ) ) ;
#31274=ORIENTED_EDGE ( 'NONE', *, *, #719, .F. ) ;
#31276=B_SPLINE_CURVE_WITH_KNOTS ( 'NONE', 3,
 ( #3138, #483, #11344, #22189, #33028, #8653 ),
 .UNSPECIFIED., .F., .F.,
 ( 4, 2, 4 ),
 ( 4.404817011192420828E-07, 0.001874269612720305071, 0.003748098743739490622 ),
 .UNSPECIFIED. ) ;
#31279=ORIENTED_EDGE ( 'NONE', *, *, #12702, .F. ) ;
#31295=AXIS2_PLACEMENT_3D ( 'NONE', #12957, #26461, #2085 ) ;
#31298=VERTEX_POINT ( 'NONE', #20456 ) ;
#31299=CARTESIAN_POINT ( 'NONE',  ( 2.261199752785263861, -24.86182815675638835, -22.28830832814908547 ) ) ;
#31304=EDGE_CURVE ( 'NONE', #5389, #9440, #12106, .T. ) ;
#31315=AXIS2_PLACEMENT_3D ( 'NONE', #16464, #24266, #71 ) ;
#31322=EDGE_CURVE ( 'NONE', #13445, #1771, #3595, .T. ) ;
#31334=DIRECTION ( 'NONE',  ( 0.000000000000000000, 0.000000000000000000, 1.000000000000000000 ) ) ;
#31338=B_SPLINE_CURVE_WITH_KNOTS ( 'NONE', 3,
 ( #698, #33432, #19919, #14236 ),
 .UNSPECIFIED., .F., .F.,
 ( 4, 4 ),
 ( 2.335573237721180036E-07, 0.0006879695513619570393 ),
 .UNSPECIFIED. ) ;
#31341=LINE ( 'NONE', #6946, #9740 ) ;
#31344=CARTESIAN_POINT ( 'NONE',  ( 2.719010671502130272, 31.23843357299755041, 5.357709411917663367 ) ) ;
#31350=CARTESIAN_POINT ( 'NONE',  ( 0.07094833869610567278, -27.07192087577299588, -16.48097105307910581 ) ) ;
#31357=AXIS2_PLACEMENT_3D ( 'NONE', #5851, #14250, #8712 ) ;
#31361=VERTEX_POINT ( 'NONE', #28982 ) ;
#31370=CARTESIAN_POINT ( 'NONE',  ( 0.07094833594414887146, 24.79283726477109084, 19.74402504231806077 ) ) ;
#31373=CARTESIAN_POINT ( 'NONE',  ( 2.789999999999999147, -29.91351748324107263, 5.799410679710522487 ) ) ;
#31377=CARTESIAN_POINT ( 'NONE',  ( 1.395000000000002238, -30.28730148581174220, 16.34215476954022961 ) ) ;
#31384=ORIENTED_EDGE ( 'NONE', *, *, #15999, .F. ) ;
#31387=B_SPLINE_CURVE_WITH_KNOTS ( 'NONE', 3,
 ( #6822, #22866, #17191, #22331, #33710, #33894 ),
 .UNSPECIFIED., .F., .F.,
 ( 4, 2, 4 ),
 ( 2.178692865977853586E-07, 0.001873416183138251236, 0.003746614496989904633 ),
 .UNSPECIFIED. ) ;
#31399=VERTEX_POINT ( 'NONE', #26837 ) ;
#31401=CARTESIAN_POINT ( 'NONE',  ( -10.00000000000000000, 0.000000000000000000, 0.000000000000000000 ) ) ;
#31402=EDGE_CURVE ( 'NONE', #23546, #6373, #26930, .T. ) ;
#31408=CARTESIAN_POINT ( 'NONE',  ( 2.765921099433440666, -11.07880054387200985, -29.04985141099774637 ) ) ;
#31426=CARTESIAN_POINT ( 'NONE',  ( 0.7561992231261003283, -18.61835568386921835, -28.34776818504862916 ) ) ;
#31440=FACE_OUTER_BOUND ( 'NONE', #27484, .T. ) ;
#31445=ORIENTED_EDGE ( 'NONE', *, *, #20144, .F. ) ;
#31446=CARTESIAN_POINT ( 'NONE',  ( 2.789999999999999591, -0.2191908000477053864, -30.66081142815918170 ) ) ;
#31458=ORIENTED_EDGE ( 'NONE', *, *, #33292, .T. ) ;
#31459=AXIS2_PLACEMENT_3D ( 'NONE', #32745, #32388, #8367 ) ;
#31468=VERTEX_POINT ( 'NONE', #10287 ) ;
#31475=VERTEX_POINT ( 'NONE', #17060 ) ;
#31477=CARTESIAN_POINT ( 'NONE',  ( 2.783128945346505567, 14.58967697705802813, 27.20420702726705642 ) ) ;
#31482=CARTESIAN_POINT ( 'NONE',  ( -8.245173163873238465E-14, -0.2199561701056887975, -30.66195251245371622 ) ) ;
#31494=LINE ( 'NONE', #12649, #12358 ) ;
#31496=EDGE_CURVE ( 'NONE', #28354, #21081, #5855, .T. ) ;
#31497=VERTEX_POINT ( 'NONE', #31107 ) ;
#31499=CARTESIAN_POINT ( 'NONE',  ( 2.719010673589308258, -3.385659728284398540, 31.51320498992184227 ) ) ;
#31506=CARTESIAN_POINT ( 'NONE',  ( 2.789999999999999147, -31.05158812718220673, -1.559667679918931738 ) ) ;
#31508=B_SPLINE_CURVE_WITH_KNOTS ( 'NONE', 3,
 ( #27524, #21655, #30373, #2608, #21828, #32683 ),
 .UNSPECIFIED., .F., .F.,
 ( 4, 2, 4 ),
 ( 4.404817003536901581E-07, 0.001874269606490584555, 0.003748098731280815471 ),
 .UNSPECIFIED. ) ;
#31509=CARTESIAN_POINT ( 'NONE',  ( 0.02407890056655564992, 31.00221527374952046, 2.344426712874309260 ) ) ;
#31523=CARTESIAN_POINT ( 'NONE',  ( 0.5248941635506316761, -9.574141296992504380, 31.97728166840266439 ) ) ;
#31528=ORIENTED_EDGE ( 'NONE', *, *, #31496, .F. ) ;
#31530=ORIENTED_EDGE ( 'NONE', *, *, #17337, .F. ) ;
#31533=ORIENTED_EDGE ( 'NONE', *, *, #35018, .F. ) ;
#31535=ORIENTED_EDGE ( 'NONE', *, *, #24185, .F. ) ;
#31538=AXIS2_PLACEMENT_3D ( 'NONE', #21033, #7671, #34928 ) ;
#31545=EDGE_CURVE ( 'NONE', #10504, #29101, #25762, .T. ) ;
#31550=CARTESIAN_POINT ( 'NONE',  ( 1.395000000000002238, 22.14447232807545163, -26.34405054495533349 ) ) ;
#31564=CARTESIAN_POINT ( 'NONE',  ( 2.604019713477800035, 25.38927130757801010, -19.93727243998111476 ) ) ;
#31581=EDGE_LOOP ( 'NONE', ( #34378, #18011, #27676, #8743, #17352, #11179, #25444 ) ) ;
#31586=CARTESIAN_POINT ( 'NONE',  ( 1.040000000000000924, 0.000000000000000000, 0.000000000000000000 ) ) ;
#31595=ORIENTED_EDGE ( 'NONE', *, *, #29364, .F. ) ;
#31598=CARTESIAN_POINT ( 'NONE',  ( -5.018880456227426877E-16, -21.14855567236476119, 22.20072382163045077 ) ) ;
#31601=CARTESIAN_POINT ( 'NONE',  ( 0.1859802940384192305, 31.85364232850768218, 5.239790278973186055 ) ) ;
#31606=ORIENTED_EDGE ( 'NONE', *, *, #34508, .T. ) ;
#31611=EDGE_CURVE ( 'NONE', #13324, #29345, #34875, .T. ) ;
#31615=CARTESIAN_POINT ( 'NONE',  ( 1.394999999999999574, -25.27164158951551087, -23.36088151536946000 ) ) ;
#31622=VERTEX_POINT ( 'NONE', #31261 ) ;
#31627=CARTESIAN_POINT ( 'NONE',  ( 0.5288002541271116241, 33.21438043751174973, -3.418204286533154335 ) ) ;
#31635=DIRECTION ( 'NONE',  ( 0.000000000000000000, 0.000000000000000000, -1.000000000000000000 ) ) ;
#31640=CARTESIAN_POINT ( 'NONE',  ( 0.006871126357153574046, -15.15173253686488053, -26.89521541643909330 ) ) ;
#31649=FACE_OUTER_BOUND ( 'NONE', #10610, .T. ) ;
#31657=ORIENTED_EDGE ( 'NONE', *, *, #31784, .T. ) ;
#31661=AXIS2_PLACEMENT_3D ( 'NONE', #6240, #20324, #28503 ) ;
#31667=DIRECTION ( 'NONE',  ( -1.000000000000000000, 0.000000000000000000, 0.000000000000000000 ) ) ;
#31669=ORIENTED_EDGE ( 'NONE', *, *, #18983, .T. ) ;
#31674=CARTESIAN_POINT ( 'NONE',  ( 0.000000000000000000, -20.92506858792743785, -22.14933852381697932 ) ) ;
#31690=DIRECTION ( 'NONE',  ( 0.000000000000000000, 0.000000000000000000, -1.000000000000000000 ) ) ;
#31700=EDGE_CURVE ( 'NONE', #21389, #11399, #32562, .T. ) ;
#31703=EDGE_LOOP ( 'NONE', ( #34318, #7974, #3308, #17442 ) ) ;
#31708=AXIS2_PLACEMENT_3D ( 'NONE', #35076, #24197, #13186 ) ;
#31711=CARTESIAN_POINT ( 'NONE',  ( 2.783107610007986121, 14.58972988903205525, -27.20448975989763696 ) ) ;
#31713=ORIENTED_EDGE ( 'NONE', *, *, #17853, .F. ) ;
#31714=ORIENTED_EDGE ( 'NONE', *, *, #16566, .T. ) ;
#31720=CARTESIAN_POINT ( 'NONE',  ( 0.000000000000000000, 28.95078156989558948, 9.502838467758177643 ) ) ;
#31726=CARTESIAN_POINT ( 'NONE',  ( -5.210000000000000853, 0.000000000000000000, 0.000000000000000000 ) ) ;
#31728=TOROIDAL_SURFACE ( 'NONE', #11941, 30.47050528711512030, 8.000000000000000000 ) ;
#31731=CARTESIAN_POINT ( 'NONE',  ( 8.000000000000000000, 0.000000000000000000, 0.000000000000000000 ) ) ;
#31732=AXIS2_PLACEMENT_3D ( 'NONE', #3748, #915, #33473 ) ;
#31743=VECTOR ( 'NONE', #28239, 1000.000000000000000 ) ;
#31744=EDGE_LOOP ( 'NONE', ( #20252, #11993, #7860, #8954 ) ) ;
#31747=ORIENTED_EDGE ( 'NONE', *, *, #14919, .T. ) ;
#31748=B_SPLINE_CURVE_WITH_KNOTS ( 'NONE', 3,
 ( #12111, #25967, #28985, #7258, #34145, #9604 ),
 .UNSPECIFIED., .F., .F.,
 ( 4, 2, 4 ),
 ( 4.404817204574324437E-07, 0.001874269756547609737, 0.003748099031374762125 ),
 .UNSPECIFIED. ) ;
#31749=CARTESIAN_POINT ( 'NONE',  ( 1.040000000000002034, 34.17636915695680244, 4.045051921974835096 ) ) ;
#31754=ORIENTED_EDGE ( 'NONE', *, *, #11866, .F. ) ;
#31756=DIRECTION ( 'NONE',  ( -1.000000000000000000, -0.000000000000000000, -0.000000000000000000 ) ) ;
#31757=LINE ( 'NONE', #16423, #11819 ) ;
#31765=AXIS2_PLACEMENT_3D ( 'NONE', #22357, #33204, #27861 ) ;
#31779=ORIENTED_EDGE ( 'NONE', *, *, #32605, .T. ) ;
#31784=EDGE_CURVE ( 'NONE', #7014, #31468, #17836, .T. ) ;
#31786=B_SPLINE_CURVE_WITH_KNOTS ( 'NONE', 3,
 ( #11692, #3657, #17044, #27692, #22544, #33388 ),
 .UNSPECIFIED., .F., .F.,
 ( 4, 2, 4 ),
 ( 4.404817080791679206E-07, 0.001874269664496251448, 0.003748098847284423666 ),
 .UNSPECIFIED. ) ;
#31787=CARTESIAN_POINT ( 'NONE',  ( 2.765921099433441999, -15.32140196853772984, 27.05343472112986092 ) ) ;
#31795=VECTOR ( 'NONE', #9040, 1000.000000000000000 ) ;
#31801=ORIENTED_EDGE ( 'NONE', *, *, #11866, .T. ) ;
#31812=DIRECTION ( 'NONE',  ( -1.000000000000000000, 0.000000000000000000, 0.000000000000000000 ) ) ;
#31816=ORIENTED_EDGE ( 'NONE', *, *, #31611, .T. ) ;
#31817=DIRECTION ( 'NONE',  ( 0.000000000000000000, 0.000000000000000000, 1.000000000000000000 ) ) ;
#31829=DIRECTION ( 'NONE',  ( 0.000000000000000000, 0.000000000000000000, 1.000000000000000000 ) ) ;
#31831=ORIENTED_EDGE ( 'NONE', *, *, #10125, .F. ) ;
#31837=CARTESIAN_POINT ( 'NONE',  ( 2.265105736952408133, -2.869810969761243502, 33.25620129461680818 ) ) ;
#31839=ORIENTED_EDGE ( 'NONE', *, *, #3366, .F. ) ;
#31842=PRODUCT_DEFINITION ( 'UNKNOWN', '', #11032, #7847 ) ;
#31843=CARTESIAN_POINT ( 'NONE',  ( -1.791748084920704960E-16, 30.58654839005191661, 2.143968220813881942 ) ) ;
#31846=DIRECTION ( 'NONE',  ( -1.000000000000000000, 0.000000000000000000, 0.000000000000000000 ) ) ;
#31852=DIRECTION ( 'NONE',  ( 0.000000000000000000, 0.000000000000000000, 1.000000000000000000 ) ) ;
#31855=LINE ( 'NONE', #1624, #10478 ) ;
#31858=CARTESIAN_POINT ( 'NONE',  ( 2.719010691449824879, 4.557722287734057076, 31.36513882472106474 ) ) ;
#31864=B_SPLINE_CURVE_WITH_KNOTS ( 'NONE', 3,
 ( #11611, #30218, #16541, #507, #2640, #13508 ),
 .UNSPECIFIED., .F., .F.,
 ( 4, 2, 4 ),
 ( 2.040444213405217924E-07, 0.001873402343194273921, 0.003746600641967207362 ),
 .UNSPECIFIED. ) ;
#31871=VERTEX_POINT ( 'NONE', #34997 ) ;
#31875=EDGE_CURVE ( 'NONE', #23345, #30647, #7563, .T. ) ;
#31880=CARTESIAN_POINT ( 'NONE',  ( 1.040000000000001590, -33.39989884085085947, -8.296590337300607132 ) ) ;
#31884=DIRECTION ( 'NONE',  ( -1.000000000000000000, 0.000000000000000000, 0.000000000000000000 ) ) ;
#31892=CARTESIAN_POINT ( 'NONE',  ( 1.040000000000001146, -25.27164158951551087, -23.36088151536945645 ) ) ;
#31899=AXIS2_PLACEMENT_3D ( 'NONE', #7114, #9462, #9629 ) ;
#31914=CARTESIAN_POINT ( 'NONE',  ( 2.790000000000081748, -29.22921979676814175, 9.265873697118957253 ) ) ;
#31921=AXIS2_PLACEMENT_3D ( 'NONE', #6562, #15119, #17457 ) ;
#31925=AXIS2_PLACEMENT_3D ( 'NONE', #8501, #13334, #24164 ) ;
#31938=FACE_OUTER_BOUND ( 'NONE', #462, .T. ) ;
#31945=ORIENTED_EDGE ( 'NONE', *, *, #3451, .T. ) ;
#31949=DIRECTION ( 'NONE',  ( -1.000000000000000000, -0.000000000000000000, -0.000000000000000000 ) ) ;
#31950=CARTESIAN_POINT ( 'NONE',  ( 1.040000000000001146, -2.430610048906252985, 34.32897884578299852 ) ) ;
#31951=ADVANCED_FACE ( 'NONE', ( #21628 ), #205, .T. ) ;
#31958=DIRECTION ( 'NONE',  ( -1.000000000000000000, 0.000000000000000000, 0.000000000000000000 ) ) ;
#31976=DIRECTION ( 'NONE',  ( -1.000000000000000000, 0.000000000000000000, -0.000000000000000000 ) ) ;
#31979=DIRECTION ( 'NONE',  ( 0.000000000000000000, 0.000000000000000000, 1.000000000000000000 ) ) ;
#31984=CARTESIAN_POINT ( 'NONE',  ( -8.191443212915034962E-14, -27.65011189337360520, 13.25424764731395655 ) ) ;
#31986=DIRECTION ( 'NONE',  ( 0.000000000000000000, 0.000000000000000000, 1.000000000000000000 ) ) ;
#31988=CARTESIAN_POINT ( 'NONE',  ( 2.789999999999999147, 30.93646776788807173, -7.943134866715984899 ) ) ;
#31998=DIRECTION ( 'NONE',  ( 0.000000000000000000, 0.000000000000000000, -1.000000000000000000 ) ) ;
#32009=DIRECTION ( 'NONE',  ( -1.000000000000000000, -0.000000000000000000, 0.000000000000000000 ) ) ;
#32013=CARTESIAN_POINT ( 'NONE',  ( 5.048285286872369737E-16, -27.64940622781549351, -13.25307083675178887 ) ) ;
#32020=DIRECTION ( 'NONE',  ( -1.000000000000000000, 0.000000000000000000, -0.000000000000000000 ) ) ;
#32021=EDGE_LOOP ( 'NONE', ( #20515, #28860, #18040, #19777 ) ) ;
#32027=ORIENTED_EDGE ( 'NONE', *, *, #18707, .T. ) ;
#32034=EDGE_CURVE ( 'NONE', #7089, #29651, #5878, .T. ) ;
#32037=FACE_OUTER_BOUND ( 'NONE', #25510, .T. ) ;
#32039=DIRECTION ( 'NONE',  ( 1.000000000000000000, 0.000000000000000000, 0.000000000000000000 ) ) ;
#32041=CARTESIAN_POINT ( 'NONE',  ( 0.01077896562537771982, 28.09136514857379296, -12.86217335695005559 ) ) ;
#32042=FACE_OUTER_BOUND ( 'NONE', #6800, .T. ) ;
#32044=ADVANCED_FACE ( 'NONE', ( #5420 ), #16309, .T. ) ;
#32055=ORIENTED_EDGE ( 'NONE', *, *, #9768, .F. ) ;
#32059=AXIS2_PLACEMENT_3D ( 'NONE', #32799, #422, #19296 ) ;
#32075=DIRECTION ( 'NONE',  ( 1.000000000000000000, 0.000000000000000000, -0.000000000000000000 ) ) ;
#32083=ADVANCED_FACE ( 'NONE', ( #25165 ), #22518, .T. ) ;
#32097=ORIENTED_EDGE ( 'NONE', *, *, #30128, .T. ) ;
#32102=CIRCLE ( 'NONE', #7074, 2.524999999999999911 ) ;
#32105=AXIS2_PLACEMENT_3D ( 'NONE', #30388, #22379, #3847 ) ;
#32111=CARTESIAN_POINT ( 'NONE',  ( 0.02407890056655781832, 7.350529080603967813, -30.20932655202929595 ) ) ;
#32117=ORIENTED_EDGE ( 'NONE', *, *, #19889, .F. ) ;
#32123=CARTESIAN_POINT ( 'NONE',  ( 2.604019726408915769, -8.821517218320241938, 31.05303142369421465 ) ) ;
#32127=AXIS2_PLACEMENT_3D ( 'NONE', #21486, #32327, #16335 ) ;
#32129=CARTESIAN_POINT ( 'NONE',  ( 1.395000000000002238, 31.89769921723006263, -12.91988538846923973 ) ) ;
#32130=ORIENTED_EDGE ( 'NONE', *, *, #17902, .F. ) ;
#32131=CARTESIAN_POINT ( 'NONE',  ( 0.2014843505975234261, 29.63244935463695739, 13.00174666746673324 ) ) ;
#32132=CARTESIAN_POINT ( 'NONE',  ( 0.000000000000000000, 9.869977788041397915, -30.37666815053925973 ) ) ;
#32137=TOROIDAL_SURFACE ( 'NONE', #20765, 30.47050528711512030, 8.000000000000000000 ) ;
#32139=DIRECTION ( 'NONE',  ( 0.000000000000000000, 0.000000000000000000, 1.000000000000000000 ) ) ;
#32140=CARTESIAN_POINT ( 'NONE',  ( 1.749999999999999778, 28.00026196654270905, 20.00929742917132970 ) ) ;
#32143=ADVANCED_FACE ( 'NONE', ( #12371 ), #24630, .T. ) ;
#32150=ORIENTED_EDGE ( 'NONE', *, *, #25780, .F. ) ;
#32160=FACE_OUTER_BOUND ( 'NONE', #33832, .T. ) ;
#32162=EDGE_CURVE ( 'NONE', #29128, #27741, #12895, .T. ) ;
#32169=B_SPLINE_CURVE_WITH_KNOTS ( 'NONE', 3,
 ( #26728, #34934, #26379, #7501 ),
 .UNSPECIFIED., .F., .F.,
 ( 4, 4 ),
 ( 4.608367445541821421E-07, 0.0006881987313283487910 ),
 .UNSPECIFIED. ) ;
#32178=ORIENTED_EDGE ( 'NONE', *, *, #23425, .T. ) ;
#32189=EDGE_CURVE ( 'NONE', #33069, #21781, #23048, .T. ) ;
#32200=ORIENTED_EDGE ( 'NONE', *, *, #29364, .T. ) ;
#32203=DIRECTION ( 'NONE',  ( 0.000000000000000000, 0.000000000000000000, 1.000000000000000000 ) ) ;
#32210=CARTESIAN_POINT ( 'NONE',  ( 2.783128945071976723, -3.550602046213238161, -30.66465032581545103 ) ) ;
#32222=DIRECTION ( 'NONE',  ( -1.000000000000000000, -0.000000000000000000, 0.000000000000000000 ) ) ;
#32225=B_SPLINE_CURVE_WITH_KNOTS ( 'NONE', 3,
 ( #1939, #12823, #12470, #34515, #4423, #20471 ),
 .UNSPECIFIED., .F., .F.,
 ( 4, 2, 4 ),
 ( 2.257612537762607475E-07, 0.001873424083712463013, 0.003746622406171149465 ),
 .UNSPECIFIED. ) ;
#32230=AXIS2_PLACEMENT_3D ( 'NONE', #30601, #6192, #17087 ) ;
#32232=VERTEX_POINT ( 'NONE', #26748 ) ;
#32243=ORIENTED_EDGE ( 'NONE', *, *, #1100, .T. ) ;
#32247=CARTESIAN_POINT ( 'NONE',  ( 0.7561992106246575585, 31.72496621377049308, 11.99023130257964986 ) ) ;
#32249=CARTESIAN_POINT ( 'NONE',  ( 2.789999999999999591, 23.76428138080743224, 19.37504760381664326 ) ) ;
#32257=CARTESIAN_POINT ( 'NONE',  ( 50.00050000000000239, 12.80000000000000071, 3.000000000000000000 ) ) ;
#32258=CARTESIAN_POINT ( 'NONE',  ( 0.5248941666463887712, -24.85743842207099874, -22.27820639183348916 ) ) ;
#32261=FACE_OUTER_BOUND ( 'NONE', #34563, .T. ) ;
#32264=ORIENTED_EDGE ( 'NONE', *, *, #3010, .T. ) ;
#32268=AXIS2_PLACEMENT_3D ( 'NONE', #18047, #10006, #13043 ) ;
#32274=VERTEX_POINT ( 'NONE', #20888 ) ;
#32276=ORIENTED_EDGE ( 'NONE', *, *, #16095, .T. ) ;
#32281=EDGE_LOOP ( 'NONE', ( #32293, #34433, #21868, #29656, #25181, #31831 ) ) ;
#32290=EDGE_CURVE ( 'NONE', #693, #29128, #7611, .T. ) ;
#32292=DIRECTION ( 'NONE',  ( -1.000000000000000000, -0.000000000000000000, 0.000000000000000000 ) ) ;
#32293=ORIENTED_EDGE ( 'NONE', *, *, #17058, .F. ) ;
#32309=ORIENTED_EDGE ( 'NONE', *, *, #31304, .T. ) ;
#32310=CARTESIAN_POINT ( 'NONE',  ( 2.789999999999999147, -20.92506858792771851, 22.14933852381669510 ) ) ;
#32311=CARTESIAN_POINT ( 'NONE',  ( 2.604019738671253137, 26.80718912072147120, 17.98567582844242807 ) ) ;
#32315=ORIENTED_EDGE ( 'NONE', *, *, #25953, .F. ) ;
#32327=DIRECTION ( 'NONE',  ( -1.000000000000000000, -0.000000000000000000, -0.000000000000000000 ) ) ;
#32328=DIRECTION ( 'NONE',  ( 0.000000000000000000, 0.000000000000000000, 1.000000000000000000 ) ) ;
#32330=CARTESIAN_POINT ( 'NONE',  ( 2.790000000000000924, 9.539392014169456147, 3.000000000000000000 ) ) ;
#32332=CARTESIAN_POINT ( 'NONE',  ( -5.210000000000000853, 0.000000000000000000, 0.000000000000000000 ) ) ;
#32333=CARTESIAN_POINT ( 'NONE',  ( 2.604019717250312560, 4.859980099383894192, -31.91379830674618390 ) ) ;
#32336=VERTEX_POINT ( 'NONE', #2359 ) ;
#32338=LINE ( 'NONE', #10466, #364 ) ;
#32339=EDGE_CURVE ( 'NONE', #18246, #14020, #6932, .T. ) ;
#32364=CARTESIAN_POINT ( 'NONE',  ( -8.271081742788348749E-14, -25.79732705422383177, -16.24908268024335101 ) ) ;
#32368=CARTESIAN_POINT ( 'NONE',  ( 2.789999999999999147, 0.000000000000000000, 0.000000000000000000 ) ) ;
#32374=ORIENTED_EDGE ( 'NONE', *, *, #30869, .T. ) ;
#32376=EDGE_CURVE ( 'NONE', #31497, #16394, #15384, .T. ) ;
#32388=DIRECTION ( 'NONE',  ( -1.000000000000000000, -0.000000000000000000, 0.000000000000000000 ) ) ;
#32393=CARTESIAN_POINT ( 'NONE',  ( 2.765921099433441555, 4.286445725888036407, 30.79383171238946204 ) ) ;
#32396=DIRECTION ( 'NONE',  ( -1.000000000000000000, 0.000000000000000000, 0.000000000000000000 ) ) ;
#32403=EDGE_CURVE ( 'NONE', #12523, #34039, #4713, .T. ) ;
#32406=ORIENTED_EDGE ( 'NONE', *, *, #1011, .T. ) ;
#32409=ADVANCED_FACE ( 'NONE', ( #5381 ), #24098, .T. ) ;
#32416=DIRECTION ( 'NONE',  ( -1.000000000000000000, -0.000000000000000000, -0.000000000000000000 ) ) ;
#32425=CIRCLE ( 'NONE', #27968, 34.41491905851385269 ) ;
#32426=CARTESIAN_POINT ( 'NONE',  ( 0.02407890056655825201, -23.70329957282570632, -20.11932597908854703 ) ) ;
#32428=AXIS2_PLACEMENT_3D ( 'NONE', #15810, #10449, #1564 ) ;
#32440=EDGE_CURVE ( 'NONE', #8699, #29138, #14531, .T. ) ;
#32441=EDGE_CURVE ( 'NONE', #23190, #21389, #6474, .T. ) ;
#32447=LINE ( 'NONE', #15574, #13926 ) ;
#32465=VECTOR ( 'NONE', #30654, 1000.000000000000000 ) ;
#32472=VERTEX_POINT ( 'NONE', #13761 ) ;
#32475=DIRECTION ( 'NONE',  ( -1.000000000000000000, -0.000000000000000000, 0.000000000000000000 ) ) ;
#32482=ADVANCED_FACE ( 'NONE', ( #16802 ), #26365, .T. ) ;
#32487=DIRECTION ( 'NONE',  ( 0.000000000000000000, 0.000000000000000000, 1.000000000000000000 ) ) ;
#32497=VERTEX_POINT ( 'NONE', #29954 ) ;
#32502=CIRCLE ( 'NONE', #29671, 2.525000000000001243 ) ;
#32510=CARTESIAN_POINT ( 'NONE',  ( 2.765921099433441999, -0.3931553186915530129, 31.08824725498900321 ) ) ;
#32515=EDGE_LOOP ( 'NONE', ( #22086, #26925, #33039, #31160, #26474, #24888 ) ) ;
#32517=CARTESIAN_POINT ( 'NONE',  ( 2.765921099433443331, 18.59128259035506758, -24.91982945642901726 ) ) ;
#32524=ORIENTED_EDGE ( 'NONE', *, *, #19016, .T. ) ;
#32528=B_SPLINE_CURVE_WITH_KNOTS ( 'NONE', 3,
 ( #23844, #29007, #21179, #1956, #12834, #23674 ),
 .UNSPECIFIED., .F., .F.,
 ( 4, 2, 4 ),
 ( 2.178692866010994808E-07, 0.001873416183138254271, 0.003746614496989907669 ),
 .UNSPECIFIED. ) ;
#32538=VECTOR ( 'NONE', #5548, 1000.000000000000000 ) ;
#32541=VERTEX_POINT ( 'NONE', #8757 ) ;
#32546=ORIENTED_EDGE ( 'NONE', *, *, #15449, .F. ) ;
#32548=CARTESIAN_POINT ( 'NONE',  ( 2.719010745927727513, -28.42160548755730787, 14.02701190433877265 ) ) ;
#32551=CARTESIAN_POINT ( 'NONE',  ( 2.789999999999999147, 0.000000000000000000, 0.000000000000000000 ) ) ;
#32554=DIRECTION ( 'NONE',  ( -1.000000000000000000, -0.000000000000000000, -0.000000000000000000 ) ) ;
#32557=CARTESIAN_POINT ( 'NONE',  ( 1.040000000000001590, 32.09669216789235691, 12.41728656686385968 ) ) ;
#32559=DIRECTION ( 'NONE',  ( -1.000000000000000000, -0.000000000000000000, -0.000000000000000000 ) ) ;
#32562=CIRCLE ( 'NONE', #12694, 30.47050528711512030 ) ;
#32565=FACE_OUTER_BOUND ( 'NONE', #27320, .T. ) ;
#32567=DIRECTION ( 'NONE',  ( 0.000000000000000000, 0.000000000000000000, 1.000000000000000000 ) ) ;
#32581=CARTESIAN_POINT ( 'NONE',  ( 2.783107618245967085, 20.89684813776040428, -22.72149230800609487 ) ) ;
#32585=AXIS2_PLACEMENT_3D ( 'NONE', #11668, #22699, #6119 ) ;
#32598=CARTESIAN_POINT ( 'NONE',  ( -10.00000000000000000, 0.000000000000000000, 0.000000000000000000 ) ) ;
#32600=B_SPLINE_CURVE_WITH_KNOTS ( 'NONE', 3,
 ( #23879, #26904, #2518, #34748 ),
 .UNSPECIFIED., .F., .F.,
 ( 4, 4 ),
 ( 1.980634265047890748E-07, 0.0006879337600918691668 ),
 .UNSPECIFIED. ) ;
#32603=CARTESIAN_POINT ( 'NONE',  ( 0.006871088337153627955, -23.57967537501776789, 19.92301408446852307 ) ) ;
#32605=EDGE_CURVE ( 'NONE', #3111, #23519, #21757, .T. ) ;
#32609=VERTEX_POINT ( 'NONE', #25653 ) ;
#32612=CARTESIAN_POINT ( 'NONE',  ( 1.749999999999999778, -34.41385771548412720, -0.2702793785573802121 ) ) ;
#32617=EDGE_CURVE ( 'NONE', #28456, #7179, #17116, .T. ) ;
#32621=VERTEX_POINT ( 'NONE', #28509 ) ;
#32624=B_SPLINE_CURVE_WITH_KNOTS ( 'NONE', 3,
 ( #10928, #16460, #32969, #16818 ),
 .UNSPECIFIED., .F., .F.,
 ( 4, 4 ),
 ( 2.180635439307184488E-07, 0.0006879539277919237373 ),
 .UNSPECIFIED. ) ;
#32629=VERTEX_POINT ( 'NONE', #12497 ) ;
#32632=CIRCLE ( 'NONE', #16176, 30.47050528711512030 ) ;
#32634=DIRECTION ( 'NONE',  ( 0.000000000000000000, 0.000000000000000000, 1.000000000000000000 ) ) ;
#32635=VERTEX_POINT ( 'NONE', #9986 ) ;
#32640=CYLINDRICAL_SURFACE ( 'NONE', #16455, 2.524999999999999467 ) ;
#32641=VERTEX_POINT ( 'NONE', #7473 ) ;
#32644=CARTESIAN_POINT ( 'NONE',  ( 0.02407890056655781832, 4.286445725888479608, -30.79383171238939809 ) ) ;
#32648=ORIENTED_EDGE ( 'NONE', *, *, #12233, .F. ) ;
#32657=EDGE_CURVE ( 'NONE', #8838, #25584, #31855, .T. ) ;
#32672=VERTEX_POINT ( 'NONE', #34545 ) ;
#32675=CARTESIAN_POINT ( 'NONE',  ( 2.789999999999999591, 30.58654839005191306, -2.143968220813880166 ) ) ;
#32676=DIRECTION ( 'NONE',  ( -1.000000000000000000, -0.000000000000000000, -0.000000000000000000 ) ) ;
#32682=CARTESIAN_POINT ( 'NONE',  ( 2.789999999999999147, -16.83127206196721914, -25.36297913013192584 ) ) ;
#32683=CARTESIAN_POINT ( 'NONE',  ( 2.765921099433441999, 7.350529080603541487, 30.20932655202940254 ) ) ;
#32685=CYLINDRICAL_SURFACE ( 'NONE', #16230, 34.41491905851385269 ) ;
#32689=VECTOR ( 'NONE', #11520, 1000.000000000000000 ) ;
#32696=ORIENTED_EDGE ( 'NONE', *, *, #26275, .F. ) ;
#32698=AXIS2_PLACEMENT_3D ( 'NONE', #30211, #5815, #27543 ) ;
#32716=CARTESIAN_POINT ( 'NONE',  ( 0.07098931521633271291, 24.79335165344852854, -19.74422662903591785 ) ) ;
#32723=DIRECTION ( 'NONE',  ( 0.000000000000000000, 0.9980267284282708928, 0.06279051952932451774 ) ) ;
#32725=CARTESIAN_POINT ( 'NONE',  ( 1.749999999999999778, -30.28730148581149706, -16.34215476954067015 ) ) ;
#32727=CARTESIAN_POINT ( 'NONE',  ( 2.789999999999999147, 27.98916443103598439, 15.38717335695048227 ) ) ;
#32730=CARTESIAN_POINT ( 'NONE',  ( 2.790000000000082192, -17.84469521343956444, -24.93532764985541661 ) ) ;
#32733=CYLINDRICAL_SURFACE ( 'NONE', #20945, 2.524999999999999467 ) ;
#32740=CARTESIAN_POINT ( 'NONE',  ( 1.394999999999999574, 28.00026196654270905, 20.00929742917132970 ) ) ;
#32744=DIRECTION ( 'NONE',  ( 0.000000000000000000, -0.6845471059286900584, 0.7289686274214099981 ) ) ;
#32745=CARTESIAN_POINT ( 'NONE',  ( 2.789999999999999147, -26.96806452364392470, 14.11722088188904145 ) ) ;
#32759=VERTEX_POINT ( 'NONE', #15168 ) ;
#32760=DIRECTION ( 'NONE',  ( -1.000000000000000000, -0.000000000000000000, -0.000000000000000000 ) ) ;
#32779=EDGE_CURVE ( 'NONE', #2667, #6345, #17712, .T. ) ;
#32780=CARTESIAN_POINT ( 'NONE',  ( 0.7561992263366478229, -10.98362253094209606, -32.08736770015226369 ) ) ;
#32783=CARTESIAN_POINT ( 'NONE',  ( 2.789999999999999147, 23.28319895603611300, -21.86437915510192909 ) ) ;
#32785=AXIS2_PLACEMENT_3D ( 'NONE', #18873, #19056, #19398 ) ;
#32787=EDGE_CURVE ( 'NONE', #16809, #27823, #29394, .T. ) ;
#32795=DIRECTION ( 'NONE',  ( 1.000000000000000000, 0.000000000000000000, 0.000000000000000000 ) ) ;
#32799=CARTESIAN_POINT ( 'NONE',  ( 1.040000000000000924, 0.000000000000000000, 0.000000000000000000 ) ) ;
#32808=EDGE_LOOP ( 'NONE', ( #24519, #25249, #31192, #2966, #18015, #19062, #2649 ) ) ;
#32814=CIRCLE ( 'NONE', #18641, 30.47050528711511674 ) ;
#32819=DIRECTION ( 'NONE',  ( -0.000000000000000000, 0.000000000000000000, 1.000000000000000000 ) ) ;
#32820=CARTESIAN_POINT ( 'NONE',  ( 2.033800773547048024, -32.71371797491563882, -8.947166372575045656 ) ) ;
#32831=CIRCLE ( 'NONE', #4982, 30.47050528711512030 ) ;
#32842=ORIENTED_EDGE ( 'NONE', *, *, #15287, .F. ) ;
#32849=CARTESIAN_POINT ( 'NONE',  ( 2.719010697917859876, -22.12324074713392719, -22.69596835361152998 ) ) ;
#32859=DIRECTION ( 'NONE',  ( 0.000000000000000000, 0.000000000000000000, 1.000000000000000000 ) ) ;
#32866=CARTESIAN_POINT ( 'NONE',  ( 2.783128676084626552, 4.186936631163378664, -30.58426604563490159 ) ) ;
#32877=ORIENTED_EDGE ( 'NONE', *, *, #20176, .T. ) ;
#32886=ORIENTED_EDGE ( 'NONE', *, *, #10871, .F. ) ;
#32890=EDGE_CURVE ( 'NONE', #24367, #14830, #19607, .T. ) ;
#32896=ORIENTED_EDGE ( 'NONE', *, *, #4562, .T. ) ;
#32900=CARTESIAN_POINT ( 'NONE',  ( 2.604019720910715652, -22.69026646801078329, 22.96218055026789528 ) ) ;
#32908=ORIENTED_EDGE ( 'NONE', *, *, #15863, .F. ) ;
#32912=LINE ( 'NONE', #32740, #6951 ) ;
#32914=CARTESIAN_POINT ( 'NONE',  ( 0.000000000000000000, 0.000000000000000000, 0.000000000000000000 ) ) ;
#32919=CARTESIAN_POINT ( 'NONE',  ( 2.719051660475461762, -3.385765165811317701, -31.51266256086719153 ) ) ;
#32931=ADVANCED_FACE ( 'NONE', ( #32261 ), #16086, .F. ) ;
#32934=ORIENTED_EDGE ( 'NONE', *, *, #14083, .T. ) ;
#32938=DIRECTION ( 'NONE',  ( 0.000000000000000000, 0.000000000000000000, 1.000000000000000000 ) ) ;
#32949=VERTEX_POINT ( 'NONE', #27096 ) ;
#32950=CARTESIAN_POINT ( 'NONE',  ( 2.265105771424310355, 33.20489141755878393, -3.412611943275337900 ) ) ;
#32957=CARTESIAN_POINT ( 'NONE',  ( 0.02407890056655695096, 30.61125888652969707, -5.439165181698684570 ) ) ;
#32959=AXIS2_PLACEMENT_3D ( 'NONE', #34346, #2163, #24220 ) ;
#32968=EDGE_CURVE ( 'NONE', #34030, #2667, #21327, .T. ) ;
#32969=CARTESIAN_POINT ( 'NONE',  ( 2.790000000000081748, 20.82920972943033888, 22.50217193233309487 ) ) ;
#32979=EDGE_CURVE ( 'NONE', #21650, #13146, #17947, .T. ) ;
#32997=CARTESIAN_POINT ( 'NONE',  ( 1.749999999999999778, 28.00026196654299326, -20.00929742917092469 ) ) ;
#32999=ORIENTED_EDGE ( 'NONE', *, *, #21975, .T. ) ;
#33000=FACE_OUTER_BOUND ( 'NONE', #5862, .T. ) ;
#33001=CARTESIAN_POINT ( 'NONE',  ( 0.000000000000000000, 23.28319895603611300, -19.33937915510192695 ) ) ;
#33003=ORIENTED_EDGE ( 'NONE', *, *, #28406, .F. ) ;
#33010=VERTEX_POINT ( 'NONE', #7880 ) ;
#33014=CARTESIAN_POINT ( 'NONE',  ( 0.000000000000000000, -17.83604598421647935, -24.70480026434186982 ) ) ;
#33017=EDGE_CURVE ( 'NONE', #29292, #28354, #8225, .T. ) ;
#33019=EDGE_CURVE ( 'NONE', #33515, #32629, #24125, .T. ) ;
#33020=ORIENTED_EDGE ( 'NONE', *, *, #30836, .T. ) ;
#33021=CIRCLE ( 'NONE', #2330, 34.41491905851385269 ) ;
#33022=CARTESIAN_POINT ( 'NONE',  ( 0.02407890056655651728, 29.44518845714764765, 9.980709654879525772 ) ) ;
#33023=LINE ( 'NONE', #27693, #11826 ) ;
#33028=CARTESIAN_POINT ( 'NONE',  ( 0.07094833961210175732, 14.74858964725109267, -28.05334937082576374 ) ) ;
#33032=ORIENTED_EDGE ( 'NONE', *, *, #22851, .T. ) ;
#33039=ORIENTED_EDGE ( 'NONE', *, *, #9384, .F. ) ;
#33044=EDGE_CURVE ( 'NONE', #23276, #16809, #7078, .T. ) ;
#33050=CARTESIAN_POINT ( 'NONE',  ( 0.006892399591254335864, -7.987299431473847910, 29.81857704081742355 ) ) ;
#33053=CARTESIAN_POINT ( 'NONE',  ( -10.00000000000000000, 0.000000000000000000, 0.000000000000000000 ) ) ;
#33057=CARTESIAN_POINT ( 'NONE',  ( 2.790000000000079972, -30.07763130521186312, -5.961539033704989166 ) ) ;
#33061=CARTESIAN_POINT ( 'NONE',  ( 2.765921099433441999, -31.05158812718222450, 1.559667679918499417 ) ) ;
#33069=VERTEX_POINT ( 'NONE', #8410 ) ;
#33074=CARTESIAN_POINT ( 'NONE',  ( 2.719051683612535797, -28.42120447776860104, -14.02663268823320486 ) ) ;
#33078=ORIENTED_EDGE ( 'NONE', *, *, #29931, .T. ) ;
#33079=ORIENTED_EDGE ( 'NONE', *, *, #26237, .F. ) ;
#33100=ADVANCED_FACE ( 'NONE', ( #408 ), #3582, .F. ) ;
#33101=AXIS2_PLACEMENT_3D ( 'NONE', #2026, #18242, #1846 ) ;
#33102=ORIENTED_EDGE ( 'NONE', *, *, #23664, .T. ) ;
#33121=DIRECTION ( 'NONE',  ( -1.000000000000000000, 0.000000000000000000, -0.000000000000000000 ) ) ;
#33134=EDGE_CURVE ( 'NONE', #13146, #34260, #16208, .T. ) ;
#33146=B_SPLINE_CURVE_WITH_KNOTS ( 'NONE', 3,
 ( #33351, #22687, #14685, #9320 ),
 .UNSPECIFIED., .F., .F.,
 ( 4, 4 ),
 ( 3.346525879968219986E-07, 0.0006880714927763689238 ),
 .UNSPECIFIED. ) ;
#33159=ORIENTED_EDGE ( 'NONE', *, *, #1253, .F. ) ;
#33162=ORIENTED_EDGE ( 'NONE', *, *, #28945, .F. ) ;
#33169=ORIENTED_EDGE ( 'NONE', *, *, #19114, .F. ) ;
#33172=CARTESIAN_POINT ( 'NONE',  ( 0.07098932641069075067, -3.385659728283963332, -31.51320498992189911 ) ) ;
#33193=EDGE_CURVE ( 'NONE', #34596, #7115, #12383, .T. ) ;
#33200=ORIENTED_EDGE ( 'NONE', *, *, #21992, .F. ) ;
#33204=DIRECTION ( 'NONE',  ( -1.000000000000000000, 0.000000000000000000, -0.000000000000000000 ) ) ;
#33205=AXIS2_PLACEMENT_3D ( 'NONE', #18235, #9852, #1839 ) ;
#33218=LINE ( 'NONE', #833, #11315 ) ;
#33223=CARTESIAN_POINT ( 'NONE',  ( 2.789999999999999147, -0.09145294252698496495, 30.47036804522407749 ) ) ;
#33225=AXIS2_PLACEMENT_3D ( 'NONE', #12340, #4297, #33866 ) ;
#33228=EDGE_CURVE ( 'NONE', #5130, #23546, #12324, .T. ) ;
#33233=LINE ( 'NONE', #8030, #18128 ) ;
#33234=AXIS2_PLACEMENT_3D ( 'NONE', #20716, #15382, #25520 ) ;
#33245=DIRECTION ( 'NONE',  ( 0.000000000000000000, 0.000000000000000000, 1.000000000000000000 ) ) ;
#33247=CARTESIAN_POINT ( 'NONE',  ( 0.000000000000000000, -25.83993731729781729, -18.77381338200996552 ) ) ;
#33253=VERTEX_POINT ( 'NONE', #20672 ) ;
#33260=CARTESIAN_POINT ( 'NONE',  ( 2.783107609940381533, 11.66157578832064345, 28.58237449055242152 ) ) ;
#33273=CARTESIAN_POINT ( 'NONE',  ( 0.000000000000000000, 29.94779062842788164, 5.619744560739158068 ) ) ;
#33277=CIRCLE ( 'NONE', #24784, 2.525000000000000799 ) ;
#33281=CARTESIAN_POINT ( 'NONE',  ( 0.7561992229685223776, -1.599833918847833880, 33.87742110695030107 ) ) ;
#33292=EDGE_CURVE ( 'NONE', #34395, #6886, #5984, .T. ) ;
#33301=EDGE_CURVE ( 'NONE', #32672, #6398, #22136, .T. ) ;
#33304=DIRECTION ( 'NONE',  ( -1.000000000000000000, 0.000000000000000000, 0.000000000000000000 ) ) ;
#33312=DIRECTION ( 'NONE',  ( -1.000000000000000000, -0.000000000000000000, -0.000000000000000000 ) ) ;
#33341=ORIENTED_EDGE ( 'NONE', *, *, #17193, .T. ) ;
#33342=DIRECTION ( 'NONE',  ( 0.000000000000000000, 0.000000000000000000, 1.000000000000000000 ) ) ;
#33348=VECTOR ( 'NONE', #31846, 1000.000000000000000 ) ;
#33349=CARTESIAN_POINT ( 'NONE',  ( -7.057945688734196724E-17, 18.19930456030807164, -24.67628137665877830 ) ) ;
#33351=CARTESIAN_POINT ( 'NONE',  ( 2.765921099433444663, 29.44518845714764765, 9.980709654879525772 ) ) ;
#33352=ORIENTED_EDGE ( 'NONE', *, *, #13428, .T. ) ;
#33355=CARTESIAN_POINT ( 'NONE',  ( 0.000000000000000000, -23.41952779159775488, 19.49300927180538778 ) ) ;
#33367=B_SPLINE_CURVE_WITH_KNOTS ( 'NONE', 3,
 ( #7034, #20738, #8090, #267 ),
 .UNSPECIFIED., .F., .F.,
 ( 4, 4 ),
 ( 3.668583969211562668E-07, 0.0006881039678813115779 ),
 .UNSPECIFIED. ) ;
#33378=VERTEX_POINT ( 'NONE', #27355 ) ;
#33382=CARTESIAN_POINT ( 'NONE',  ( 0.000000000000000000, 28.95078156989571738, -9.502838467757779739 ) ) ;
#33388=CARTESIAN_POINT ( 'NONE',  ( 0.02407890056655564992, -30.46391896562411716, 6.211548095912460710 ) ) ;
#33390=EDGE_CURVE ( 'NONE', #7267, #2456, #34375, .T. ) ;
#33396=CARTESIAN_POINT ( 'NONE',  ( 2.397606348813468014, 30.27116788627787614, 13.00174666746673324 ) ) ;
#33408=TOROIDAL_SURFACE ( 'NONE', #19779, 30.47050528711511674, 8.000000000000000000 ) ;
#33417=ORIENTED_EDGE ( 'NONE', *, *, #23868, .T. ) ;
#33421=CIRCLE ( 'NONE', #14625, 2.524999999999999467 ) ;
#33423=DIRECTION ( 'NONE',  ( -1.000000000000000000, -0.000000000000000000, -0.000000000000000000 ) ) ;
#33424=DIRECTION ( 'NONE',  ( -1.000000000000000000, 0.000000000000000000, 0.000000000000000000 ) ) ;
#33432=CARTESIAN_POINT ( 'NONE',  ( 2.783128911662848370, -23.57967537501747302, -19.92301408446885347 ) ) ;
#33439=ORIENTED_EDGE ( 'NONE', *, *, #13471, .F. ) ;
#33440=CARTESIAN_POINT ( 'NONE',  ( 2.765921099433443331, 26.03801215795517621, 16.98986790278620873 ) ) ;
#33443=AXIS2_PLACEMENT_3D ( 'NONE', #18538, #9798, #10325 ) ;
#33445=ORIENTED_EDGE ( 'NONE', *, *, #34382, .T. ) ;
#33457=ORIENTED_EDGE ( 'NONE', *, *, #2567, .T. ) ;
#33461=EDGE_LOOP ( 'NONE', ( #23431, #6394, #21867, #34779 ) ) ;
#33463=CARTESIAN_POINT ( 'NONE',  ( 2.789999999999999147, -29.68817180695682723, 9.232883799364120847 ) ) ;
#33465=CYLINDRICAL_SURFACE ( 'NONE', #28986, 34.41491905851385269 ) ;
#33471=B_SPLINE_CURVE_WITH_KNOTS ( 'NONE', 3,
 ( #19032, #29874, #30923, #3856 ),
 .UNSPECIFIED., .F., .F.,
 ( 4, 4 ),
 ( 2.038594426221743809E-07, 0.0006879396046783100693 ),
 .UNSPECIFIED. ) ;
#33473=DIRECTION ( 'NONE',  ( 0.000000000000000000, 0.000000000000000000, 1.000000000000000000 ) ) ;
#33474=ORIENTED_EDGE ( 'NONE', *, *, #17723, .T. ) ;
#33476=ADVANCED_FACE ( 'NONE', ( #4614 ), #23578, .T. ) ;
#33479=FACE_OUTER_BOUND ( 'NONE', #12337, .T. ) ;
#33485=DIRECTION ( 'NONE',  ( -1.000000000000000000, 0.000000000000000000, 0.000000000000000000 ) ) ;
#33495=CARTESIAN_POINT ( 'NONE',  ( 2.789999999999999147, 30.93646776788796160, 7.943134866716423659 ) ) ;
#33504=ORIENTED_EDGE ( 'NONE', *, *, #25868, .F. ) ;
#33508=ORIENTED_EDGE ( 'NONE', *, *, #19889, .T. ) ;
#33511=VERTEX_POINT ( 'NONE', #28425 ) ;
#33515=VERTEX_POINT ( 'NONE', #22202 ) ;
#33519=CARTESIAN_POINT ( 'NONE',  ( 0.000000000000000000, -31.68806325674609781, 4.003133335385473224 ) ) ;
#33520=B_SPLINE_CURVE_WITH_KNOTS ( 'NONE', 3,
 ( #25538, #9534, #31240, #23236, #28575, #33911 ),
 .UNSPECIFIED., .F., .F.,
 ( 4, 2, 4 ),
 ( 4.404817032094653926E-07, 0.001874269626248360049, 0.003748098770793510670 ),
 .UNSPECIFIED. ) ;
#33524=ORIENTED_EDGE ( 'NONE', *, *, #2196, .F. ) ;
#33532=AXIS2_PLACEMENT_3D ( 'NONE', #908, #9087, #19953 ) ;
#33537=CARTESIAN_POINT ( 'NONE',  ( 2.789999999999999147, 6.312585643774966115, -29.77790610619679512 ) ) ;
#33544=CARTESIAN_POINT ( 'NONE',  ( 2.765921099433443775, -31.05158812718220673, -1.559667679918931738 ) ) ;
#33551=ORIENTED_EDGE ( 'NONE', *, *, #1408, .T. ) ;
#33557=ORIENTED_EDGE ( 'NONE', *, *, #10687, .T. ) ;
#33566=CARTESIAN_POINT ( 'NONE',  ( 2.789999999999999147, 28.06759692514767934, 11.78059558880223712 ) ) ;
#33576=( NAMED_UNIT ( * ) PLANE_ANGLE_UNIT ( ) SI_UNIT ( $, .RADIAN. ) );
#33578=EDGE_CURVE ( 'NONE', #33515, #16809, #12249, .T. ) ;
#33582=VERTEX_POINT ( 'NONE', #31099 ) ;
#33586=MANIFOLD_SOLID_BREP ( 'Keyway', #26452 ) ;
#33587=ORIENTED_EDGE ( 'NONE', *, *, #23864, .T. ) ;
#33599=ORIENTED_EDGE ( 'NONE', *, *, #3950, .T. ) ;
#33607=CARTESIAN_POINT ( 'NONE',  ( 2.789999999999999147, 11.30192140231231868, 28.29696565125074414 ) ) ;
#33633=EDGE_LOOP ( 'NONE', ( #1002, #20836, #7350, #4859 ) ) ;
#33637=ADVANCED_FACE ( 'NONE', ( #20419 ), #4577, .T. ) ;
#33639=CARTESIAN_POINT ( 'NONE',  ( -10.00000000000000000, 0.000000000000000000, 0.000000000000000000 ) ) ;
#33640=DIRECTION ( 'NONE',  ( -1.000000000000000000, -0.000000000000000000, -0.000000000000000000 ) ) ;
#33644=AXIS2_PLACEMENT_3D ( 'NONE', #5503, #21890, #16401 ) ;
#33654=DIRECTION ( 'NONE',  ( -1.000000000000000000, -0.000000000000000000, -0.000000000000000000 ) ) ;
#33655=DIRECTION ( 'NONE',  ( 0.000000000000000000, 1.374038396813311798E-15, -1.000000000000000000 ) ) ;
#33657=CARTESIAN_POINT ( 'NONE',  ( 0.1859802790892826907, -22.69026646801045999, -22.96218055026821858 ) ) ;
#33658=CARTESIAN_POINT ( 'NONE',  ( 1.749999999999999778, -10.89151784028311809, 32.64600270996213283 ) ) ;
#33668=AXIS2_PLACEMENT_3D ( 'NONE', #30708, #8993, #22526 ) ;
#33673=EDGE_CURVE ( 'NONE', #7946, #6878, #34639, .T. ) ;
#33679=VERTEX_POINT ( 'NONE', #21105 ) ;
#33683=B_SPLINE_CURVE_WITH_KNOTS ( 'NONE', 3,
 ( #28189, #3791, #28878, #16073 ),
 .UNSPECIFIED., .F., .F.,
 ( 4, 4 ),
 ( 1.976296719774577317E-07, 0.0006879333227023364796 ),
 .UNSPECIFIED. ) ;
#33705=ORIENTED_EDGE ( 'NONE', *, *, #34025, .T. ) ;
#33710=CARTESIAN_POINT ( 'NONE',  ( 0.7561992196122224730, 22.02446183774635102, 25.79073883748091589 ) ) ;
#33713=VECTOR ( 'NONE', #13619, 1000.000000000000000 ) ;
#33717=CARTESIAN_POINT ( 'NONE',  ( 2.765921099433442443, 28.29688452313417812, -12.88099432405573630 ) ) ;
#33722=EDGE_CURVE ( 'NONE', #24969, #8699, #15792, .T. ) ;
#33725=CARTESIAN_POINT ( 'NONE',  ( 2.783128933130080362, 30.78681169157792041, 2.258271426746184751 ) ) ;
#33726=ORIENTED_EDGE ( 'NONE', *, *, #33758, .F. ) ;
#33734=VECTOR ( 'NONE', #14403, 1000.000000000000000 ) ;
#33745=EDGE_CURVE ( 'NONE', #5785, #939, #1341, .T. ) ;
#33750=AXIS2_PLACEMENT_3D ( 'NONE', #14650, #25650, #5895 ) ;
#33752=ORIENTED_EDGE ( 'NONE', *, *, #20387, .F. ) ;
#33753=CARTESIAN_POINT ( 'NONE',  ( 0.02407890056655651728, -15.32140196853772984, 27.05343472112986092 ) ) ;
#33758=EDGE_CURVE ( 'NONE', #5512, #6878, #34881, .T. ) ;
#33764=FACE_OUTER_BOUND ( 'NONE', #29397, .T. ) ;
#33768=DIRECTION ( 'NONE',  ( -1.000000000000000000, -0.000000000000000000, -0.000000000000000000 ) ) ;
#33782=CARTESIAN_POINT ( 'NONE',  ( 8.000000000000000000, 0.000000000000000000, 0.000000000000000000 ) ) ;
#33798=FACE_OUTER_BOUND ( 'NONE', #8330, .T. ) ;
#33812=ORIENTED_EDGE ( 'NONE', *, *, #10904, .T. ) ;
#33814=B_SPLINE_CURVE_WITH_KNOTS ( 'NONE', 3,
 ( #16698, #14018, #27010, #8490, #2963, #131 ),
 .UNSPECIFIED., .F., .F.,
 ( 4, 2, 4 ),
 ( 2.699892344249078029E-07, 0.001873468359919019379, 0.003746666730603614125 ),
 .UNSPECIFIED. ) ;
#33818=AXIS2_PLACEMENT_3D ( 'NONE', #26823, #26469, #2786 ) ;
#33828=EDGE_CURVE ( 'NONE', #34039, #8710, #1710, .T. ) ;
#33830=CARTESIAN_POINT ( 'NONE',  ( 1.749999999999999778, 14.89726405156217126, 31.02351007835983054 ) ) ;
#33832=EDGE_LOOP ( 'NONE', ( #4007, #27857, #27402, #4545 ) ) ;
#33844=B_SPLINE_CURVE_WITH_KNOTS ( 'NONE', 3,
 ( #6036, #8896, #30966, #19770, #30617, #17105 ),
 .UNSPECIFIED., .F., .F.,
 ( 4, 2, 4 ),
 ( 2.446897702433135647E-07, 0.001873443032870421906, 0.003746641375970600780 ),
 .UNSPECIFIED. ) ;
#33856=CARTESIAN_POINT ( 'NONE',  ( 2.789999999999999147, -20.35927063852824048, 24.61013060777164796 ) ) ;
#33862=FACE_OUTER_BOUND ( 'NONE', #16792, .T. ) ;
#33866=DIRECTION ( 'NONE',  ( 0.000000000000000000, 0.000000000000000000, 1.000000000000000000 ) ) ;
#33872=CARTESIAN_POINT ( 'NONE',  ( 0.5288002543229157748, 26.55216317045622532, 20.24504431679649485 ) ) ;
#33874=VERTEX_POINT ( 'NONE', #33717 ) ;
#33887=ADVANCED_FACE ( 'NONE', ( #30529 ), #16661, .T. ) ;
#33890=CARTESIAN_POINT ( 'NONE',  ( 1.749999999999999778, 28.00026196654299326, -20.00929742917092469 ) ) ;
#33892=CARTESIAN_POINT ( 'NONE',  ( 0.000000000000000000, -20.92506858792743785, -22.14933852381697932 ) ) ;
#33893=EDGE_CURVE ( 'NONE', #1226, #28359, #27668, .T. ) ;
#33894=CARTESIAN_POINT ( 'NONE',  ( 1.040000000000000702, 22.14447232807505728, 26.34405054495564968 ) ) ;
#33895=DIRECTION ( 'NONE',  ( -1.000000000000000000, 0.000000000000000000, 0.000000000000000000 ) ) ;
#33898=VERTEX_POINT ( 'NONE', #27495 ) ;
#33899=CARTESIAN_POINT ( 'NONE',  ( 0.02407890056655695096, 20.99477179376858871, -22.93149026599722617 ) ) ;
#33902=AXIS2_PLACEMENT_3D ( 'NONE', #22643, #9103, #20149 ) ;
#33904=DIRECTION ( 'NONE',  ( -1.000000000000000000, -0.000000000000000000, -0.000000000000000000 ) ) ;
#33911=CARTESIAN_POINT ( 'NONE',  ( 0.02407890056655825201, -17.95514392185434360, 25.38201125280350468 ) ) ;
#33929=FACE_OUTER_BOUND ( 'NONE', #29833, .T. ) ;
#33934=VERTEX_POINT ( 'NONE', #11853 ) ;
#33936=VERTEX_POINT ( 'NONE', #22702 ) ;
#33944=CARTESIAN_POINT ( 'NONE',  ( 0.000000000000000000, -30.41598411195412055, 1.821977758773545952 ) ) ;
#33956=CARTESIAN_POINT ( 'NONE',  ( 0.5248942554772805247, -28.86920449294106916, 16.75648442687110773 ) ) ;
#33960=ORIENTED_EDGE ( 'NONE', *, *, #30783, .T. ) ;
#33961=CARTESIAN_POINT ( 'NONE',  ( 1.040000000000001146, 34.10861917999622506, -4.581348211831715034 ) ) ;
#33970=CARTESIAN_POINT ( 'NONE',  ( 2.789940898827340199, -25.81863125502495038, -16.24881338200996694 ) ) ;
#33973=ORIENTED_EDGE ( 'NONE', *, *, #1510, .F. ) ;
#33975=CARTESIAN_POINT ( 'NONE',  ( 0.000000000000000000, 0.000000000000000000, 0.000000000000000000 ) ) ;
#33977=CARTESIAN_POINT ( 'NONE',  ( 2.604019725809434860, -24.34160354263056547, -21.20368514569445750 ) ) ;
#33989=EDGE_LOOP ( 'NONE', ( #27618, #3807, #23286, #6020 ) ) ;
#33996=CARTESIAN_POINT ( 'NONE',  ( 2.789999999999999147, -13.59935610937951900, -26.37510281771846365 ) ) ;
#33999=CYLINDRICAL_SURFACE ( 'NONE', #30608, 2.525000000000001243 ) ;
#34002=ORIENTED_EDGE ( 'NONE', *, *, #4051, .F. ) ;
#34010=CIRCLE ( 'NONE', #10725, 34.41491905851385269 ) ;
#34021=CARTESIAN_POINT ( 'NONE',  ( 0.02407890056655695096, -8.112136323389137260, 30.01377904834206589 ) ) ;
#34023=ADVANCED_FACE ( 'NONE', ( #6655 ), #3978, .F. ) ;
#34025=EDGE_CURVE ( 'NONE', #31497, #6008, #28001, .T. ) ;
#34030=VERTEX_POINT ( 'NONE', #4497 ) ;
#34035=ORIENTED_EDGE ( 'NONE', *, *, #34470, .T. ) ;
#34039=VERTEX_POINT ( 'NONE', #1671 ) ;
#34043=VERTEX_POINT ( 'NONE', #20723 ) ;
#34048=CARTESIAN_POINT ( 'NONE',  ( 2.765921099433442443, 20.99477179376858871, -22.93149026599722617 ) ) ;
#34052=TOROIDAL_SURFACE ( 'NONE', #1628, 30.47050528711512030, 8.000000000000000000 ) ;
#34056=CARTESIAN_POINT ( 'NONE',  ( 0.02407890056655781832, -29.68817180695682723, 9.232883799364120847 ) ) ;
#34059=CARTESIAN_POINT ( 'NONE',  ( -5.210000000000000853, 0.000000000000000000, 0.000000000000000000 ) ) ;
#34065=ORIENTED_EDGE ( 'NONE', *, *, #29687, .T. ) ;
#34068=DIRECTION ( 'NONE',  ( -1.000000000000000000, -0.000000000000000000, -0.000000000000000000 ) ) ;
#34077=FACE_OUTER_BOUND ( 'NONE', #21007, .T. ) ;
#34082=ADVANCED_FACE ( 'NONE', ( #21424 ), #27447, .T. ) ;
#34090=DIRECTION ( 'NONE',  ( -1.000000000000000000, -0.000000000000000000, -0.000000000000000000 ) ) ;
#34091=CARTESIAN_POINT ( 'NONE',  ( 2.789999999999999147, 0.000000000000000000, 0.000000000000000000 ) ) ;
#34095=CARTESIAN_POINT ( 'NONE',  ( 0.5248942443853367168, -18.53613167721941579, -27.76008932203601276 ) ) ;
#34096=ORIENTED_EDGE ( 'NONE', *, *, #15863, .T. ) ;
#34097=CARTESIAN_POINT ( 'NONE',  ( 2.604019705202075041, -11.11575656128824185, -30.30758796111462772 ) ) ;
#34107=DIRECTION ( 'NONE',  ( 1.000000000000000000, 0.000000000000000000, -0.000000000000000000 ) ) ;
#34136=CARTESIAN_POINT ( 'NONE',  ( 1.749999999999999778, -34.41385771548413430, 0.2702793785568976537 ) ) ;
#34137=CIRCLE ( 'NONE', #32428, 30.47050528711512030 ) ;
#34142=CARTESIAN_POINT ( 'NONE',  ( 2.606461937191911105, -24.33633102984369856, 21.19365992153269573 ) ) ;
#34145=CARTESIAN_POINT ( 'NONE',  ( 0.07094831696795600440, -15.78353653323357619, -27.48438217453501409 ) ) ;
#34157=CIRCLE ( 'NONE', #12579, 30.47050528711511674 ) ;
#34159=EDGE_CURVE ( 'NONE', #26602, #25989, #2885, .T. ) ;
#34169=DIRECTION ( 'NONE',  ( 0.000000000000000000, 0.000000000000000000, 1.000000000000000000 ) ) ;
#34172=ORIENTED_EDGE ( 'NONE', *, *, #22543, .T. ) ;
#34174=AXIS2_PLACEMENT_3D ( 'NONE', #24206, #27586, #5859 ) ;
#34180=EDGE_CURVE ( 'NONE', #25584, #20352, #24583, .T. ) ;
#34183=B_SPLINE_CURVE_WITH_KNOTS ( 'NONE', 3,
 ( #9145, #20370, #31217, #20202 ),
 .UNSPECIFIED., .F., .F.,
 ( 4, 4 ),
 ( 0.005298366463358190892, 0.005985234859393911803 ),
 .UNSPECIFIED. ) ;
#34188=VECTOR ( 'NONE', #30230, 1000.000000000000000 ) ;
#34198=VECTOR ( 'NONE', #12852, 1000.000000000000000 ) ;
#34220=CYLINDRICAL_SURFACE ( 'NONE', #8998, 16.19999999999999929 ) ;
#34236=CARTESIAN_POINT ( 'NONE',  ( 2.789999999999999147, -5.984944020945660803, -31.37417528048448645 ) ) ;
#34260=VERTEX_POINT ( 'NONE', #22480 ) ;
#34261=ORIENTED_EDGE ( 'NONE', *, *, #17723, .F. ) ;
#34262=CARTESIAN_POINT ( 'NONE',  ( 50.00050000000000239, 9.539392014169456147, -3.000000000000000000 ) ) ;
#34263=CARTESIAN_POINT ( 'NONE',  ( -6.246745248748235768E-16, -30.07665394020986227, -5.960573492977661481 ) ) ;
#34265=EDGE_CURVE ( 'NONE', #14153, #33515, #15718, .T. ) ;
#34269=ORIENTED_EDGE ( 'NONE', *, *, #10878, .F. ) ;
#34270=CARTESIAN_POINT ( 'NONE',  ( 2.783128947185056656, 30.38119646769590787, -5.469045072944661356 ) ) ;
#34273=ORIENTED_EDGE ( 'NONE', *, *, #16898, .F. ) ;
#34276=CARTESIAN_POINT ( 'NONE',  ( 1.040000000000000924, 0.000000000000000000, 0.000000000000000000 ) ) ;
#34277=LINE ( 'NONE', #9893, #12673 ) ;
#34278=VERTEX_POINT ( 'NONE', #25485 ) ;
#34281=CIRCLE ( 'NONE', #23476, 2.525000000000003020 ) ;
#34282=DIRECTION ( 'NONE',  ( 0.000000000000000000, 0.000000000000000000, 1.000000000000000000 ) ) ;
#34296=CARTESIAN_POINT ( 'NONE',  ( 1.395000000000002238, -34.41385771548413430, 0.2702793785568976537 ) ) ;
#34300=CARTESIAN_POINT ( 'NONE',  ( 0.07094833575216234756, 31.58891575048174971, -2.579090161526253588 ) ) ;
#34305=ORIENTED_EDGE ( 'NONE', *, *, #10871, .T. ) ;
#34310=CARTESIAN_POINT ( 'NONE',  ( 2.033589658306851344, 5.833445725193281639, -33.41010632092317678 ) ) ;
#34311=CARTESIAN_POINT ( 'NONE',  ( 2.789999999999999147, 17.11426446101236820, -26.96776559937708129 ) ) ;
#34312=CARTESIAN_POINT ( 'NONE',  ( 2.789999999999999147, -25.79731400673761144, -16.24908301080859374 ) ) ;
#34318=ORIENTED_EDGE ( 'NONE', *, *, #28945, .T. ) ;
#34321=EDGE_CURVE ( 'NONE', #20282, #26849, #15276, .T. ) ;
#34328=AXIS2_PLACEMENT_3D ( 'NONE', #18932, #16088, #16621 ) ;
#34338=CARTESIAN_POINT ( 'NONE',  ( 2.789999999999999591, -29.22790002295970524, -9.266248432308945127 ) ) ;
#34346=CARTESIAN_POINT ( 'NONE',  ( 0.000000000000000000, -5.984944020945660803, -31.37417528048448645 ) ) ;
#34352=CIRCLE ( 'NONE', #263, 34.41491905851385269 ) ;
#34353=CARTESIAN_POINT ( 'NONE',  ( 1.040000000000000480, 6.183021911001836735, 33.85493898757064812 ) ) ;
#34355=CARTESIAN_POINT ( 'NONE',  ( 2.789999999999999147, -26.36977540155018218, 15.20550475489928388 ) ) ;
#34358=CARTESIAN_POINT ( 'NONE',  ( 0.02407890056655695096, -23.70329957282599764, 20.11932597908820242 ) ) ;
#34360=ADVANCED_FACE ( 'NONE', ( #17514 ), #28345, .F. ) ;
#34362=DIRECTION ( 'NONE',  ( 0.000000000000000000, 0.000000000000000000, 1.000000000000000000 ) ) ;
#34365=CARTESIAN_POINT ( 'NONE',  ( 0.02407890056655825201, -31.05158812718220673, -1.559667679918931738 ) ) ;
#34372=CIRCLE ( 'NONE', #33818, 30.47050528711512030 ) ;
#34375=CIRCLE ( 'NONE', #10532, 34.41491905851385269 ) ;
#34377=AXIS2_PLACEMENT_3D ( 'NONE', #11187, #4945, #13156 ) ;
#34378=ORIENTED_EDGE ( 'NONE', *, *, #7737, .F. ) ;
#34379=ADVANCED_FACE ( 'NONE', ( #34548 ), #24384, .T. ) ;
#34381=EDGE_CURVE ( 'NONE', #33934, #30641, #12317, .T. ) ;
#34382=EDGE_CURVE ( 'NONE', #26602, #6257, #18686, .T. ) ;
#34383=DIRECTION ( 'NONE',  ( -1.000000000000000000, -0.000000000000000000, -0.000000000000000000 ) ) ;
#34389=ADVANCED_FACE ( 'NONE', ( #15885 ), #17260, .T. ) ;
#34395=VERTEX_POINT ( 'NONE', #11 ) ;
#34401=CARTESIAN_POINT ( 'NONE',  ( 1.040000000000000036, 14.40815186467775533, 31.25366880301323746 ) ) ;
#34402=DIRECTION ( 'NONE',  ( -1.000000000000000000, 0.000000000000000000, -0.000000000000000000 ) ) ;
#34407=EDGE_CURVE ( 'NONE', #28097, #22681, #24029, .T. ) ;
#34410=EDGE_LOOP ( 'NONE', ( #20427, #24428, #2346, #3940, #13810, #10454 ) ) ;
#34411=TOROIDAL_SURFACE ( 'NONE', #9397, 30.47050528711511674, 8.000000000000000000 ) ;
#34429=ADVANCED_FACE ( 'NONE', ( #32042 ), #188, .T. ) ;
#34433=ORIENTED_EDGE ( 'NONE', *, *, #34470, .F. ) ;
#34443=CARTESIAN_POINT ( 'NONE',  ( 0.02407890056655651728, 11.80989368511502846, -28.76039115933972923 ) ) ;
#34456=ORIENTED_EDGE ( 'NONE', *, *, #22597, .F. ) ;
#34457=DIRECTION ( 'NONE',  ( 1.000000000000000000, -0.000000000000000000, 0.000000000000000000 ) ) ;
#34459=CYLINDRICAL_SURFACE ( 'NONE', #21960, 2.525000000000003020 ) ;
#34463=ORIENTED_EDGE ( 'NONE', *, *, #15727, .T. ) ;
#34470=EDGE_CURVE ( 'NONE', #5322, #26512, #28032, .T. ) ;
#34472=ORIENTED_EDGE ( 'NONE', *, *, #2592, .F. ) ;
#34480=CARTESIAN_POINT ( 'NONE',  ( 1.040000000000002922, 34.17636915695680244, -4.045051921974834208 ) ) ;
#34481=ORIENTED_EDGE ( 'NONE', *, *, #2968, .T. ) ;
#34482=VERTEX_POINT ( 'NONE', #16229 ) ;
#34485=AXIS2_PLACEMENT_3D ( 'NONE', #25887, #4154, #30530 ) ;
#34486=CARTESIAN_POINT ( 'NONE',  ( -8.242531583266565685E-14, -3.624739946994197215, 30.44774159452261486 ) ) ;
#34494=DIRECTION ( 'NONE',  ( -1.000000000000000000, 0.000000000000000000, 0.000000000000000000 ) ) ;
#34498=CIRCLE ( 'NONE', #28251, 30.47050528711512030 ) ;
#34505=CARTESIAN_POINT ( 'NONE',  ( 0.02407890056655651728, 7.350529080603541487, 30.20932655202940254 ) ) ;
#34508=EDGE_CURVE ( 'NONE', #30531, #9222, #10525, .T. ) ;
#34510=ORIENTED_EDGE ( 'NONE', *, *, #21700, .F. ) ;
#34515=CARTESIAN_POINT ( 'NONE',  ( 0.5248941893598875197, -32.51534716424833960, -7.547378828040798737 ) ) ;
#34519=CARTESIAN_POINT ( 'NONE',  ( 0.006892386851572370257, -27.79373726981368620, -13.43326644626254662 ) ) ;
#34522=CARTESIAN_POINT ( 'NONE',  ( 1.394999999999999574, -10.37741591188917134, 32.81304455236865181 ) ) ;
#34526=CARTESIAN_POINT ( 'NONE',  ( 1.749999999999999778, 27.68252950111338251, 20.44661865013498669 ) ) ;
#34530=CARTESIAN_POINT ( 'NONE',  ( 0.07094833381203961842, 4.557485336350485028, 31.36463980626633941 ) ) ;
#34531=ORIENTED_EDGE ( 'NONE', *, *, #17651, .T. ) ;
#34545=CARTESIAN_POINT ( 'NONE',  ( 1.040000000000001812, -34.41385771548413430, -0.2702793785573777696 ) ) ;
#34548=FACE_OUTER_BOUND ( 'NONE', #22128, .T. ) ;
#34549=VECTOR ( 'NONE', #19139, 1000.000000000000000 ) ;
#34551=SHAPE_REPRESENTATION_RELATIONSHIP ( 'NONE' , 'NONE' ,  #1195, #17803 ) ;
#34552=B_SPLINE_CURVE_WITH_KNOTS ( 'NONE', 3,
 ( #29291, #2228, #24107, #32123, #14776, #14947 ),
 .UNSPECIFIED., .F., .F.,
 ( 4, 2, 4 ),
 ( 4.404817104804532277E-07, 0.001874269682437030085, 0.003748098883163587889 ),
 .UNSPECIFIED. ) ;
#34562=EDGE_LOOP ( 'NONE', ( #12605, #25051, #4187, #33020 ) ) ;
#34563=EDGE_LOOP ( 'NONE', ( #7642, #31657, #15723, #22802, #24108, #3189, #1638, #11823 ) ) ;
#34565=CARTESIAN_POINT ( 'NONE',  ( 2.765921099433442443, 20.99477179376825120, 22.93149026599753526 ) ) ;
#34568=ORIENTED_EDGE ( 'NONE', *, *, #13776, .F. ) ;
#34572=ORIENTED_EDGE ( 'NONE', *, *, #9390, .T. ) ;
#34575=DIRECTION ( 'NONE',  ( -1.000000000000000000, 0.000000000000000000, 0.000000000000000000 ) ) ;
#34587=CYLINDRICAL_SURFACE ( 'NONE', #5847, 2.524999999999999467 ) ;
#34596=VERTEX_POINT ( 'NONE', #11765 ) ;
#34598=CARTESIAN_POINT ( 'NONE',  ( 2.789999999999999147, -5.984944020946091570, 31.37417528048439763 ) ) ;
#34623=ORIENTED_EDGE ( 'NONE', *, *, #968, .T. ) ;
#34626=CARTESIAN_POINT ( 'NONE',  ( 0.07098932002541190334, -18.14847849655012624, -25.98417794693637362 ) ) ;
#34639=LINE ( 'NONE', #12416, #29035 ) ;
#34651=VERTEX_POINT ( 'NONE', #6391 ) ;
#34655=VECTOR ( 'NONE', #8816, 1000.000000000000000 ) ;
#34656=DIRECTION ( 'NONE',  ( -1.000000000000000000, -0.000000000000000000, -0.000000000000000000 ) ) ;
#34658=CARTESIAN_POINT ( 'NONE',  ( 0.02407890056655781832, 31.00221527374952046, -2.344426712874310148 ) ) ;
#34660=VERTEX_POINT ( 'NONE', #17472 ) ;
#34672=DIRECTION ( 'NONE',  ( 1.000000000000000000, -0.000000000000000000, 0.000000000000000000 ) ) ;
#34678=CARTESIAN_POINT ( 'NONE',  ( -8.455559046012042135E-14, 30.58763704338517897, -2.144802104989565361 ) ) ;
#34698=DIRECTION ( 'NONE',  ( 1.000000000000000000, 0.000000000000000000, -0.000000000000000000 ) ) ;
#34702=VERTEX_POINT ( 'NONE', #14787 ) ;
#34706=EDGE_LOOP ( 'NONE', ( #7291, #34994, #30354, #31081, #11832, #34096 ) ) ;
#34707=EDGE_CURVE ( 'NONE', #22622, #8559, #2936, .T. ) ;
#34722=DIRECTION ( 'NONE',  ( 0.000000000000000000, -0.9822872507286879440, -0.1873813145857282925 ) ) ;
#34724=CARTESIAN_POINT ( 'NONE',  ( 0.02407890056441847060, -0.3931553186915530129, 31.08824725498900321 ) ) ;
#34726=CARTESIAN_POINT ( 'NONE',  ( 2.789999999999999147, 17.98401995359667893, -24.59729088254936613 ) ) ;
#34748=CARTESIAN_POINT ( 'NONE',  ( 0.000000000000000000, 7.489092610871481703, -29.53582882395380693 ) ) ;
#34752=CARTESIAN_POINT ( 'NONE',  ( 0.000000000000000000, -23.41952779159748843, -19.49300927180572529 ) ) ;
#34761=DIRECTION ( 'NONE',  ( 0.000000000000000000, 0.000000000000000000, 1.000000000000000000 ) ) ;
#34776=CARTESIAN_POINT ( 'NONE',  ( 1.039999999999999147, -33.39989884085096605, 8.296590337300141726 ) ) ;
#34779=ORIENTED_EDGE ( 'NONE', *, *, #9542, .T. ) ;
#34788=EDGE_CURVE ( 'NONE', #19079, #26414, #21156, .T. ) ;
#34794=ORIENTED_EDGE ( 'NONE', *, *, #13867, .T. ) ;
#34807=DIRECTION ( 'NONE',  ( 0.000000000000000000, -0.7705132427757861446, -0.6374239897486932982 ) ) ;
#34821=B_SPLINE_CURVE_WITH_KNOTS ( 'NONE', 3,
 ( #25921, #1871, #15422, #34097, #6857, #22902 ),
 .UNSPECIFIED., .F., .F.,
 ( 4, 2, 4 ),
 ( 4.404817002564676105E-07, 0.001874269606309968183, 0.003748098730919679870 ),
 .UNSPECIFIED. ) ;
#34842=ORIENTED_EDGE ( 'NONE', *, *, #3243, .T. ) ;
#34853=AXIS2_PLACEMENT_3D ( 'NONE', #7659, #4808, #27061 ) ;
#34854=DIRECTION ( 'NONE',  ( -1.000000000000000000, -0.000000000000000000, -0.000000000000000000 ) ) ;
#34859=CARTESIAN_POINT ( 'NONE',  ( 0.006871268844553799111, -30.26101440722787217, 6.099076262612395993 ) ) ;
#34862=EDGE_CURVE ( 'NONE', #22788, #2604, #14395, .T. ) ;
#34865=CARTESIAN_POINT ( 'NONE',  ( 2.789999999999999147, 29.94779062842794559, -5.619744560738758388 ) ) ;
#34872=ORIENTED_EDGE ( 'NONE', *, *, #15465, .T. ) ;
#34875=CIRCLE ( 'NONE', #6976, 2.525000000000000799 ) ;
#34878=VERTEX_POINT ( 'NONE', #16533 ) ;
#34881=B_SPLINE_CURVE_WITH_KNOTS ( 'NONE', 3,
 ( #29475, #10426, #13286, #8096 ),
 .UNSPECIFIED., .F., .F.,
 ( 4, 4 ),
 ( 0.005298517298376327969, 0.005985383706685561134 ),
 .UNSPECIFIED. ) ;
#34885=ORIENTED_EDGE ( 'NONE', *, *, #26670, .T. ) ;
#34889=CARTESIAN_POINT ( 'NONE',  ( 2.765921099433443775, -11.07880054387241664, 29.04985141099759360 ) ) ;
#34892=CARTESIAN_POINT ( 'NONE',  ( 0.1859802827496877808, 4.859980099383433227, 31.91379830674626206 ) ) ;
#34896=EDGE_LOOP ( 'NONE', ( #9352, #32315, #4339, #19844, #20272, #10227 ) ) ;
#34902=ORIENTED_EDGE ( 'NONE', *, *, #20295, .F. ) ;
#34911=DIRECTION ( 'NONE',  ( 0.000000000000000000, 0.000000000000000000, 1.000000000000000000 ) ) ;
#34913=VERTEX_POINT ( 'NONE', #25036 ) ;
#34917=ORIENTED_EDGE ( 'NONE', *, *, #18898, .T. ) ;
#34921=VERTEX_POINT ( 'NONE', #11719 ) ;
#34928=DIRECTION ( 'NONE',  ( 0.000000000000000000, 0.000000000000000000, 1.000000000000000000 ) ) ;
#34934=CARTESIAN_POINT ( 'NONE',  ( 0.006871323915374539550, 4.186936631162940792, 30.58426604563496909 ) ) ;
#34936=B_SPLINE_CURVE_WITH_KNOTS ( 'NONE', 3,
 ( #7614, #21154, #17804, #34505 ),
 .UNSPECIFIED., .F., .F.,
 ( 4, 4 ),
 ( 0.005298458409503519449, 0.005985325590332028593 ),
 .UNSPECIFIED. ) ;
#34939=CARTESIAN_POINT ( 'NONE',  ( 1.749999999999999778, -33.39989884085096605, 8.296590337300138174 ) ) ;
#34940=ORIENTED_EDGE ( 'NONE', *, *, #34862, .T. ) ;
#34952=ORIENTED_EDGE ( 'NONE', *, *, #15125, .T. ) ;
#34958=CARTESIAN_POINT ( 'NONE',  ( -8.256681647508496812E-14, -11.08290750743005226, 28.58973358960017919 ) ) ;
#34967=DIRECTION ( 'NONE',  ( -1.000000000000000000, -0.000000000000000000, -0.000000000000000000 ) ) ;
#34969=ADVANCED_FACE ( 'NONE', ( #5472 ), #27892, .T. ) ;
#34971=VECTOR ( 'NONE', #20156, 1000.000000000000000 ) ;
#34980=CARTESIAN_POINT ( 'NONE',  ( 0.000000000000000000, 0.000000000000000000, 0.000000000000000000 ) ) ;
#34987=CARTESIAN_POINT ( 'NONE',  ( 0.000000000000000000, 23.28319895603578971, 21.86437915510226659 ) ) ;
#34992=ORIENTED_EDGE ( 'NONE', *, *, #31149, .T. ) ;
#34994=ORIENTED_EDGE ( 'NONE', *, *, #4490, .F. ) ;
#34995=CIRCLE ( 'NONE', #2577, 30.47050528711511674 ) ;
#34997=CARTESIAN_POINT ( 'NONE',  ( 2.765921099433442443, 29.44518845714779332, -9.980709654879110104 ) ) ;
#35002=CARTESIAN_POINT ( 'NONE',  ( 2.789999999999999147, -30.41598411195407081, -1.821977758773984490 ) ) ;
#35003=ORIENTED_EDGE ( 'NONE', *, *, #3548, .F. ) ;
#35006=AXIS2_PLACEMENT_3D ( 'NONE', #8226, #29952, #19283 ) ;
#35018=EDGE_CURVE ( 'NONE', #19221, #2759, #33471, .T. ) ;
#35019=ORIENTED_EDGE ( 'NONE', *, *, #24005, .T. ) ;
#35021=ORIENTED_EDGE ( 'NONE', *, *, #11984, .F. ) ;
#35022=ORIENTED_EDGE ( 'NONE', *, *, #33017, .F. ) ;
#35023=DIRECTION ( 'NONE',  ( 0.000000000000000000, 0.000000000000000000, 1.000000000000000000 ) ) ;
#35027=DIRECTION ( 'NONE',  ( -1.000000000000000000, 0.000000000000000000, 0.000000000000000000 ) ) ;
#35031=ORIENTED_EDGE ( 'NONE', *, *, #21992, .T. ) ;
#35034=CYLINDRICAL_SURFACE ( 'NONE', #102, 16.19999999999999574 ) ;
#35036=CARTESIAN_POINT ( 'NONE',  ( 2.261199741286049836, 30.75271593550620608, -13.00575455800169955 ) ) ;
#35056=CARTESIAN_POINT ( 'NONE',  ( 0.02407890056655738464, 24.20451283648857554, -19.51346322004903300 ) ) ;
#35057=LINE ( 'NONE', #13681, #13564 ) ;
#35058=CARTESIAN_POINT ( 'NONE',  ( 5.917509466954039044E-05, -25.81864426690146885, -16.24881338200996694 ) ) ;
#35073=CARTESIAN_POINT ( 'NONE',  ( 0.000000000000000000, 7.489092610871481703, -29.53582882395380693 ) ) ;
#35076=CARTESIAN_POINT ( 'NONE',  ( 1.749999999999999778, 0.000000000000000000, 0.000000000000000000 ) ) ;
#35078=ORIENTED_EDGE ( 'NONE', *, *, #31078, .T. ) ;
#35085=CARTESIAN_POINT ( 'NONE',  ( 1.394999999999999574, 14.40815186467820475, -31.25366880301303496 ) ) ;
#35087=DIRECTION ( 'NONE',  ( -1.000000000000000000, 0.000000000000000000, 0.000000000000000000 ) ) ;
#35088=AXIS2_PLACEMENT_3D ( 'NONE', #18271, #29635, #18793 ) ;
#35092=CARTESIAN_POINT ( 'NONE',  ( 2.789999999999999147, 30.40449935640660684, 2.004522720844263084 ) ) ;
#35283=COLOUR_RGB('Off White',0.89,0.88,0.83);
#35284=FILL_AREA_STYLE_COLOUR('',#35283);
#35285=FILL_AREA_STYLE('',(#35284));
#35286=SURFACE_STYLE_FILL_AREA(#35285);
#35287=SURFACE_SIDE_STYLE('',(#35286));
#35288=SURFACE_STYLE_USAGE(.BOTH.,#35287);
#35289=PRESENTATION_STYLE_ASSIGNMENT((#35288));
ENDSEC;
END-ISO-10303-21;
